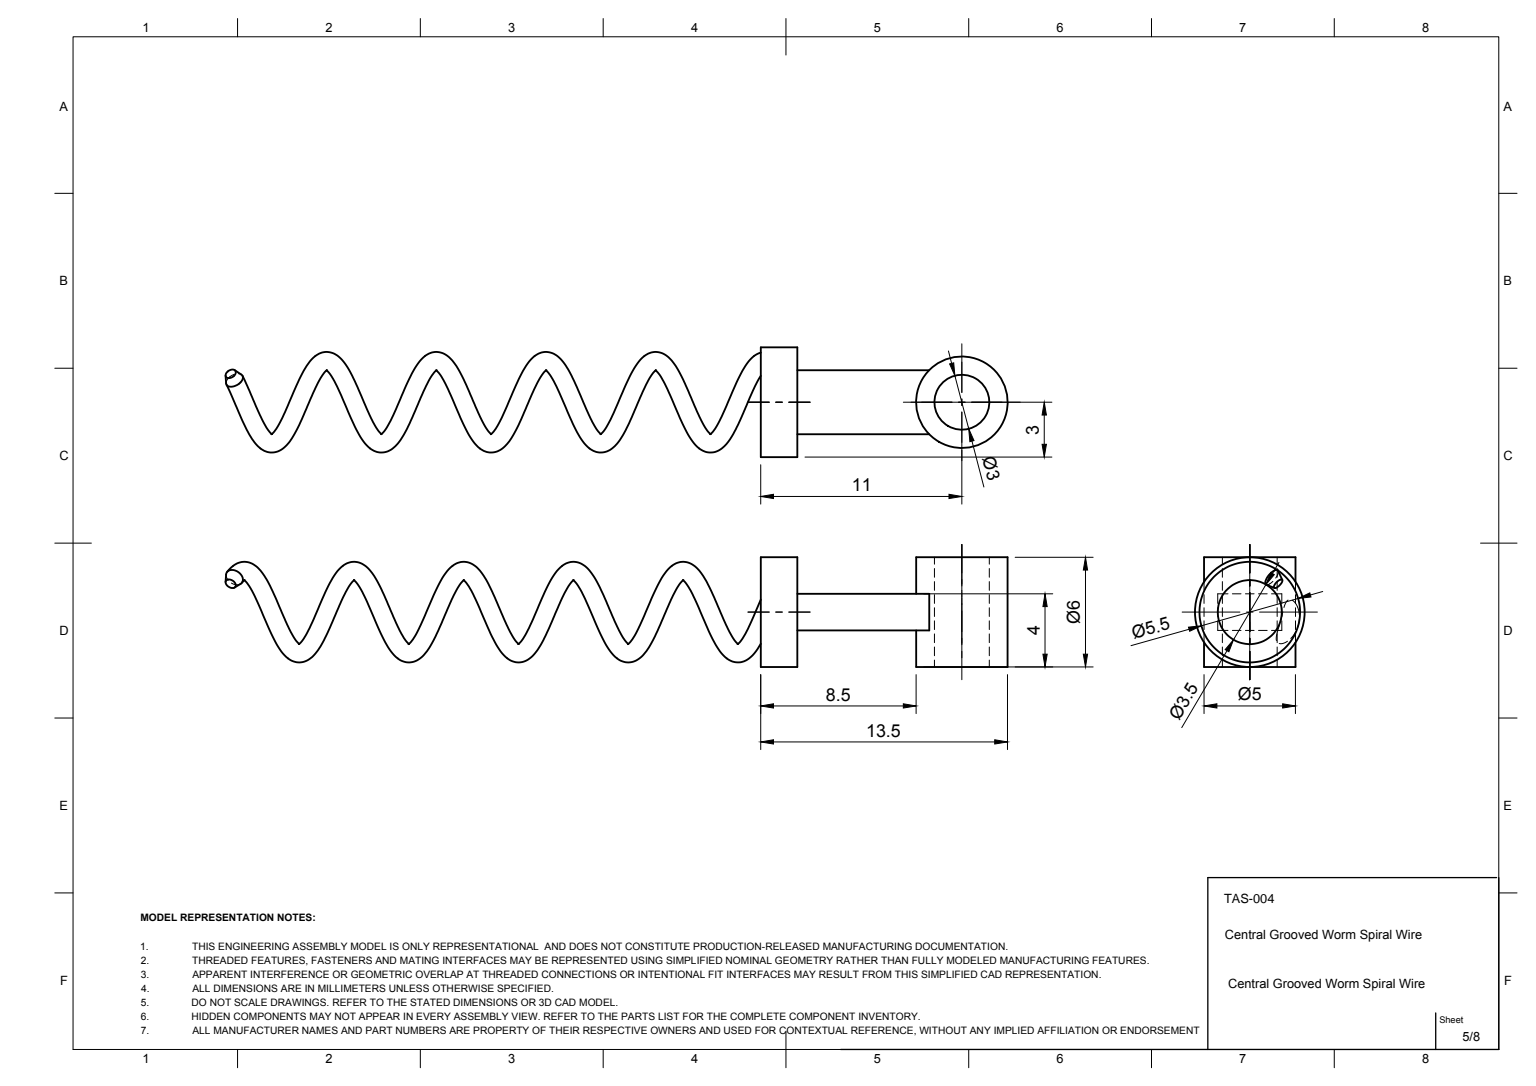
ISO-10303-21;
HEADER;
/* Generated by software containing ST-Developer
 * from STEP Tools, Inc. (www.steptools.com) 
 */

FILE_DESCRIPTION(
/* description */ ('STEP AP214'),
/* implementation_level */ '2;1');

FILE_NAME(
/* name */ 'Central Grooved Worm Spiral Wire.step',
/* time_stamp */ '2026-11-04T19:48:07-08:00',
/* author */ (''),
/* organization */ (''),
/* preprocessor_version */ 'ST-DEVELOPER v20.2',
/* originating_system */ 'Autodesk Translation Framework v15.17.0.0',
/* authorisation */ '');

FILE_SCHEMA (('AUTOMOTIVE_DESIGN { 1 0 10303 214 3 1 1 }'));
ENDSEC;

DATA;
#10=MECHANICAL_DESIGN_GEOMETRIC_PRESENTATION_REPRESENTATION('',(#61),#9561);
#35=(
BOUNDED_SURFACE()
B_SPLINE_SURFACE(3,2,((#4268,#4269,#4270,#4271,#4272,#4273,#4274,#4275,
#4276,#4277,#4278,#4279,#4280,#4281,#4282,#4283,#4284,#4285,#4286,#4287,
#4288,#4289,#4290,#4291,#4292,#4293,#4294,#4295,#4296,#4297,#4298,#4299,
#4300,#4301,#4302,#4303,#4304,#4305,#4306,#4307,#4308,#4309,#4310,#4311,
#4312,#4313,#4314,#4315,#4316,#4317,#4318,#4319,#4320,#4321,#4322,#4323,
#4324,#4325,#4326,#4327,#4328,#4329,#4330,#4331,#4332,#4333,#4334,#4335,
#4336,#4337,#4338,#4339,#4340,#4341,#4342,#4343,#4344,#4345,#4346,#4347,
#4348,#4349,#4350,#4351,#4352,#4353,#4354,#4355,#4356,#4357,#4358,#4359,
#4360,#4361,#4362,#4363,#4364,#4365,#4366,#4367,#4368,#4369,#4370,#4371,
#4372,#4373,#4374,#4375,#4376,#4377,#4378,#4379,#4380,#4381,#4382,#4383,
#4384,#4385,#4386,#4387,#4388,#4389,#4390,#4391,#4392,#4393,#4394,#4395,
#4396,#4397,#4398,#4399,#4400,#4401,#4402,#4403,#4404,#4405,#4406,#4407,
#4408),(#4409,#4410,#4411,#4412,#4413,#4414,#4415,#4416,#4417,#4418,#4419,
#4420,#4421,#4422,#4423,#4424,#4425,#4426,#4427,#4428,#4429,#4430,#4431,
#4432,#4433,#4434,#4435,#4436,#4437,#4438,#4439,#4440,#4441,#4442,#4443,
#4444,#4445,#4446,#4447,#4448,#4449,#4450,#4451,#4452,#4453,#4454,#4455,
#4456,#4457,#4458,#4459,#4460,#4461,#4462,#4463,#4464,#4465,#4466,#4467,
#4468,#4469,#4470,#4471,#4472,#4473,#4474,#4475,#4476,#4477,#4478,#4479,
#4480,#4481,#4482,#4483,#4484,#4485,#4486,#4487,#4488,#4489,#4490,#4491,
#4492,#4493,#4494,#4495,#4496,#4497,#4498,#4499,#4500,#4501,#4502,#4503,
#4504,#4505,#4506,#4507,#4508,#4509,#4510,#4511,#4512,#4513,#4514,#4515,
#4516,#4517,#4518,#4519,#4520,#4521,#4522,#4523,#4524,#4525,#4526,#4527,
#4528,#4529,#4530,#4531,#4532,#4533,#4534,#4535,#4536,#4537,#4538,#4539,
#4540,#4541,#4542,#4543,#4544,#4545,#4546,#4547,#4548,#4549),(#4550,#4551,
#4552,#4553,#4554,#4555,#4556,#4557,#4558,#4559,#4560,#4561,#4562,#4563,
#4564,#4565,#4566,#4567,#4568,#4569,#4570,#4571,#4572,#4573,#4574,#4575,
#4576,#4577,#4578,#4579,#4580,#4581,#4582,#4583,#4584,#4585,#4586,#4587,
#4588,#4589,#4590,#4591,#4592,#4593,#4594,#4595,#4596,#4597,#4598,#4599,
#4600,#4601,#4602,#4603,#4604,#4605,#4606,#4607,#4608,#4609,#4610,#4611,
#4612,#4613,#4614,#4615,#4616,#4617,#4618,#4619,#4620,#4621,#4622,#4623,
#4624,#4625,#4626,#4627,#4628,#4629,#4630,#4631,#4632,#4633,#4634,#4635,
#4636,#4637,#4638,#4639,#4640,#4641,#4642,#4643,#4644,#4645,#4646,#4647,
#4648,#4649,#4650,#4651,#4652,#4653,#4654,#4655,#4656,#4657,#4658,#4659,
#4660,#4661,#4662,#4663,#4664,#4665,#4666,#4667,#4668,#4669,#4670,#4671,
#4672,#4673,#4674,#4675,#4676,#4677,#4678,#4679,#4680,#4681,#4682,#4683,
#4684,#4685,#4686,#4687,#4688,#4689,#4690),(#4691,#4692,#4693,#4694,#4695,
#4696,#4697,#4698,#4699,#4700,#4701,#4702,#4703,#4704,#4705,#4706,#4707,
#4708,#4709,#4710,#4711,#4712,#4713,#4714,#4715,#4716,#4717,#4718,#4719,
#4720,#4721,#4722,#4723,#4724,#4725,#4726,#4727,#4728,#4729,#4730,#4731,
#4732,#4733,#4734,#4735,#4736,#4737,#4738,#4739,#4740,#4741,#4742,#4743,
#4744,#4745,#4746,#4747,#4748,#4749,#4750,#4751,#4752,#4753,#4754,#4755,
#4756,#4757,#4758,#4759,#4760,#4761,#4762,#4763,#4764,#4765,#4766,#4767,
#4768,#4769,#4770,#4771,#4772,#4773,#4774,#4775,#4776,#4777,#4778,#4779,
#4780,#4781,#4782,#4783,#4784,#4785,#4786,#4787,#4788,#4789,#4790,#4791,
#4792,#4793,#4794,#4795,#4796,#4797,#4798,#4799,#4800,#4801,#4802,#4803,
#4804,#4805,#4806,#4807,#4808,#4809,#4810,#4811,#4812,#4813,#4814,#4815,
#4816,#4817,#4818,#4819,#4820,#4821,#4822,#4823,#4824,#4825,#4826,#4827,
#4828,#4829,#4830,#4831),(#4832,#4833,#4834,#4835,#4836,#4837,#4838,#4839,
#4840,#4841,#4842,#4843,#4844,#4845,#4846,#4847,#4848,#4849,#4850,#4851,
#4852,#4853,#4854,#4855,#4856,#4857,#4858,#4859,#4860,#4861,#4862,#4863,
#4864,#4865,#4866,#4867,#4868,#4869,#4870,#4871,#4872,#4873,#4874,#4875,
#4876,#4877,#4878,#4879,#4880,#4881,#4882,#4883,#4884,#4885,#4886,#4887,
#4888,#4889,#4890,#4891,#4892,#4893,#4894,#4895,#4896,#4897,#4898,#4899,
#4900,#4901,#4902,#4903,#4904,#4905,#4906,#4907,#4908,#4909,#4910,#4911,
#4912,#4913,#4914,#4915,#4916,#4917,#4918,#4919,#4920,#4921,#4922,#4923,
#4924,#4925,#4926,#4927,#4928,#4929,#4930,#4931,#4932,#4933,#4934,#4935,
#4936,#4937,#4938,#4939,#4940,#4941,#4942,#4943,#4944,#4945,#4946,#4947,
#4948,#4949,#4950,#4951,#4952,#4953,#4954,#4955,#4956,#4957,#4958,#4959,
#4960,#4961,#4962,#4963,#4964,#4965,#4966,#4967,#4968,#4969,#4970,#4971,
#4972),(#4973,#4974,#4975,#4976,#4977,#4978,#4979,#4980,#4981,#4982,#4983,
#4984,#4985,#4986,#4987,#4988,#4989,#4990,#4991,#4992,#4993,#4994,#4995,
#4996,#4997,#4998,#4999,#5000,#5001,#5002,#5003,#5004,#5005,#5006,#5007,
#5008,#5009,#5010,#5011,#5012,#5013,#5014,#5015,#5016,#5017,#5018,#5019,
#5020,#5021,#5022,#5023,#5024,#5025,#5026,#5027,#5028,#5029,#5030,#5031,
#5032,#5033,#5034,#5035,#5036,#5037,#5038,#5039,#5040,#5041,#5042,#5043,
#5044,#5045,#5046,#5047,#5048,#5049,#5050,#5051,#5052,#5053,#5054,#5055,
#5056,#5057,#5058,#5059,#5060,#5061,#5062,#5063,#5064,#5065,#5066,#5067,
#5068,#5069,#5070,#5071,#5072,#5073,#5074,#5075,#5076,#5077,#5078,#5079,
#5080,#5081,#5082,#5083,#5084,#5085,#5086,#5087,#5088,#5089,#5090,#5091,
#5092,#5093,#5094,#5095,#5096,#5097,#5098,#5099,#5100,#5101,#5102,#5103,
#5104,#5105,#5106,#5107,#5108,#5109,#5110,#5111,#5112,#5113),(#5114,#5115,
#5116,#5117,#5118,#5119,#5120,#5121,#5122,#5123,#5124,#5125,#5126,#5127,
#5128,#5129,#5130,#5131,#5132,#5133,#5134,#5135,#5136,#5137,#5138,#5139,
#5140,#5141,#5142,#5143,#5144,#5145,#5146,#5147,#5148,#5149,#5150,#5151,
#5152,#5153,#5154,#5155,#5156,#5157,#5158,#5159,#5160,#5161,#5162,#5163,
#5164,#5165,#5166,#5167,#5168,#5169,#5170,#5171,#5172,#5173,#5174,#5175,
#5176,#5177,#5178,#5179,#5180,#5181,#5182,#5183,#5184,#5185,#5186,#5187,
#5188,#5189,#5190,#5191,#5192,#5193,#5194,#5195,#5196,#5197,#5198,#5199,
#5200,#5201,#5202,#5203,#5204,#5205,#5206,#5207,#5208,#5209,#5210,#5211,
#5212,#5213,#5214,#5215,#5216,#5217,#5218,#5219,#5220,#5221,#5222,#5223,
#5224,#5225,#5226,#5227,#5228,#5229,#5230,#5231,#5232,#5233,#5234,#5235,
#5236,#5237,#5238,#5239,#5240,#5241,#5242,#5243,#5244,#5245,#5246,#5247,
#5248,#5249,#5250,#5251,#5252,#5253,#5254)),.UNSPECIFIED.,.T.,.F.,.F.)
B_SPLINE_SURFACE_WITH_KNOTS((4,3,4),(3,2,2,2,2,2,2,2,2,2,2,2,2,2,2,2,2,
2,2,2,2,2,2,2,2,2,2,2,2,2,2,2,2,2,2,2,2,2,2,2,2,2,2,2,2,2,2,2,2,2,2,2,2,
2,2,2,2,2,2,2,2,2,2,2,2,2,2,2,2,2,3),(0.,0.5,1.),(0.,0.0142857142857143,
0.0285714285714286,0.0428571428571429,0.0571428571428571,0.0714285714285714,
0.0857142857142857,0.1,0.114285714285714,0.128571428571429,0.142857142857143,
0.157142857142857,0.171428571428571,0.185714285714286,0.2,0.214285714285714,
0.228571428571429,0.242857142857143,0.257142857142857,0.271428571428571,
0.285714285714286,0.3,0.314285714285714,0.328571428571429,0.342857142857143,
0.357142857142857,0.371428571428571,0.385714285714286,0.4,0.414285714285714,
0.428571428571429,0.442857142857143,0.457142857142857,0.471428571428571,
0.485714285714286,0.5,0.514285714285714,0.528571428571429,0.542857142857143,
0.557142857142857,0.571428571428571,0.585714285714286,0.6,0.614285714285714,
0.628571428571429,0.642857142857143,0.657142857142857,0.671428571428571,
0.685714285714286,0.7,0.714285714285714,0.728571428571429,0.742857142857143,
0.757142857142857,0.771428571428571,0.785714285714286,0.8,0.814285714285714,
0.828571428571429,0.842857142857143,0.857142857142857,0.871428571428571,
0.885714285714286,0.9,0.914285714285714,0.928571428571429,0.942857142857143,
0.957142857142857,0.971428571428571,0.985714285714286,1.),.UNSPECIFIED.)
GEOMETRIC_REPRESENTATION_ITEM()
RATIONAL_B_SPLINE_SURFACE(((1.,0.974927912181824,1.,0.974927912181824,1.,
0.974927912181824,1.,0.974927912181824,1.,0.974927912181824,1.,0.974927912181824,
1.,0.974927912181824,1.,0.974927912181824,1.,0.974927912181824,1.,0.974927912181824,
1.,0.974927912181824,1.,0.974927912181824,1.,0.974927912181824,1.,0.974927912181824,
1.,0.974927912181824,1.,0.974927912181824,1.,0.974927912181824,1.,0.974927912181824,
1.,0.974927912181824,1.,0.974927912181824,1.,0.974927912181824,1.,0.974927912181824,
1.,0.974927912181824,1.,0.974927912181824,1.,0.974927912181824,1.,0.974927912181824,
1.,0.974927912181824,1.,0.974927912181824,1.,0.974927912181824,1.,0.974927912181824,
1.,0.974927912181824,1.,0.974927912181824,1.,0.974927912181824,1.,0.974927912181824,
1.,0.974927912181824,1.,0.974927912181824,1.,0.974927912181824,1.,0.974927912181824,
1.,0.974927912181824,1.,0.974927912181824,1.,0.974927912181824,1.,0.974927912181824,
1.,0.974927912181824,1.,0.974927912181824,1.,0.974927912181824,1.,0.974927912181824,
1.,0.974927912181824,1.,0.974927912181824,1.,0.974927912181824,1.,0.974927912181824,
1.,0.974927912181824,1.,0.974927912181824,1.,0.974927912181824,1.,0.974927912181824,
1.,0.974927912181824,1.,0.974927912181824,1.,0.974927912181824,1.,0.974927912181824,
1.,0.974927912181824,1.,0.974927912181824,1.,0.974927912181824,1.,0.974927912181824,
1.,0.974927912181824,1.,0.974927912181824,1.,0.974927912181824,1.,0.974927912181824,
1.,0.974927912181824,1.,0.974927912181824,1.,0.974927912181824,1.,0.974927912181824,
1.),(0.333333333333333,0.324975970727275,0.333333333333333,0.324975970727275,
0.333333333333333,0.324975970727275,0.333333333333333,0.324975970727275,
0.333333333333333,0.324975970727275,0.333333333333333,0.324975970727275,
0.333333333333333,0.324975970727275,0.333333333333333,0.324975970727275,
0.333333333333333,0.324975970727275,0.333333333333333,0.324975970727275,
0.333333333333333,0.324975970727275,0.333333333333333,0.324975970727275,
0.333333333333333,0.324975970727275,0.333333333333333,0.324975970727275,
0.333333333333333,0.324975970727275,0.333333333333333,0.324975970727275,
0.333333333333333,0.324975970727275,0.333333333333333,0.324975970727275,
0.333333333333333,0.324975970727275,0.333333333333333,0.324975970727275,
0.333333333333333,0.324975970727275,0.333333333333333,0.324975970727275,
0.333333333333333,0.324975970727275,0.333333333333333,0.324975970727275,
0.333333333333333,0.324975970727275,0.333333333333333,0.324975970727275,
0.333333333333333,0.324975970727275,0.333333333333333,0.324975970727275,
0.333333333333333,0.324975970727275,0.333333333333333,0.324975970727275,
0.333333333333333,0.324975970727275,0.333333333333333,0.324975970727275,
0.333333333333333,0.324975970727275,0.333333333333333,0.324975970727275,
0.333333333333333,0.324975970727275,0.333333333333333,0.324975970727275,
0.333333333333333,0.324975970727275,0.333333333333333,0.324975970727275,
0.333333333333333,0.324975970727275,0.333333333333333,0.324975970727275,
0.333333333333333,0.324975970727275,0.333333333333333,0.324975970727275,
0.333333333333333,0.324975970727275,0.333333333333333,0.324975970727275,
0.333333333333333,0.324975970727275,0.333333333333333,0.324975970727275,
0.333333333333333,0.324975970727275,0.333333333333333,0.324975970727275,
0.333333333333333,0.324975970727275,0.333333333333333,0.324975970727275,
0.333333333333333,0.324975970727275,0.333333333333333,0.324975970727275,
0.333333333333333,0.324975970727275,0.333333333333333,0.324975970727275,
0.333333333333333,0.324975970727275,0.333333333333333,0.324975970727275,
0.333333333333333,0.324975970727275,0.333333333333333,0.324975970727275,
0.333333333333333,0.324975970727275,0.333333333333333,0.324975970727275,
0.333333333333333,0.324975970727275,0.333333333333333,0.324975970727275,
0.333333333333333,0.324975970727275,0.333333333333333,0.324975970727275,
0.333333333333333,0.324975970727275,0.333333333333333,0.324975970727275,
0.333333333333333,0.324975970727275,0.333333333333333,0.324975970727275,
0.333333333333333,0.324975970727275,0.333333333333333,0.324975970727275,
0.333333333333333),(0.333333333333333,0.324975970727275,0.333333333333333,
0.324975970727275,0.333333333333333,0.324975970727275,0.333333333333333,
0.324975970727275,0.333333333333333,0.324975970727275,0.333333333333333,
0.324975970727275,0.333333333333333,0.324975970727275,0.333333333333333,
0.324975970727275,0.333333333333333,0.324975970727275,0.333333333333333,
0.324975970727275,0.333333333333333,0.324975970727275,0.333333333333333,
0.324975970727275,0.333333333333333,0.324975970727275,0.333333333333333,
0.324975970727275,0.333333333333333,0.324975970727275,0.333333333333333,
0.324975970727275,0.333333333333333,0.324975970727275,0.333333333333333,
0.324975970727275,0.333333333333333,0.324975970727275,0.333333333333333,
0.324975970727275,0.333333333333333,0.324975970727275,0.333333333333333,
0.324975970727275,0.333333333333333,0.324975970727275,0.333333333333333,
0.324975970727275,0.333333333333333,0.324975970727275,0.333333333333333,
0.324975970727275,0.333333333333333,0.324975970727275,0.333333333333333,
0.324975970727275,0.333333333333333,0.324975970727275,0.333333333333333,
0.324975970727275,0.333333333333333,0.324975970727275,0.333333333333333,
0.324975970727275,0.333333333333333,0.324975970727275,0.333333333333333,
0.324975970727275,0.333333333333333,0.324975970727275,0.333333333333333,
0.324975970727275,0.333333333333333,0.324975970727275,0.333333333333333,
0.324975970727275,0.333333333333333,0.324975970727275,0.333333333333333,
0.324975970727275,0.333333333333333,0.324975970727275,0.333333333333333,
0.324975970727275,0.333333333333333,0.324975970727275,0.333333333333333,
0.324975970727275,0.333333333333333,0.324975970727275,0.333333333333333,
0.324975970727275,0.333333333333333,0.324975970727275,0.333333333333333,
0.324975970727275,0.333333333333333,0.324975970727275,0.333333333333333,
0.324975970727275,0.333333333333333,0.324975970727275,0.333333333333333,
0.324975970727275,0.333333333333333,0.324975970727275,0.333333333333333,
0.324975970727275,0.333333333333333,0.324975970727275,0.333333333333333,
0.324975970727275,0.333333333333333,0.324975970727275,0.333333333333333,
0.324975970727275,0.333333333333333,0.324975970727275,0.333333333333333,
0.324975970727275,0.333333333333333,0.324975970727275,0.333333333333333,
0.324975970727275,0.333333333333333,0.324975970727275,0.333333333333333,
0.324975970727275,0.333333333333333,0.324975970727275,0.333333333333333,
0.324975970727275,0.333333333333333,0.324975970727275,0.333333333333333,
0.324975970727275,0.333333333333333,0.324975970727275,0.333333333333333,
0.324975970727275,0.333333333333333),(1.,0.974927912181824,1.,0.974927912181824,
1.,0.974927912181824,1.,0.974927912181824,1.,0.974927912181824,1.,0.974927912181824,
1.,0.974927912181824,1.,0.974927912181824,1.,0.974927912181824,1.,0.974927912181824,
1.,0.974927912181824,1.,0.974927912181824,1.,0.974927912181824,1.,0.974927912181824,
1.,0.974927912181824,1.,0.974927912181824,1.,0.974927912181824,1.,0.974927912181824,
1.,0.974927912181824,1.,0.974927912181824,1.,0.974927912181824,1.,0.974927912181824,
1.,0.974927912181824,1.,0.974927912181824,1.,0.974927912181824,1.,0.974927912181824,
1.,0.974927912181824,1.,0.974927912181824,1.,0.974927912181824,1.,0.974927912181824,
1.,0.974927912181824,1.,0.974927912181824,1.,0.974927912181824,1.,0.974927912181824,
1.,0.974927912181824,1.,0.974927912181824,1.,0.974927912181824,1.,0.974927912181824,
1.,0.974927912181824,1.,0.974927912181824,1.,0.974927912181824,1.,0.974927912181824,
1.,0.974927912181824,1.,0.974927912181824,1.,0.974927912181824,1.,0.974927912181824,
1.,0.974927912181824,1.,0.974927912181824,1.,0.974927912181824,1.,0.974927912181824,
1.,0.974927912181824,1.,0.974927912181824,1.,0.974927912181824,1.,0.974927912181824,
1.,0.974927912181824,1.,0.974927912181824,1.,0.974927912181824,1.,0.974927912181824,
1.,0.974927912181824,1.,0.974927912181824,1.,0.974927912181824,1.,0.974927912181824,
1.,0.974927912181824,1.,0.974927912181824,1.,0.974927912181824,1.,0.974927912181824,
1.,0.974927912181824,1.,0.974927912181824,1.,0.974927912181824,1.,0.974927912181824,
1.),(0.333333333333333,0.324975970727275,0.333333333333333,0.324975970727275,
0.333333333333333,0.324975970727275,0.333333333333333,0.324975970727275,
0.333333333333333,0.324975970727275,0.333333333333333,0.324975970727275,
0.333333333333333,0.324975970727275,0.333333333333333,0.324975970727275,
0.333333333333333,0.324975970727275,0.333333333333333,0.324975970727275,
0.333333333333333,0.324975970727275,0.333333333333333,0.324975970727275,
0.333333333333333,0.324975970727275,0.333333333333333,0.324975970727275,
0.333333333333333,0.324975970727275,0.333333333333333,0.324975970727275,
0.333333333333333,0.324975970727275,0.333333333333333,0.324975970727275,
0.333333333333333,0.324975970727275,0.333333333333333,0.324975970727275,
0.333333333333333,0.324975970727275,0.333333333333333,0.324975970727275,
0.333333333333333,0.324975970727275,0.333333333333333,0.324975970727275,
0.333333333333333,0.324975970727275,0.333333333333333,0.324975970727275,
0.333333333333333,0.324975970727275,0.333333333333333,0.324975970727275,
0.333333333333333,0.324975970727275,0.333333333333333,0.324975970727275,
0.333333333333333,0.324975970727275,0.333333333333333,0.324975970727275,
0.333333333333333,0.324975970727275,0.333333333333333,0.324975970727275,
0.333333333333333,0.324975970727275,0.333333333333333,0.324975970727275,
0.333333333333333,0.324975970727275,0.333333333333333,0.324975970727275,
0.333333333333333,0.324975970727275,0.333333333333333,0.324975970727275,
0.333333333333333,0.324975970727275,0.333333333333333,0.324975970727275,
0.333333333333333,0.324975970727275,0.333333333333333,0.324975970727275,
0.333333333333333,0.324975970727275,0.333333333333333,0.324975970727275,
0.333333333333333,0.324975970727275,0.333333333333333,0.324975970727275,
0.333333333333333,0.324975970727275,0.333333333333333,0.324975970727275,
0.333333333333333,0.324975970727275,0.333333333333333,0.324975970727275,
0.333333333333333,0.324975970727275,0.333333333333333,0.324975970727275,
0.333333333333333,0.324975970727275,0.333333333333333,0.324975970727275,
0.333333333333333,0.324975970727275,0.333333333333333,0.324975970727275,
0.333333333333333,0.324975970727275,0.333333333333333,0.324975970727275,
0.333333333333333,0.324975970727275,0.333333333333333,0.324975970727275,
0.333333333333333,0.324975970727275,0.333333333333333,0.324975970727275,
0.333333333333333,0.324975970727275,0.333333333333333,0.324975970727275,
0.333333333333333,0.324975970727275,0.333333333333333,0.324975970727275,
0.333333333333333,0.324975970727275,0.333333333333333,0.324975970727275,
0.333333333333333),(0.333333333333333,0.324975970727275,0.333333333333333,
0.324975970727275,0.333333333333333,0.324975970727275,0.333333333333333,
0.324975970727275,0.333333333333333,0.324975970727275,0.333333333333333,
0.324975970727275,0.333333333333333,0.324975970727275,0.333333333333333,
0.324975970727275,0.333333333333333,0.324975970727275,0.333333333333333,
0.324975970727275,0.333333333333333,0.324975970727275,0.333333333333333,
0.324975970727275,0.333333333333333,0.324975970727275,0.333333333333333,
0.324975970727275,0.333333333333333,0.324975970727275,0.333333333333333,
0.324975970727275,0.333333333333333,0.324975970727275,0.333333333333333,
0.324975970727275,0.333333333333333,0.324975970727275,0.333333333333333,
0.324975970727275,0.333333333333333,0.324975970727275,0.333333333333333,
0.324975970727275,0.333333333333333,0.324975970727275,0.333333333333333,
0.324975970727275,0.333333333333333,0.324975970727275,0.333333333333333,
0.324975970727275,0.333333333333333,0.324975970727275,0.333333333333333,
0.324975970727275,0.333333333333333,0.324975970727275,0.333333333333333,
0.324975970727275,0.333333333333333,0.324975970727275,0.333333333333333,
0.324975970727275,0.333333333333333,0.324975970727275,0.333333333333333,
0.324975970727275,0.333333333333333,0.324975970727275,0.333333333333333,
0.324975970727275,0.333333333333333,0.324975970727275,0.333333333333333,
0.324975970727275,0.333333333333333,0.324975970727275,0.333333333333333,
0.324975970727275,0.333333333333333,0.324975970727275,0.333333333333333,
0.324975970727275,0.333333333333333,0.324975970727275,0.333333333333333,
0.324975970727275,0.333333333333333,0.324975970727275,0.333333333333333,
0.324975970727275,0.333333333333333,0.324975970727275,0.333333333333333,
0.324975970727275,0.333333333333333,0.324975970727275,0.333333333333333,
0.324975970727275,0.333333333333333,0.324975970727275,0.333333333333333,
0.324975970727275,0.333333333333333,0.324975970727275,0.333333333333333,
0.324975970727275,0.333333333333333,0.324975970727275,0.333333333333333,
0.324975970727275,0.333333333333333,0.324975970727275,0.333333333333333,
0.324975970727275,0.333333333333333,0.324975970727275,0.333333333333333,
0.324975970727275,0.333333333333333,0.324975970727275,0.333333333333333,
0.324975970727275,0.333333333333333,0.324975970727275,0.333333333333333,
0.324975970727275,0.333333333333333,0.324975970727275,0.333333333333333,
0.324975970727275,0.333333333333333,0.324975970727275,0.333333333333333,
0.324975970727275,0.333333333333333,0.324975970727275,0.333333333333333,
0.324975970727275,0.333333333333333),(1.,0.974927912181824,1.,0.974927912181824,
1.,0.974927912181824,1.,0.974927912181824,1.,0.974927912181824,1.,0.974927912181824,
1.,0.974927912181824,1.,0.974927912181824,1.,0.974927912181824,1.,0.974927912181824,
1.,0.974927912181824,1.,0.974927912181824,1.,0.974927912181824,1.,0.974927912181824,
1.,0.974927912181824,1.,0.974927912181824,1.,0.974927912181824,1.,0.974927912181824,
1.,0.974927912181824,1.,0.974927912181824,1.,0.974927912181824,1.,0.974927912181824,
1.,0.974927912181824,1.,0.974927912181824,1.,0.974927912181824,1.,0.974927912181824,
1.,0.974927912181824,1.,0.974927912181824,1.,0.974927912181824,1.,0.974927912181824,
1.,0.974927912181824,1.,0.974927912181824,1.,0.974927912181824,1.,0.974927912181824,
1.,0.974927912181824,1.,0.974927912181824,1.,0.974927912181824,1.,0.974927912181824,
1.,0.974927912181824,1.,0.974927912181824,1.,0.974927912181824,1.,0.974927912181824,
1.,0.974927912181824,1.,0.974927912181824,1.,0.974927912181824,1.,0.974927912181824,
1.,0.974927912181824,1.,0.974927912181824,1.,0.974927912181824,1.,0.974927912181824,
1.,0.974927912181824,1.,0.974927912181824,1.,0.974927912181824,1.,0.974927912181824,
1.,0.974927912181824,1.,0.974927912181824,1.,0.974927912181824,1.,0.974927912181824,
1.,0.974927912181824,1.,0.974927912181824,1.,0.974927912181824,1.,0.974927912181824,
1.,0.974927912181824,1.,0.974927912181824,1.,0.974927912181824,1.,0.974927912181824,
1.,0.974927912181824,1.,0.974927912181824,1.,0.974927912181824,1.,0.974927912181824,
1.)))
REPRESENTATION_ITEM('')
SURFACE()
);
#36=(
BOUNDED_SURFACE()
B_SPLINE_SURFACE(3,2,((#8296,#8297,#8298,#8299,#8300,#8301,#8302,#8303,
#8304,#8305,#8306,#8307,#8308,#8309,#8310,#8311,#8312,#8313,#8314,#8315,
#8316,#8317,#8318,#8319,#8320,#8321,#8322,#8323,#8324,#8325,#8326,#8327,
#8328,#8329,#8330,#8331,#8332,#8333,#8334,#8335,#8336,#8337,#8338,#8339,
#8340,#8341,#8342,#8343,#8344,#8345,#8346,#8347,#8348,#8349,#8350,#8351,
#8352,#8353,#8354,#8355,#8356,#8357,#8358,#8359,#8360,#8361,#8362,#8363,
#8364,#8365,#8366,#8367,#8368,#8369,#8370,#8371,#8372,#8373,#8374,#8375,
#8376,#8377,#8378,#8379,#8380,#8381,#8382,#8383,#8384,#8385,#8386,#8387,
#8388,#8389,#8390,#8391,#8392,#8393,#8394,#8395,#8396,#8397,#8398,#8399,
#8400,#8401,#8402,#8403,#8404,#8405,#8406,#8407,#8408,#8409,#8410,#8411,
#8412,#8413,#8414,#8415,#8416,#8417,#8418,#8419,#8420,#8421,#8422,#8423,
#8424,#8425,#8426,#8427,#8428,#8429,#8430,#8431,#8432,#8433,#8434,#8435,
#8436),(#8437,#8438,#8439,#8440,#8441,#8442,#8443,#8444,#8445,#8446,#8447,
#8448,#8449,#8450,#8451,#8452,#8453,#8454,#8455,#8456,#8457,#8458,#8459,
#8460,#8461,#8462,#8463,#8464,#8465,#8466,#8467,#8468,#8469,#8470,#8471,
#8472,#8473,#8474,#8475,#8476,#8477,#8478,#8479,#8480,#8481,#8482,#8483,
#8484,#8485,#8486,#8487,#8488,#8489,#8490,#8491,#8492,#8493,#8494,#8495,
#8496,#8497,#8498,#8499,#8500,#8501,#8502,#8503,#8504,#8505,#8506,#8507,
#8508,#8509,#8510,#8511,#8512,#8513,#8514,#8515,#8516,#8517,#8518,#8519,
#8520,#8521,#8522,#8523,#8524,#8525,#8526,#8527,#8528,#8529,#8530,#8531,
#8532,#8533,#8534,#8535,#8536,#8537,#8538,#8539,#8540,#8541,#8542,#8543,
#8544,#8545,#8546,#8547,#8548,#8549,#8550,#8551,#8552,#8553,#8554,#8555,
#8556,#8557,#8558,#8559,#8560,#8561,#8562,#8563,#8564,#8565,#8566,#8567,
#8568,#8569,#8570,#8571,#8572,#8573,#8574,#8575,#8576,#8577),(#8578,#8579,
#8580,#8581,#8582,#8583,#8584,#8585,#8586,#8587,#8588,#8589,#8590,#8591,
#8592,#8593,#8594,#8595,#8596,#8597,#8598,#8599,#8600,#8601,#8602,#8603,
#8604,#8605,#8606,#8607,#8608,#8609,#8610,#8611,#8612,#8613,#8614,#8615,
#8616,#8617,#8618,#8619,#8620,#8621,#8622,#8623,#8624,#8625,#8626,#8627,
#8628,#8629,#8630,#8631,#8632,#8633,#8634,#8635,#8636,#8637,#8638,#8639,
#8640,#8641,#8642,#8643,#8644,#8645,#8646,#8647,#8648,#8649,#8650,#8651,
#8652,#8653,#8654,#8655,#8656,#8657,#8658,#8659,#8660,#8661,#8662,#8663,
#8664,#8665,#8666,#8667,#8668,#8669,#8670,#8671,#8672,#8673,#8674,#8675,
#8676,#8677,#8678,#8679,#8680,#8681,#8682,#8683,#8684,#8685,#8686,#8687,
#8688,#8689,#8690,#8691,#8692,#8693,#8694,#8695,#8696,#8697,#8698,#8699,
#8700,#8701,#8702,#8703,#8704,#8705,#8706,#8707,#8708,#8709,#8710,#8711,
#8712,#8713,#8714,#8715,#8716,#8717,#8718),(#8719,#8720,#8721,#8722,#8723,
#8724,#8725,#8726,#8727,#8728,#8729,#8730,#8731,#8732,#8733,#8734,#8735,
#8736,#8737,#8738,#8739,#8740,#8741,#8742,#8743,#8744,#8745,#8746,#8747,
#8748,#8749,#8750,#8751,#8752,#8753,#8754,#8755,#8756,#8757,#8758,#8759,
#8760,#8761,#8762,#8763,#8764,#8765,#8766,#8767,#8768,#8769,#8770,#8771,
#8772,#8773,#8774,#8775,#8776,#8777,#8778,#8779,#8780,#8781,#8782,#8783,
#8784,#8785,#8786,#8787,#8788,#8789,#8790,#8791,#8792,#8793,#8794,#8795,
#8796,#8797,#8798,#8799,#8800,#8801,#8802,#8803,#8804,#8805,#8806,#8807,
#8808,#8809,#8810,#8811,#8812,#8813,#8814,#8815,#8816,#8817,#8818,#8819,
#8820,#8821,#8822,#8823,#8824,#8825,#8826,#8827,#8828,#8829,#8830,#8831,
#8832,#8833,#8834,#8835,#8836,#8837,#8838,#8839,#8840,#8841,#8842,#8843,
#8844,#8845,#8846,#8847,#8848,#8849,#8850,#8851,#8852,#8853,#8854,#8855,
#8856,#8857,#8858,#8859),(#8860,#8861,#8862,#8863,#8864,#8865,#8866,#8867,
#8868,#8869,#8870,#8871,#8872,#8873,#8874,#8875,#8876,#8877,#8878,#8879,
#8880,#8881,#8882,#8883,#8884,#8885,#8886,#8887,#8888,#8889,#8890,#8891,
#8892,#8893,#8894,#8895,#8896,#8897,#8898,#8899,#8900,#8901,#8902,#8903,
#8904,#8905,#8906,#8907,#8908,#8909,#8910,#8911,#8912,#8913,#8914,#8915,
#8916,#8917,#8918,#8919,#8920,#8921,#8922,#8923,#8924,#8925,#8926,#8927,
#8928,#8929,#8930,#8931,#8932,#8933,#8934,#8935,#8936,#8937,#8938,#8939,
#8940,#8941,#8942,#8943,#8944,#8945,#8946,#8947,#8948,#8949,#8950,#8951,
#8952,#8953,#8954,#8955,#8956,#8957,#8958,#8959,#8960,#8961,#8962,#8963,
#8964,#8965,#8966,#8967,#8968,#8969,#8970,#8971,#8972,#8973,#8974,#8975,
#8976,#8977,#8978,#8979,#8980,#8981,#8982,#8983,#8984,#8985,#8986,#8987,
#8988,#8989,#8990,#8991,#8992,#8993,#8994,#8995,#8996,#8997,#8998,#8999,
#9000),(#9001,#9002,#9003,#9004,#9005,#9006,#9007,#9008,#9009,#9010,#9011,
#9012,#9013,#9014,#9015,#9016,#9017,#9018,#9019,#9020,#9021,#9022,#9023,
#9024,#9025,#9026,#9027,#9028,#9029,#9030,#9031,#9032,#9033,#9034,#9035,
#9036,#9037,#9038,#9039,#9040,#9041,#9042,#9043,#9044,#9045,#9046,#9047,
#9048,#9049,#9050,#9051,#9052,#9053,#9054,#9055,#9056,#9057,#9058,#9059,
#9060,#9061,#9062,#9063,#9064,#9065,#9066,#9067,#9068,#9069,#9070,#9071,
#9072,#9073,#9074,#9075,#9076,#9077,#9078,#9079,#9080,#9081,#9082,#9083,
#9084,#9085,#9086,#9087,#9088,#9089,#9090,#9091,#9092,#9093,#9094,#9095,
#9096,#9097,#9098,#9099,#9100,#9101,#9102,#9103,#9104,#9105,#9106,#9107,
#9108,#9109,#9110,#9111,#9112,#9113,#9114,#9115,#9116,#9117,#9118,#9119,
#9120,#9121,#9122,#9123,#9124,#9125,#9126,#9127,#9128,#9129,#9130,#9131,
#9132,#9133,#9134,#9135,#9136,#9137,#9138,#9139,#9140,#9141),(#9142,#9143,
#9144,#9145,#9146,#9147,#9148,#9149,#9150,#9151,#9152,#9153,#9154,#9155,
#9156,#9157,#9158,#9159,#9160,#9161,#9162,#9163,#9164,#9165,#9166,#9167,
#9168,#9169,#9170,#9171,#9172,#9173,#9174,#9175,#9176,#9177,#9178,#9179,
#9180,#9181,#9182,#9183,#9184,#9185,#9186,#9187,#9188,#9189,#9190,#9191,
#9192,#9193,#9194,#9195,#9196,#9197,#9198,#9199,#9200,#9201,#9202,#9203,
#9204,#9205,#9206,#9207,#9208,#9209,#9210,#9211,#9212,#9213,#9214,#9215,
#9216,#9217,#9218,#9219,#9220,#9221,#9222,#9223,#9224,#9225,#9226,#9227,
#9228,#9229,#9230,#9231,#9232,#9233,#9234,#9235,#9236,#9237,#9238,#9239,
#9240,#9241,#9242,#9243,#9244,#9245,#9246,#9247,#9248,#9249,#9250,#9251,
#9252,#9253,#9254,#9255,#9256,#9257,#9258,#9259,#9260,#9261,#9262,#9263,
#9264,#9265,#9266,#9267,#9268,#9269,#9270,#9271,#9272,#9273,#9274,#9275,
#9276,#9277,#9278,#9279,#9280,#9281,#9282)),.UNSPECIFIED.,.T.,.F.,.F.)
B_SPLINE_SURFACE_WITH_KNOTS((4,3,4),(3,2,2,2,2,2,2,2,2,2,2,2,2,2,2,2,2,
2,2,2,2,2,2,2,2,2,2,2,2,2,2,2,2,2,2,2,2,2,2,2,2,2,2,2,2,2,2,2,2,2,2,2,2,
2,2,2,2,2,2,2,2,2,2,2,2,2,2,2,2,2,3),(0.,0.5,1.),(0.,0.0142857142857143,
0.0285714285714286,0.0428571428571429,0.0571428571428571,0.0714285714285714,
0.0857142857142857,0.1,0.114285714285714,0.128571428571429,0.142857142857143,
0.157142857142857,0.171428571428571,0.185714285714286,0.2,0.214285714285714,
0.228571428571429,0.242857142857143,0.257142857142857,0.271428571428571,
0.285714285714286,0.3,0.314285714285714,0.328571428571429,0.342857142857143,
0.357142857142857,0.371428571428571,0.385714285714286,0.4,0.414285714285714,
0.428571428571429,0.442857142857143,0.457142857142857,0.471428571428571,
0.485714285714286,0.5,0.514285714285714,0.528571428571429,0.542857142857143,
0.557142857142857,0.571428571428571,0.585714285714286,0.6,0.614285714285714,
0.628571428571429,0.642857142857143,0.657142857142857,0.671428571428571,
0.685714285714286,0.7,0.714285714285714,0.728571428571429,0.742857142857143,
0.757142857142857,0.771428571428571,0.785714285714286,0.8,0.814285714285714,
0.828571428571429,0.842857142857143,0.857142857142857,0.871428571428571,
0.885714285714286,0.9,0.914285714285714,0.928571428571429,0.942857142857143,
0.957142857142857,0.971428571428571,0.985714285714286,1.),.UNSPECIFIED.)
GEOMETRIC_REPRESENTATION_ITEM()
RATIONAL_B_SPLINE_SURFACE(((1.,0.974927912181824,1.,0.974927912181824,1.,
0.974927912181824,1.,0.974927912181824,1.,0.974927912181824,1.,0.974927912181824,
1.,0.974927912181824,1.,0.974927912181824,1.,0.974927912181824,1.,0.974927912181824,
1.,0.974927912181824,1.,0.974927912181824,1.,0.974927912181824,1.,0.974927912181824,
1.,0.974927912181824,1.,0.974927912181824,1.,0.974927912181824,1.,0.974927912181824,
1.,0.974927912181824,1.,0.974927912181824,1.,0.974927912181824,1.,0.974927912181824,
1.,0.974927912181824,1.,0.974927912181824,1.,0.974927912181824,1.,0.974927912181824,
1.,0.974927912181824,1.,0.974927912181824,1.,0.974927912181824,1.,0.974927912181824,
1.,0.974927912181824,1.,0.974927912181824,1.,0.974927912181824,1.,0.974927912181824,
1.,0.974927912181824,1.,0.974927912181824,1.,0.974927912181824,1.,0.974927912181824,
1.,0.974927912181824,1.,0.974927912181824,1.,0.974927912181824,1.,0.974927912181824,
1.,0.974927912181824,1.,0.974927912181824,1.,0.974927912181824,1.,0.974927912181824,
1.,0.974927912181824,1.,0.974927912181824,1.,0.974927912181824,1.,0.974927912181824,
1.,0.974927912181824,1.,0.974927912181824,1.,0.974927912181824,1.,0.974927912181824,
1.,0.974927912181824,1.,0.974927912181824,1.,0.974927912181824,1.,0.974927912181824,
1.,0.974927912181824,1.,0.974927912181824,1.,0.974927912181824,1.,0.974927912181824,
1.,0.974927912181824,1.,0.974927912181824,1.,0.974927912181824,1.,0.974927912181824,
1.,0.974927912181824,1.,0.974927912181824,1.,0.974927912181824,1.,0.974927912181824,
1.),(0.333333333333333,0.324975970727275,0.333333333333333,0.324975970727275,
0.333333333333333,0.324975970727275,0.333333333333333,0.324975970727275,
0.333333333333333,0.324975970727275,0.333333333333333,0.324975970727275,
0.333333333333333,0.324975970727275,0.333333333333333,0.324975970727275,
0.333333333333333,0.324975970727275,0.333333333333333,0.324975970727275,
0.333333333333333,0.324975970727275,0.333333333333333,0.324975970727275,
0.333333333333333,0.324975970727275,0.333333333333333,0.324975970727275,
0.333333333333333,0.324975970727275,0.333333333333333,0.324975970727275,
0.333333333333333,0.324975970727275,0.333333333333333,0.324975970727275,
0.333333333333333,0.324975970727275,0.333333333333333,0.324975970727275,
0.333333333333333,0.324975970727275,0.333333333333333,0.324975970727275,
0.333333333333333,0.324975970727275,0.333333333333333,0.324975970727275,
0.333333333333333,0.324975970727275,0.333333333333333,0.324975970727275,
0.333333333333333,0.324975970727275,0.333333333333333,0.324975970727275,
0.333333333333333,0.324975970727275,0.333333333333333,0.324975970727275,
0.333333333333333,0.324975970727275,0.333333333333333,0.324975970727275,
0.333333333333333,0.324975970727275,0.333333333333333,0.324975970727275,
0.333333333333333,0.324975970727275,0.333333333333333,0.324975970727275,
0.333333333333333,0.324975970727275,0.333333333333333,0.324975970727275,
0.333333333333333,0.324975970727275,0.333333333333333,0.324975970727275,
0.333333333333333,0.324975970727275,0.333333333333333,0.324975970727275,
0.333333333333333,0.324975970727275,0.333333333333333,0.324975970727275,
0.333333333333333,0.324975970727275,0.333333333333333,0.324975970727275,
0.333333333333333,0.324975970727275,0.333333333333333,0.324975970727275,
0.333333333333333,0.324975970727275,0.333333333333333,0.324975970727275,
0.333333333333333,0.324975970727275,0.333333333333333,0.324975970727275,
0.333333333333333,0.324975970727275,0.333333333333333,0.324975970727275,
0.333333333333333,0.324975970727275,0.333333333333333,0.324975970727275,
0.333333333333333,0.324975970727275,0.333333333333333,0.324975970727275,
0.333333333333333,0.324975970727275,0.333333333333333,0.324975970727275,
0.333333333333333,0.324975970727275,0.333333333333333,0.324975970727275,
0.333333333333333,0.324975970727275,0.333333333333333,0.324975970727275,
0.333333333333333,0.324975970727275,0.333333333333333,0.324975970727275,
0.333333333333333,0.324975970727275,0.333333333333333,0.324975970727275,
0.333333333333333,0.324975970727275,0.333333333333333,0.324975970727275,
0.333333333333333),(0.333333333333333,0.324975970727275,0.333333333333333,
0.324975970727275,0.333333333333333,0.324975970727275,0.333333333333333,
0.324975970727275,0.333333333333333,0.324975970727275,0.333333333333333,
0.324975970727275,0.333333333333333,0.324975970727275,0.333333333333333,
0.324975970727275,0.333333333333333,0.324975970727275,0.333333333333333,
0.324975970727275,0.333333333333333,0.324975970727275,0.333333333333333,
0.324975970727275,0.333333333333333,0.324975970727275,0.333333333333333,
0.324975970727275,0.333333333333333,0.324975970727275,0.333333333333333,
0.324975970727275,0.333333333333333,0.324975970727275,0.333333333333333,
0.324975970727275,0.333333333333333,0.324975970727275,0.333333333333333,
0.324975970727275,0.333333333333333,0.324975970727275,0.333333333333333,
0.324975970727275,0.333333333333333,0.324975970727275,0.333333333333333,
0.324975970727275,0.333333333333333,0.324975970727275,0.333333333333333,
0.324975970727275,0.333333333333333,0.324975970727275,0.333333333333333,
0.324975970727275,0.333333333333333,0.324975970727275,0.333333333333333,
0.324975970727275,0.333333333333333,0.324975970727275,0.333333333333333,
0.324975970727275,0.333333333333333,0.324975970727275,0.333333333333333,
0.324975970727275,0.333333333333333,0.324975970727275,0.333333333333333,
0.324975970727275,0.333333333333333,0.324975970727275,0.333333333333333,
0.324975970727275,0.333333333333333,0.324975970727275,0.333333333333333,
0.324975970727275,0.333333333333333,0.324975970727275,0.333333333333333,
0.324975970727275,0.333333333333333,0.324975970727275,0.333333333333333,
0.324975970727275,0.333333333333333,0.324975970727275,0.333333333333333,
0.324975970727275,0.333333333333333,0.324975970727275,0.333333333333333,
0.324975970727275,0.333333333333333,0.324975970727275,0.333333333333333,
0.324975970727275,0.333333333333333,0.324975970727275,0.333333333333333,
0.324975970727275,0.333333333333333,0.324975970727275,0.333333333333333,
0.324975970727275,0.333333333333333,0.324975970727275,0.333333333333333,
0.324975970727275,0.333333333333333,0.324975970727275,0.333333333333333,
0.324975970727275,0.333333333333333,0.324975970727275,0.333333333333333,
0.324975970727275,0.333333333333333,0.324975970727275,0.333333333333333,
0.324975970727275,0.333333333333333,0.324975970727275,0.333333333333333,
0.324975970727275,0.333333333333333,0.324975970727275,0.333333333333333,
0.324975970727275,0.333333333333333,0.324975970727275,0.333333333333333,
0.324975970727275,0.333333333333333,0.324975970727275,0.333333333333333,
0.324975970727275,0.333333333333333),(1.,0.974927912181824,1.,0.974927912181824,
1.,0.974927912181824,1.,0.974927912181824,1.,0.974927912181824,1.,0.974927912181824,
1.,0.974927912181824,1.,0.974927912181824,1.,0.974927912181824,1.,0.974927912181824,
1.,0.974927912181824,1.,0.974927912181824,1.,0.974927912181824,1.,0.974927912181824,
1.,0.974927912181824,1.,0.974927912181824,1.,0.974927912181824,1.,0.974927912181824,
1.,0.974927912181824,1.,0.974927912181824,1.,0.974927912181824,1.,0.974927912181824,
1.,0.974927912181824,1.,0.974927912181824,1.,0.974927912181824,1.,0.974927912181824,
1.,0.974927912181824,1.,0.974927912181824,1.,0.974927912181824,1.,0.974927912181824,
1.,0.974927912181824,1.,0.974927912181824,1.,0.974927912181824,1.,0.974927912181824,
1.,0.974927912181824,1.,0.974927912181824,1.,0.974927912181824,1.,0.974927912181824,
1.,0.974927912181824,1.,0.974927912181824,1.,0.974927912181824,1.,0.974927912181824,
1.,0.974927912181824,1.,0.974927912181824,1.,0.974927912181824,1.,0.974927912181824,
1.,0.974927912181824,1.,0.974927912181824,1.,0.974927912181824,1.,0.974927912181824,
1.,0.974927912181824,1.,0.974927912181824,1.,0.974927912181824,1.,0.974927912181824,
1.,0.974927912181824,1.,0.974927912181824,1.,0.974927912181824,1.,0.974927912181824,
1.,0.974927912181824,1.,0.974927912181824,1.,0.974927912181824,1.,0.974927912181824,
1.,0.974927912181824,1.,0.974927912181824,1.,0.974927912181824,1.,0.974927912181824,
1.,0.974927912181824,1.,0.974927912181824,1.,0.974927912181824,1.,0.974927912181824,
1.),(0.333333333333333,0.324975970727275,0.333333333333333,0.324975970727275,
0.333333333333333,0.324975970727275,0.333333333333333,0.324975970727275,
0.333333333333333,0.324975970727275,0.333333333333333,0.324975970727275,
0.333333333333333,0.324975970727275,0.333333333333333,0.324975970727275,
0.333333333333333,0.324975970727275,0.333333333333333,0.324975970727275,
0.333333333333333,0.324975970727275,0.333333333333333,0.324975970727275,
0.333333333333333,0.324975970727275,0.333333333333333,0.324975970727275,
0.333333333333333,0.324975970727275,0.333333333333333,0.324975970727275,
0.333333333333333,0.324975970727275,0.333333333333333,0.324975970727275,
0.333333333333333,0.324975970727275,0.333333333333333,0.324975970727275,
0.333333333333333,0.324975970727275,0.333333333333333,0.324975970727275,
0.333333333333333,0.324975970727275,0.333333333333333,0.324975970727275,
0.333333333333333,0.324975970727275,0.333333333333333,0.324975970727275,
0.333333333333333,0.324975970727275,0.333333333333333,0.324975970727275,
0.333333333333333,0.324975970727275,0.333333333333333,0.324975970727275,
0.333333333333333,0.324975970727275,0.333333333333333,0.324975970727275,
0.333333333333333,0.324975970727275,0.333333333333333,0.324975970727275,
0.333333333333333,0.324975970727275,0.333333333333333,0.324975970727275,
0.333333333333333,0.324975970727275,0.333333333333333,0.324975970727275,
0.333333333333333,0.324975970727275,0.333333333333333,0.324975970727275,
0.333333333333333,0.324975970727275,0.333333333333333,0.324975970727275,
0.333333333333333,0.324975970727275,0.333333333333333,0.324975970727275,
0.333333333333333,0.324975970727275,0.333333333333333,0.324975970727275,
0.333333333333333,0.324975970727275,0.333333333333333,0.324975970727275,
0.333333333333333,0.324975970727275,0.333333333333333,0.324975970727275,
0.333333333333333,0.324975970727275,0.333333333333333,0.324975970727275,
0.333333333333333,0.324975970727275,0.333333333333333,0.324975970727275,
0.333333333333333,0.324975970727275,0.333333333333333,0.324975970727275,
0.333333333333333,0.324975970727275,0.333333333333333,0.324975970727275,
0.333333333333333,0.324975970727275,0.333333333333333,0.324975970727275,
0.333333333333333,0.324975970727275,0.333333333333333,0.324975970727275,
0.333333333333333,0.324975970727275,0.333333333333333,0.324975970727275,
0.333333333333333,0.324975970727275,0.333333333333333,0.324975970727275,
0.333333333333333,0.324975970727275,0.333333333333333,0.324975970727275,
0.333333333333333,0.324975970727275,0.333333333333333,0.324975970727275,
0.333333333333333),(0.333333333333333,0.324975970727275,0.333333333333333,
0.324975970727275,0.333333333333333,0.324975970727275,0.333333333333333,
0.324975970727275,0.333333333333333,0.324975970727275,0.333333333333333,
0.324975970727275,0.333333333333333,0.324975970727275,0.333333333333333,
0.324975970727275,0.333333333333333,0.324975970727275,0.333333333333333,
0.324975970727275,0.333333333333333,0.324975970727275,0.333333333333333,
0.324975970727275,0.333333333333333,0.324975970727275,0.333333333333333,
0.324975970727275,0.333333333333333,0.324975970727275,0.333333333333333,
0.324975970727275,0.333333333333333,0.324975970727275,0.333333333333333,
0.324975970727275,0.333333333333333,0.324975970727275,0.333333333333333,
0.324975970727275,0.333333333333333,0.324975970727275,0.333333333333333,
0.324975970727275,0.333333333333333,0.324975970727275,0.333333333333333,
0.324975970727275,0.333333333333333,0.324975970727275,0.333333333333333,
0.324975970727275,0.333333333333333,0.324975970727275,0.333333333333333,
0.324975970727275,0.333333333333333,0.324975970727275,0.333333333333333,
0.324975970727275,0.333333333333333,0.324975970727275,0.333333333333333,
0.324975970727275,0.333333333333333,0.324975970727275,0.333333333333333,
0.324975970727275,0.333333333333333,0.324975970727275,0.333333333333333,
0.324975970727275,0.333333333333333,0.324975970727275,0.333333333333333,
0.324975970727275,0.333333333333333,0.324975970727275,0.333333333333333,
0.324975970727275,0.333333333333333,0.324975970727275,0.333333333333333,
0.324975970727275,0.333333333333333,0.324975970727275,0.333333333333333,
0.324975970727275,0.333333333333333,0.324975970727275,0.333333333333333,
0.324975970727275,0.333333333333333,0.324975970727275,0.333333333333333,
0.324975970727275,0.333333333333333,0.324975970727275,0.333333333333333,
0.324975970727275,0.333333333333333,0.324975970727275,0.333333333333333,
0.324975970727275,0.333333333333333,0.324975970727275,0.333333333333333,
0.324975970727275,0.333333333333333,0.324975970727275,0.333333333333333,
0.324975970727275,0.333333333333333,0.324975970727275,0.333333333333333,
0.324975970727275,0.333333333333333,0.324975970727275,0.333333333333333,
0.324975970727275,0.333333333333333,0.324975970727275,0.333333333333333,
0.324975970727275,0.333333333333333,0.324975970727275,0.333333333333333,
0.324975970727275,0.333333333333333,0.324975970727275,0.333333333333333,
0.324975970727275,0.333333333333333,0.324975970727275,0.333333333333333,
0.324975970727275,0.333333333333333,0.324975970727275,0.333333333333333,
0.324975970727275,0.333333333333333),(1.,0.974927912181824,1.,0.974927912181824,
1.,0.974927912181824,1.,0.974927912181824,1.,0.974927912181824,1.,0.974927912181824,
1.,0.974927912181824,1.,0.974927912181824,1.,0.974927912181824,1.,0.974927912181824,
1.,0.974927912181824,1.,0.974927912181824,1.,0.974927912181824,1.,0.974927912181824,
1.,0.974927912181824,1.,0.974927912181824,1.,0.974927912181824,1.,0.974927912181824,
1.,0.974927912181824,1.,0.974927912181824,1.,0.974927912181824,1.,0.974927912181824,
1.,0.974927912181824,1.,0.974927912181824,1.,0.974927912181824,1.,0.974927912181824,
1.,0.974927912181824,1.,0.974927912181824,1.,0.974927912181824,1.,0.974927912181824,
1.,0.974927912181824,1.,0.974927912181824,1.,0.974927912181824,1.,0.974927912181824,
1.,0.974927912181824,1.,0.974927912181824,1.,0.974927912181824,1.,0.974927912181824,
1.,0.974927912181824,1.,0.974927912181824,1.,0.974927912181824,1.,0.974927912181824,
1.,0.974927912181824,1.,0.974927912181824,1.,0.974927912181824,1.,0.974927912181824,
1.,0.974927912181824,1.,0.974927912181824,1.,0.974927912181824,1.,0.974927912181824,
1.,0.974927912181824,1.,0.974927912181824,1.,0.974927912181824,1.,0.974927912181824,
1.,0.974927912181824,1.,0.974927912181824,1.,0.974927912181824,1.,0.974927912181824,
1.,0.974927912181824,1.,0.974927912181824,1.,0.974927912181824,1.,0.974927912181824,
1.,0.974927912181824,1.,0.974927912181824,1.,0.974927912181824,1.,0.974927912181824,
1.,0.974927912181824,1.,0.974927912181824,1.,0.974927912181824,1.,0.974927912181824,
1.)))
REPRESENTATION_ITEM('')
SURFACE()
);
#37=B_SPLINE_CURVE_WITH_KNOTS('',3,(#4016,#4017,#4018,#4019,#4020,#4021,
#4022,#4023,#4024,#4025,#4026,#4027,#4028,#4029,#4030,#4031,#4032,#4033,
#4034,#4035,#4036,#4037,#4038,#4039,#4040,#4041,#4042,#4043,#4044,#4045,
#4046,#4047,#4048,#4049,#4050,#4051,#4052,#4053,#4054,#4055,#4056,#4057,
#4058,#4059,#4060,#4061,#4062,#4063,#4064,#4065,#4066,#4067,#4068,#4069,
#4070,#4071,#4072,#4073,#4074,#4075,#4076,#4077,#4078,#4079,#4080,#4081,
#4082,#4083,#4084,#4085,#4086,#4087,#4088,#4089,#4090,#4091,#4092,#4093,
#4094,#4095,#4096,#4097,#4098,#4099,#4100,#4101,#4102,#4103,#4104,#4105,
#4106,#4107,#4108,#4109,#4110,#4111,#4112,#4113,#4114,#4115,#4116,#4117,
#4118,#4119,#4120,#4121,#4122,#4123,#4124,#4125,#4126,#4127,#4128,#4129,
#4130,#4131,#4132,#4133,#4134,#4135,#4136,#4137,#4138,#4139,#4140,#4141,
#4142,#4143,#4144,#4145,#4146,#4147,#4148,#4149,#4150,#4151,#4152,#4153,
#4154,#4155,#4156,#4157,#4158,#4159,#4160,#4161,#4162,#4163,#4164,#4165,
#4166,#4167,#4168,#4169,#4170,#4171,#4172,#4173,#4174,#4175,#4176,#4177,
#4178,#4179,#4180,#4181,#4182,#4183,#4184,#4185,#4186,#4187,#4188,#4189,
#4190,#4191,#4192,#4193,#4194,#4195,#4196,#4197,#4198,#4199,#4200,#4201,
#4202,#4203,#4204,#4205,#4206,#4207,#4208,#4209,#4210,#4211,#4212,#4213,
#4214,#4215,#4216,#4217,#4218,#4219,#4220,#4221,#4222,#4223,#4224,#4225,
#4226,#4227,#4228,#4229,#4230,#4231,#4232,#4233,#4234,#4235,#4236,#4237,
#4238,#4239,#4240,#4241),.UNSPECIFIED.,.F.,.F.,(4,3,3,3,3,3,3,3,3,3,3,3,
3,3,3,3,3,3,3,3,3,3,3,3,3,3,3,3,3,3,3,3,3,3,3,3,3,3,3,3,3,3,3,3,3,3,3,3,
3,3,3,3,3,3,3,3,3,3,3,3,3,3,3,3,3,3,3,3,3,3,3,3,3,3,3,4),(0.505622875727277,
0.517988160946919,0.520338789948538,0.520905429501515,0.52717265317845,
0.533305555196153,0.535054704170684,0.537132103408132,0.54490516587315,
0.552830838419486,0.563272810879374,0.564486532614977,0.568546357321302,
0.584201801943347,0.599912293797433,0.607745612443856,0.615542041404178,
0.623350189503564,0.631056029515969,0.6456920985192,0.646842539795389,0.661283412185915,
0.66268246093576,0.677297370184217,0.67824270230549,0.682213846392151,0.691716213252626,
0.693762976426177,0.703275083336273,0.709570647326886,0.711645674836442,
0.720271652950763,0.725345909407201,0.734085257246458,0.741077503280732,
0.741106647260554,0.748435460391805,0.751860029569614,0.755793417502878,
0.757713958294146,0.76570174867477,0.770509331725024,0.773347178256837,
0.779737634087422,0.785225245947169,0.785728872145709,0.794897633981219,
0.799848096300002,0.799941160169314,0.807299117280385,0.81097809583592,
0.814316370179752,0.814657074391455,0.818043484932961,0.829372988613599,
0.833425179548027,0.83673094572467,0.840594242287955,0.844088902835742,
0.849462701918626,0.858804817057886,0.864830932205664,0.880572108534982,
0.896355862867048,0.912005776159084,0.917668473946477,0.927580474989763,
0.938300332984732,0.943299451007609,0.947100302390772,0.958694413066092,
0.961816216612921,0.969174173723996,0.972967833922422,0.974936906461323,
0.97653213083507),.UNSPECIFIED.);
#38=B_SPLINE_CURVE_WITH_KNOTS('',3,(#4245,#4246,#4247,#4248,#4249,#4250,
#4251,#4252,#4253,#4254,#4255,#4256,#4257,#4258,#4259,#4260,#4261,#4262,
#4263,#4264),.UNSPECIFIED.,.F.,.F.,(4,2,2,2,2,2,2,2,2,4),(0.,0.0116792314509369,
0.023969165868339,0.036250854130431,0.050588906263982,0.0651100872670082,
0.0773226289799043,0.089228359128315,0.0957523155277064,0.102264320227649),
 .UNSPECIFIED.);
#39=B_SPLINE_CURVE_WITH_KNOTS('',3,(#5257,#5258,#5259,#5260,#5261,#5262,
#5263,#5264,#5265,#5266,#5267,#5268,#5269,#5270,#5271,#5272,#5273,#5274,
#5275,#5276,#5277,#5278,#5279,#5280),.UNSPECIFIED.,.F.,.F.,(4,2,2,2,2,2,
2,2,2,2,2,4),(9.99991793790667E-7,0.0409954758355881,0.116426326291497,
0.178802457956817,0.201487661798833,0.216832635254426,0.230582029229575,
0.246869198666259,0.271413998785539,0.302825983747229,0.319030712132421,
0.33517722448993),.UNSPECIFIED.);
#40=B_SPLINE_CURVE_WITH_KNOTS('',3,(#5282,#5283,#5284,#5285,#5286,#5287,
#5288,#5289,#5290,#5291,#5292,#5293,#5294,#5295,#5296,#5297,#5298,#5299,
#5300,#5301,#5302,#5303,#5304,#5305,#5306,#5307,#5308,#5309,#5310,#5311,
#5312,#5313,#5314,#5315,#5316,#5317,#5318,#5319,#5320,#5321,#5322,#5323,
#5324,#5325,#5326,#5327,#5328,#5329,#5330,#5331,#5332,#5333,#5334,#5335,
#5336,#5337,#5338,#5339,#5340,#5341,#5342,#5343,#5344,#5345,#5346,#5347,
#5348,#5349,#5350,#5351,#5352,#5353,#5354,#5355,#5356,#5357,#5358,#5359,
#5360,#5361,#5362,#5363,#5364,#5365,#5366,#5367,#5368,#5369,#5370,#5371,
#5372,#5373,#5374,#5375,#5376,#5377,#5378,#5379,#5380,#5381,#5382,#5383,
#5384,#5385,#5386,#5387,#5388,#5389,#5390,#5391,#5392,#5393,#5394,#5395,
#5396,#5397,#5398,#5399,#5400,#5401,#5402,#5403,#5404,#5405,#5406,#5407,
#5408,#5409,#5410,#5411,#5412,#5413,#5414,#5415,#5416,#5417,#5418,#5419,
#5420,#5421,#5422,#5423,#5424,#5425,#5426,#5427,#5428,#5429,#5430,#5431,
#5432,#5433,#5434,#5435,#5436,#5437,#5438,#5439,#5440,#5441,#5442,#5443,
#5444,#5445,#5446,#5447,#5448,#5449,#5450,#5451,#5452,#5453,#5454,#5455,
#5456,#5457,#5458,#5459,#5460,#5461,#5462,#5463,#5464,#5465,#5466,#5467,
#5468,#5469,#5470,#5471,#5472,#5473,#5474,#5475,#5476,#5477,#5478,#5479,
#5480,#5481,#5482,#5483,#5484,#5485,#5486,#5487,#5488,#5489,#5490,#5491,
#5492,#5493,#5494,#5495,#5496,#5497,#5498,#5499,#5500,#5501,#5502,#5503,
#5504,#5505,#5506,#5507,#5508,#5509,#5510,#5511,#5512,#5513,#5514,#5515,
#5516,#5517,#5518,#5519,#5520,#5521,#5522,#5523,#5524,#5525,#5526,#5527,
#5528,#5529,#5530,#5531,#5532,#5533,#5534,#5535,#5536,#5537,#5538,#5539,
#5540,#5541,#5542,#5543,#5544,#5545,#5546,#5547,#5548,#5549,#5550,#5551,
#5552,#5553,#5554,#5555,#5556,#5557,#5558,#5559,#5560,#5561,#5562,#5563,
#5564,#5565,#5566,#5567,#5568,#5569,#5570,#5571,#5572,#5573,#5574,#5575,
#5576,#5577,#5578,#5579,#5580,#5581,#5582,#5583,#5584,#5585,#5586,#5587,
#5588,#5589,#5590,#5591,#5592,#5593,#5594,#5595,#5596,#5597,#5598,#5599,
#5600,#5601,#5602,#5603,#5604,#5605,#5606,#5607,#5608,#5609,#5610,#5611,
#5612,#5613,#5614,#5615,#5616,#5617,#5618,#5619,#5620,#5621,#5622,#5623,
#5624,#5625,#5626,#5627,#5628,#5629,#5630,#5631,#5632,#5633,#5634,#5635,
#5636,#5637,#5638,#5639,#5640,#5641,#5642,#5643,#5644,#5645,#5646,#5647,
#5648,#5649,#5650,#5651,#5652,#5653,#5654,#5655,#5656,#5657,#5658,#5659,
#5660,#5661,#5662,#5663,#5664,#5665,#5666,#5667,#5668,#5669,#5670,#5671,
#5672,#5673,#5674,#5675,#5676,#5677,#5678,#5679,#5680,#5681,#5682,#5683,
#5684,#5685,#5686,#5687,#5688,#5689,#5690,#5691,#5692,#5693,#5694,#5695,
#5696,#5697,#5698,#5699,#5700,#5701,#5702,#5703,#5704,#5705,#5706,#5707,
#5708,#5709,#5710,#5711,#5712,#5713,#5714,#5715,#5716,#5717,#5718,#5719,
#5720,#5721,#5722,#5723,#5724,#5725,#5726,#5727,#5728,#5729,#5730,#5731,
#5732,#5733,#5734,#5735,#5736,#5737,#5738,#5739,#5740,#5741,#5742,#5743,
#5744,#5745,#5746,#5747,#5748,#5749,#5750,#5751,#5752,#5753,#5754,#5755,
#5756,#5757,#5758,#5759,#5760,#5761,#5762,#5763,#5764,#5765,#5766,#5767,
#5768,#5769,#5770,#5771,#5772,#5773,#5774,#5775,#5776,#5777,#5778,#5779,
#5780,#5781,#5782,#5783,#5784,#5785,#5786,#5787,#5788,#5789,#5790,#5791,
#5792,#5793,#5794,#5795,#5796,#5797,#5798,#5799,#5800,#5801,#5802,#5803,
#5804,#5805,#5806,#5807,#5808,#5809,#5810,#5811,#5812,#5813,#5814,#5815,
#5816,#5817,#5818,#5819,#5820,#5821,#5822,#5823,#5824,#5825,#5826,#5827,
#5828,#5829,#5830,#5831,#5832,#5833,#5834,#5835,#5836,#5837,#5838,#5839,
#5840,#5841,#5842,#5843,#5844,#5845,#5846,#5847,#5848,#5849,#5850,#5851,
#5852,#5853,#5854,#5855,#5856,#5857,#5858,#5859,#5860,#5861,#5862,#5863,
#5864,#5865,#5866,#5867,#5868,#5869,#5870,#5871,#5872,#5873,#5874,#5875,
#5876,#5877,#5878,#5879,#5880,#5881,#5882,#5883,#5884,#5885,#5886,#5887,
#5888,#5889,#5890,#5891,#5892,#5893,#5894,#5895,#5896,#5897,#5898,#5899,
#5900,#5901,#5902,#5903,#5904,#5905,#5906,#5907,#5908,#5909,#5910,#5911,
#5912,#5913,#5914,#5915,#5916,#5917,#5918,#5919,#5920,#5921,#5922,#5923,
#5924,#5925,#5926,#5927,#5928,#5929,#5930,#5931,#5932,#5933,#5934,#5935,
#5936,#5937,#5938,#5939,#5940,#5941,#5942,#5943,#5944,#5945,#5946,#5947,
#5948,#5949,#5950,#5951,#5952,#5953,#5954,#5955,#5956,#5957,#5958,#5959,
#5960,#5961,#5962,#5963,#5964,#5965,#5966,#5967,#5968,#5969,#5970,#5971,
#5972,#5973,#5974,#5975,#5976,#5977,#5978,#5979,#5980,#5981,#5982,#5983,
#5984,#5985,#5986,#5987,#5988,#5989,#5990,#5991,#5992,#5993,#5994,#5995,
#5996,#5997,#5998,#5999,#6000,#6001,#6002,#6003,#6004,#6005,#6006,#6007,
#6008,#6009,#6010,#6011,#6012,#6013,#6014,#6015,#6016,#6017,#6018,#6019,
#6020,#6021,#6022,#6023,#6024,#6025,#6026,#6027,#6028,#6029,#6030,#6031,
#6032,#6033,#6034,#6035,#6036,#6037,#6038,#6039,#6040,#6041,#6042,#6043,
#6044,#6045,#6046,#6047,#6048,#6049,#6050,#6051,#6052,#6053,#6054,#6055,
#6056,#6057,#6058,#6059,#6060,#6061,#6062,#6063,#6064,#6065,#6066,#6067,
#6068,#6069,#6070,#6071,#6072,#6073,#6074,#6075,#6076,#6077,#6078,#6079,
#6080,#6081,#6082,#6083,#6084,#6085,#6086,#6087,#6088,#6089,#6090,#6091,
#6092,#6093,#6094,#6095,#6096,#6097,#6098,#6099,#6100,#6101,#6102,#6103,
#6104,#6105,#6106,#6107,#6108,#6109,#6110,#6111,#6112,#6113,#6114,#6115,
#6116,#6117,#6118,#6119,#6120,#6121,#6122,#6123,#6124,#6125,#6126,#6127,
#6128,#6129,#6130,#6131,#6132,#6133,#6134,#6135,#6136,#6137,#6138,#6139,
#6140,#6141,#6142,#6143,#6144,#6145,#6146,#6147,#6148,#6149,#6150,#6151,
#6152,#6153,#6154,#6155,#6156,#6157,#6158,#6159,#6160,#6161,#6162,#6163,
#6164,#6165,#6166,#6167,#6168,#6169,#6170,#6171,#6172,#6173,#6174,#6175,
#6176,#6177,#6178,#6179,#6180,#6181,#6182,#6183,#6184,#6185,#6186,#6187,
#6188,#6189,#6190,#6191,#6192,#6193,#6194,#6195,#6196,#6197,#6198,#6199,
#6200,#6201,#6202,#6203,#6204,#6205,#6206,#6207,#6208,#6209,#6210,#6211,
#6212,#6213,#6214,#6215,#6216,#6217,#6218,#6219,#6220,#6221,#6222,#6223,
#6224,#6225,#6226,#6227,#6228,#6229,#6230,#6231,#6232,#6233,#6234,#6235,
#6236,#6237,#6238,#6239,#6240,#6241,#6242,#6243,#6244,#6245,#6246,#6247,
#6248,#6249,#6250,#6251,#6252,#6253,#6254,#6255,#6256,#6257,#6258,#6259,
#6260,#6261,#6262,#6263,#6264,#6265,#6266,#6267,#6268,#6269,#6270,#6271,
#6272,#6273,#6274,#6275,#6276,#6277,#6278,#6279,#6280,#6281,#6282,#6283,
#6284,#6285,#6286,#6287,#6288,#6289,#6290,#6291,#6292,#6293,#6294,#6295,
#6296,#6297,#6298,#6299,#6300,#6301,#6302,#6303,#6304,#6305,#6306,#6307,
#6308,#6309,#6310,#6311,#6312,#6313,#6314,#6315,#6316,#6317,#6318,#6319,
#6320,#6321,#6322,#6323,#6324,#6325,#6326,#6327,#6328,#6329,#6330,#6331,
#6332,#6333,#6334,#6335,#6336,#6337,#6338,#6339,#6340,#6341,#6342,#6343,
#6344,#6345,#6346,#6347,#6348,#6349,#6350,#6351,#6352,#6353,#6354,#6355,
#6356,#6357,#6358,#6359,#6360,#6361,#6362,#6363,#6364,#6365,#6366,#6367,
#6368,#6369,#6370,#6371,#6372,#6373,#6374,#6375,#6376,#6377,#6378,#6379,
#6380,#6381,#6382,#6383,#6384,#6385,#6386,#6387,#6388,#6389,#6390,#6391,
#6392,#6393,#6394,#6395,#6396,#6397,#6398,#6399,#6400,#6401,#6402,#6403,
#6404,#6405,#6406,#6407,#6408,#6409,#6410,#6411,#6412,#6413,#6414,#6415,
#6416,#6417,#6418,#6419,#6420,#6421,#6422,#6423,#6424,#6425,#6426,#6427,
#6428,#6429,#6430,#6431,#6432,#6433,#6434,#6435,#6436,#6437,#6438,#6439,
#6440,#6441,#6442,#6443,#6444,#6445,#6446,#6447,#6448,#6449,#6450,#6451,
#6452,#6453,#6454,#6455,#6456,#6457,#6458,#6459,#6460,#6461,#6462,#6463,
#6464,#6465,#6466,#6467,#6468,#6469,#6470,#6471,#6472,#6473,#6474,#6475,
#6476),.UNSPECIFIED.,.F.,.F.,(4,3,3,3,3,3,3,3,3,3,3,3,3,3,3,3,3,3,3,3,3,
3,3,3,3,3,3,3,3,3,3,3,3,3,3,3,3,3,3,3,3,3,3,3,3,3,3,3,3,3,3,3,3,3,3,3,3,
3,3,3,3,3,3,3,3,3,3,3,3,3,3,3,3,3,3,3,3,3,3,3,3,3,3,3,3,3,3,3,3,3,3,3,3,
3,3,3,3,3,3,3,3,3,3,3,3,3,3,3,3,3,3,3,3,3,3,3,3,3,3,3,3,3,3,3,3,3,3,3,3,
3,3,3,3,3,3,3,3,3,3,3,3,3,3,3,3,3,3,3,3,3,3,3,3,3,3,3,3,3,3,3,3,3,3,3,3,
3,3,3,3,3,3,3,3,3,3,3,3,3,3,3,3,3,3,3,3,3,3,3,3,3,3,3,3,3,3,3,3,3,3,3,3,
3,3,3,3,3,3,3,3,3,3,3,3,3,3,3,3,3,3,3,3,3,3,3,3,3,3,3,3,3,3,3,3,3,3,3,3,
3,3,3,3,3,3,3,3,3,3,3,3,3,3,3,3,3,3,3,3,3,3,3,3,3,3,3,3,3,3,3,3,3,3,3,3,
3,3,3,3,3,3,3,3,3,3,3,3,3,3,3,3,3,3,3,3,3,3,3,3,3,3,3,3,3,3,3,3,3,3,3,3,
3,3,3,3,3,3,3,3,3,3,3,3,3,3,3,3,3,3,3,3,3,3,3,3,3,3,3,3,3,3,3,3,3,3,3,3,
3,3,3,3,3,3,3,3,3,3,3,3,3,3,3,3,3,3,3,3,3,3,3,3,3,3,3,3,3,3,3,3,3,3,3,3,
3,3,3,3,3,3,3,3,3,3,3,3,3,3,3,3,3,4),(0.0434521468850362,0.0461873441657508,
0.0489269991702234,0.0516650038763463,0.0544039305096017,0.0571428571428571,
0.059877893422679,0.0626138848522894,0.065352304603236,0.0680886385499103,
0.0708234140605492,0.0714285714285714,0.0741636077083921,0.0768995991380027,
0.0796380188889482,0.0823743528356205,0.0851091283462598,0.0857142857142857,
0.0884493219941073,0.0911853134237064,0.093923733174652,0.0966600671213259,
0.0993948426319571,0.1,0.102735036279824,0.105471027709443,0.108209447460392,
0.110945781407079,0.113680556917732,0.114285714285714,0.117020750565535,
0.119756741995136,0.122495161746079,0.125231495692751,0.127966271203388,
0.128571428571429,0.131306464851251,0.134042456280861,0.136780876031805,
0.139517209978476,0.142251985489111,0.142857142857143,0.145592179136964,
0.148328170566579,0.151066590317524,0.153802924264195,0.156537699774842,
0.157142857142857,0.159877893422678,0.162613884852275,0.165352304603217,
0.168088638549894,0.170823414060526,0.171428571428571,0.174163607708387,
0.176899599137999,0.179638018888945,0.182374352835622,0.185109128346255,
0.185714285714286,0.188449321994121,0.191185313423734,0.193923733174678,
0.196660067121338,0.199394842631953,0.2,0.202735036279828,0.205471027709437,
0.208209447460376,0.210945781407047,0.21368055691771,0.214285714285714,
0.217020750565534,0.21975674199515,0.222495161746102,0.225231495692787,
0.227966271203424,0.228571428571429,0.231306464851263,0.23404245628089,
0.236780876031837,0.239517209978489,0.242251985489098,0.242857142857143,
0.245592179136972,0.248328170566582,0.251066590317521,0.253802924264199,
0.256537699774829,0.257142857142857,0.259877893422686,0.26261388485229,
0.265352304603237,0.268088638549896,0.270823414060528,0.271428571428571,
0.2741636077084,0.276899599138014,0.27963801888896,0.282374352835653,0.285109128346286,
0.285714285714286,0.28844932199411,0.291185313423707,0.293923733174651,
0.296660067121322,0.299394842631966,0.3,0.302735036279835,0.305471027709446,
0.308209447460395,0.310945781407089,0.313680556917723,0.314285714285714,
0.31702075056553,0.319756741995162,0.322495161746109,0.325231495692777,
0.32796627120343,0.328571428571429,0.331306464851255,0.334042456280855,
0.336780876031804,0.339517209978488,0.342251985489124,0.342857142857143,
0.345592179136954,0.348328170566521,0.351066590317465,0.353802924264142,
0.3565376997748,0.357142857142857,0.359877893422679,0.362613884852294,0.365352304603241,
0.368088638549919,0.370823414060555,0.371428571428571,0.374163607708382,
0.376899599137964,0.37963801888891,0.382374352835591,0.385109128346204,
0.385714285714286,0.388449321994103,0.391185313423703,0.393923733174653,
0.396660067121351,0.399394842632005,0.4,0.402735036279825,0.405471027709447,
0.408209447460393,0.410945781407081,0.413680556917718,0.414285714285714,
0.417020750565532,0.419756741995165,0.422495161746111,0.425231495692786,
0.427966271203415,0.428571428571429,0.431306464851253,0.434042456280863,
0.436780876031811,0.439517209978483,0.442251985489122,0.442857142857143,
0.445592179136974,0.448328170566577,0.451066590317522,0.453802924264206,
0.45653769977484,0.457142857142857,0.459877893422679,0.462613884852274,
0.46535230460322,0.468088638549892,0.470823414060526,0.471428571428571,
0.474163607708389,0.476899599137977,0.479638018888923,0.482374352835603,
0.485109128346238,0.485714285714286,0.488449321994099,0.491185313423694,
0.493923733174635,0.496660067121315,0.499394842631956,0.5,0.502735036279827,
0.505471027709436,0.508209447460376,0.510945781407021,0.513680556917665,
0.514285714285714,0.517020750565532,0.519756741995121,0.522495161746054,
0.525231495692741,0.527966271203371,0.528571428571429,0.531306464851231,
0.534042456280826,0.53678087603177,0.539517209978444,0.542251985489095,
0.542857142857143,0.545592179136964,0.54832817056658,0.551066590317522,
0.553802924264182,0.556537699774845,0.557142857142857,0.559877893422674,
0.562613884852282,0.565352304603234,0.568088638549889,0.570823414060542,
0.571428571428571,0.574163607708401,0.576899599138019,0.579638018888965,
0.582374352835606,0.585109128346239,0.585714285714286,0.588449321994126,
0.591185313423754,0.5939237331747,0.596660067121342,0.599394842631994,0.6,
0.60273503627982,0.605471027709411,0.608209447460348,0.610945781407044,
0.613680556917701,0.614285714285714,0.617020750565514,0.619756741995111,
0.622495161746057,0.625231495692732,0.627966271203357,0.628571428571429,
0.631306464851258,0.634042456280886,0.636780876031825,0.639517209978507,
0.642251985489135,0.642857142857143,0.645592179136954,0.648328170566526,
0.651066590317477,0.653802924264148,0.656537699774774,0.657142857142857,
0.65987789342268,0.662613884852296,0.66535230460324,0.668088638549891,0.670823414060543,
0.671428571428571,0.674163607708392,0.676899599138033,0.679638018888974,
0.682374352835659,0.685109128346312,0.685714285714286,0.688449321994104,
0.6911853134237,0.693923733174643,0.696660067121325,0.699394842631902,0.7,
0.702735036279801,0.705471027709409,0.708209447460343,0.710945781407061,
0.713680556917779,0.714285714285714,0.717020750565534,0.719756741995116,
0.722495161746074,0.72523149569276,0.727966271203408,0.728571428571429,
0.731306464851277,0.734042456280897,0.736780876031841,0.739517209978497,
0.742251985489142,0.742857142857143,0.745592179136962,0.748328170566599,
0.751066590317548,0.753802924264176,0.756537699774778,0.757142857142857,
0.759877893422655,0.762613884852237,0.765352304603176,0.768088638549865,
0.770823414060485,0.771428571428571,0.774163607708391,0.776899599137959,
0.77963801888891,0.782374352835568,0.785109128346213,0.785714285714286,
0.788449321994106,0.791185313423719,0.793923733174654,0.796660067121301,
0.799394842631947,0.8,0.802735036279805,0.805471027709432,0.808209447460388,
0.810945781407092,0.813680556917737,0.814285714285714,0.817020750565548,
0.819756741995165,0.822495161746102,0.825231495692781,0.827966271203429,
0.828571428571429,0.831306464851221,0.83404245628079,0.836780876031735,
0.8395172099784,0.842251985489027,0.842857142857143,0.845592179136976,0.84832817056658,
0.851066590317534,0.853802924264192,0.856537699774856,0.857142857142857,
0.85987789342267,0.86261388485227,0.865352304603208,0.868088638549884,0.870823414060506,
0.871428571428571,0.874163607708391,0.876899599137982,0.87963801888893,
0.882374352835648,0.88510912834627,0.885714285714286,0.888449321994109,
0.891185313423738,0.893923733174676,0.896660067121346,0.899394842631965,
0.9,0.902735036279826,0.9054710277094,0.908209447460347,0.910945781407016,
0.913680556917645,0.914285714285714,0.917020750565528,0.919756741995146,
0.922495161746083,0.925231495692764,0.927966271203396,0.928571428571429,
0.931306464851252,0.934042456280889,0.936780876031843,0.939517209978495,
0.942251985489148,0.942857142857143,0.945592179136907,0.948328170566525,
0.951066590317466,0.953802924264139,0.956537699774797,0.957142857142857,
0.95987789342267,0.962613884852283,0.965352304603234,0.968088638549892,
0.970823414060527,0.971428571428571,0.974163607708378,0.976899599137948,
0.979638018888884,0.982374352835551,0.985109128346214,0.985714285714286,
0.988448991390083,0.991186079127076,0.992296011182497),.UNSPECIFIED.);
#41=B_SPLINE_CURVE_WITH_KNOTS('',3,(#6478,#6479,#6480,#6481,#6482,#6483,
#6484,#6485,#6486,#6487,#6488,#6489,#6490,#6491,#6492,#6493,#6494,#6495,
#6496,#6497,#6498,#6499,#6500,#6501,#6502,#6503,#6504,#6505,#6506,#6507,
#6508,#6509,#6510,#6511,#6512,#6513,#6514,#6515,#6516,#6517,#6518,#6519,
#6520,#6521,#6522,#6523,#6524,#6525,#6526,#6527,#6528,#6529,#6530,#6531,
#6532,#6533,#6534,#6535,#6536,#6537,#6538,#6539,#6540,#6541,#6542,#6543,
#6544,#6545,#6546,#6547,#6548,#6549,#6550,#6551,#6552,#6553,#6554,#6555,
#6556,#6557,#6558,#6559,#6560,#6561,#6562,#6563,#6564,#6565,#6566,#6567,
#6568,#6569,#6570,#6571,#6572,#6573,#6574,#6575,#6576,#6577,#6578,#6579,
#6580,#6581,#6582,#6583,#6584,#6585,#6586,#6587,#6588,#6589,#6590,#6591,
#6592,#6593,#6594,#6595,#6596,#6597,#6598,#6599,#6600,#6601,#6602,#6603,
#6604,#6605,#6606,#6607,#6608,#6609,#6610,#6611,#6612,#6613,#6614,#6615,
#6616,#6617,#6618,#6619,#6620,#6621,#6622,#6623,#6624,#6625,#6626,#6627,
#6628,#6629,#6630,#6631,#6632,#6633,#6634,#6635,#6636,#6637,#6638,#6639,
#6640,#6641,#6642,#6643,#6644,#6645,#6646,#6647,#6648,#6649,#6650,#6651,
#6652,#6653,#6654,#6655,#6656,#6657,#6658,#6659,#6660,#6661,#6662,#6663,
#6664,#6665,#6666,#6667,#6668,#6669,#6670,#6671,#6672,#6673,#6674,#6675,
#6676,#6677,#6678,#6679,#6680,#6681,#6682,#6683,#6684,#6685,#6686,#6687,
#6688,#6689,#6690,#6691,#6692,#6693,#6694,#6695,#6696,#6697,#6698,#6699,
#6700,#6701,#6702,#6703,#6704,#6705,#6706,#6707,#6708,#6709,#6710,#6711,
#6712,#6713,#6714,#6715,#6716,#6717,#6718,#6719,#6720,#6721,#6722,#6723,
#6724,#6725,#6726,#6727,#6728,#6729,#6730,#6731,#6732,#6733,#6734,#6735,
#6736,#6737,#6738,#6739,#6740,#6741,#6742,#6743,#6744,#6745,#6746,#6747,
#6748,#6749,#6750,#6751,#6752,#6753,#6754,#6755,#6756,#6757,#6758,#6759,
#6760,#6761,#6762,#6763,#6764,#6765,#6766,#6767,#6768,#6769,#6770,#6771,
#6772,#6773,#6774,#6775,#6776,#6777,#6778,#6779,#6780,#6781,#6782,#6783,
#6784,#6785,#6786,#6787,#6788,#6789,#6790,#6791,#6792,#6793,#6794,#6795,
#6796,#6797,#6798,#6799,#6800,#6801,#6802,#6803,#6804,#6805,#6806,#6807,
#6808,#6809,#6810,#6811,#6812,#6813,#6814,#6815,#6816,#6817,#6818,#6819,
#6820,#6821,#6822,#6823,#6824,#6825,#6826,#6827,#6828,#6829,#6830,#6831,
#6832,#6833,#6834,#6835,#6836,#6837,#6838,#6839,#6840,#6841,#6842,#6843,
#6844,#6845,#6846,#6847,#6848,#6849,#6850,#6851,#6852,#6853,#6854,#6855,
#6856,#6857,#6858,#6859,#6860,#6861,#6862,#6863,#6864,#6865,#6866,#6867,
#6868,#6869,#6870,#6871,#6872,#6873,#6874,#6875,#6876,#6877,#6878,#6879,
#6880,#6881,#6882,#6883,#6884,#6885,#6886,#6887,#6888,#6889,#6890,#6891,
#6892,#6893,#6894,#6895,#6896,#6897,#6898,#6899,#6900,#6901,#6902,#6903,
#6904,#6905,#6906,#6907,#6908,#6909,#6910,#6911,#6912,#6913,#6914,#6915,
#6916,#6917,#6918,#6919,#6920,#6921,#6922,#6923,#6924,#6925,#6926,#6927,
#6928,#6929,#6930,#6931,#6932,#6933,#6934,#6935,#6936,#6937,#6938,#6939,
#6940,#6941,#6942,#6943,#6944,#6945,#6946,#6947,#6948,#6949,#6950,#6951,
#6952,#6953,#6954,#6955,#6956,#6957,#6958,#6959,#6960,#6961,#6962,#6963,
#6964,#6965,#6966,#6967,#6968,#6969,#6970,#6971,#6972,#6973,#6974,#6975,
#6976,#6977,#6978,#6979,#6980,#6981,#6982,#6983,#6984,#6985,#6986,#6987,
#6988,#6989,#6990,#6991,#6992,#6993,#6994,#6995,#6996,#6997,#6998,#6999,
#7000,#7001,#7002,#7003,#7004,#7005,#7006,#7007,#7008,#7009,#7010,#7011,
#7012,#7013,#7014,#7015,#7016,#7017,#7018,#7019,#7020,#7021,#7022,#7023,
#7024,#7025,#7026,#7027,#7028,#7029,#7030,#7031,#7032,#7033,#7034,#7035,
#7036,#7037,#7038,#7039,#7040,#7041,#7042,#7043,#7044,#7045,#7046,#7047,
#7048,#7049,#7050,#7051,#7052,#7053,#7054,#7055,#7056,#7057,#7058,#7059,
#7060,#7061,#7062,#7063,#7064,#7065,#7066,#7067,#7068,#7069,#7070,#7071,
#7072,#7073,#7074,#7075,#7076,#7077,#7078,#7079,#7080,#7081,#7082,#7083,
#7084,#7085,#7086,#7087,#7088,#7089,#7090,#7091,#7092,#7093,#7094,#7095,
#7096,#7097,#7098,#7099,#7100,#7101,#7102,#7103,#7104,#7105,#7106,#7107,
#7108,#7109,#7110,#7111,#7112,#7113,#7114,#7115,#7116,#7117,#7118,#7119,
#7120,#7121,#7122,#7123,#7124,#7125,#7126,#7127,#7128,#7129,#7130,#7131,
#7132,#7133,#7134,#7135,#7136,#7137,#7138,#7139,#7140,#7141,#7142,#7143,
#7144,#7145,#7146,#7147,#7148,#7149,#7150,#7151,#7152,#7153,#7154,#7155,
#7156,#7157,#7158,#7159,#7160,#7161,#7162,#7163,#7164,#7165,#7166,#7167,
#7168,#7169,#7170,#7171,#7172,#7173,#7174,#7175,#7176,#7177,#7178,#7179,
#7180,#7181,#7182,#7183,#7184,#7185,#7186,#7187,#7188,#7189,#7190,#7191,
#7192,#7193,#7194,#7195,#7196,#7197,#7198,#7199,#7200,#7201,#7202,#7203,
#7204,#7205,#7206,#7207,#7208,#7209,#7210,#7211,#7212,#7213,#7214,#7215,
#7216,#7217,#7218,#7219,#7220,#7221,#7222,#7223,#7224,#7225,#7226,#7227,
#7228,#7229,#7230,#7231,#7232,#7233,#7234,#7235,#7236,#7237,#7238,#7239,
#7240,#7241,#7242,#7243,#7244,#7245,#7246,#7247,#7248,#7249,#7250,#7251,
#7252,#7253,#7254,#7255,#7256,#7257,#7258,#7259,#7260,#7261,#7262,#7263,
#7264,#7265,#7266,#7267,#7268,#7269,#7270,#7271,#7272,#7273,#7274,#7275,
#7276,#7277,#7278,#7279,#7280,#7281,#7282,#7283,#7284,#7285,#7286,#7287,
#7288,#7289,#7290,#7291,#7292,#7293,#7294,#7295,#7296,#7297,#7298,#7299,
#7300,#7301,#7302,#7303,#7304,#7305,#7306,#7307,#7308,#7309,#7310,#7311,
#7312,#7313,#7314,#7315,#7316,#7317,#7318,#7319,#7320,#7321,#7322,#7323,
#7324,#7325,#7326,#7327,#7328,#7329,#7330,#7331,#7332,#7333,#7334,#7335,
#7336,#7337,#7338,#7339,#7340,#7341,#7342,#7343,#7344,#7345,#7346,#7347,
#7348,#7349,#7350,#7351,#7352,#7353,#7354,#7355,#7356,#7357,#7358,#7359,
#7360,#7361,#7362,#7363,#7364,#7365,#7366,#7367,#7368,#7369,#7370,#7371,
#7372,#7373,#7374,#7375,#7376,#7377,#7378,#7379,#7380,#7381,#7382,#7383,
#7384,#7385,#7386,#7387,#7388,#7389,#7390,#7391,#7392,#7393,#7394,#7395,
#7396,#7397,#7398,#7399,#7400,#7401,#7402,#7403,#7404,#7405,#7406,#7407,
#7408,#7409,#7410,#7411,#7412,#7413,#7414,#7415,#7416,#7417,#7418,#7419,
#7420,#7421,#7422,#7423,#7424,#7425,#7426,#7427,#7428,#7429,#7430,#7431,
#7432,#7433,#7434,#7435,#7436,#7437,#7438,#7439,#7440,#7441,#7442,#7443,
#7444,#7445,#7446,#7447,#7448,#7449,#7450,#7451,#7452,#7453,#7454,#7455,
#7456,#7457,#7458,#7459,#7460,#7461,#7462,#7463,#7464,#7465,#7466,#7467,
#7468,#7469,#7470,#7471,#7472,#7473,#7474,#7475,#7476,#7477,#7478,#7479,
#7480,#7481,#7482,#7483,#7484,#7485,#7486,#7487,#7488,#7489,#7490,#7491,
#7492,#7493,#7494,#7495,#7496,#7497,#7498,#7499,#7500,#7501,#7502,#7503,
#7504,#7505,#7506,#7507,#7508,#7509,#7510,#7511,#7512,#7513,#7514,#7515,
#7516,#7517,#7518,#7519,#7520,#7521,#7522,#7523,#7524,#7525,#7526,#7527,
#7528,#7529,#7530,#7531,#7532,#7533,#7534,#7535,#7536,#7537,#7538,#7539,
#7540,#7541,#7542,#7543,#7544,#7545,#7546,#7547,#7548,#7549,#7550,#7551,
#7552,#7553,#7554,#7555,#7556,#7557,#7558,#7559,#7560,#7561,#7562,#7563,
#7564,#7565,#7566,#7567,#7568,#7569,#7570,#7571,#7572,#7573,#7574,#7575,
#7576,#7577,#7578,#7579,#7580,#7581,#7582,#7583,#7584,#7585,#7586,#7587,
#7588,#7589,#7590,#7591,#7592,#7593,#7594,#7595,#7596,#7597,#7598,#7599,
#7600,#7601,#7602,#7603,#7604,#7605,#7606,#7607,#7608,#7609,#7610,#7611,
#7612,#7613,#7614,#7615,#7616,#7617,#7618,#7619,#7620,#7621,#7622,#7623,
#7624,#7625,#7626,#7627,#7628,#7629,#7630,#7631,#7632,#7633,#7634,#7635,
#7636,#7637,#7638,#7639,#7640,#7641,#7642,#7643,#7644,#7645,#7646,#7647,
#7648,#7649,#7650,#7651,#7652,#7653,#7654,#7655,#7656,#7657,#7658,#7659,
#7660,#7661,#7662,#7663,#7664,#7665,#7666,#7667,#7668,#7669,#7670,#7671,
#7672,#7673,#7674,#7675,#7676,#7677,#7678,#7679,#7680,#7681,#7682,#7683,
#7684,#7685,#7686,#7687,#7688,#7689,#7690,#7691,#7692,#7693,#7694,#7695,
#7696,#7697,#7698,#7699,#7700,#7701,#7702),.UNSPECIFIED.,.F.,.F.,(4,3,3,
3,3,3,3,3,3,3,3,3,3,3,3,3,3,3,3,3,3,3,3,3,3,3,3,3,3,3,3,3,3,3,3,3,3,3,3,
3,3,3,3,3,3,3,3,3,3,3,3,3,3,3,3,3,3,3,3,3,3,3,3,3,3,3,3,3,3,3,3,3,3,3,3,
3,3,3,3,3,3,3,3,3,3,3,3,3,3,3,3,3,3,3,3,3,3,3,3,3,3,3,3,3,3,3,3,3,3,3,3,
3,3,3,3,3,3,3,3,3,3,3,3,3,3,3,3,3,3,3,3,3,3,3,3,3,3,3,3,3,3,3,3,3,3,3,3,
3,3,3,3,3,3,3,3,3,3,3,3,3,3,3,3,3,3,3,3,3,3,3,3,3,3,3,3,3,3,3,3,3,3,3,3,
3,3,3,3,3,3,3,3,3,3,3,3,3,3,3,3,3,3,3,3,3,3,3,3,3,3,3,3,3,3,3,3,3,3,3,3,
3,3,3,3,3,3,3,3,3,3,3,3,3,3,3,3,3,3,3,3,3,3,3,3,3,3,3,3,3,3,3,3,3,3,3,3,
3,3,3,3,3,3,3,3,3,3,3,3,3,3,3,3,3,3,3,3,3,3,3,3,3,3,3,3,3,3,3,3,3,3,3,3,
3,3,3,3,3,3,3,3,3,3,3,3,3,3,3,3,3,3,3,3,3,3,3,3,3,3,3,3,3,3,3,3,3,3,3,3,
3,3,3,3,3,3,3,3,3,3,3,3,3,3,3,3,3,3,3,3,3,3,3,3,3,3,3,3,3,3,3,3,3,3,3,3,
3,3,3,3,3,3,3,3,3,3,3,3,3,3,3,3,3,3,3,3,3,3,3,3,3,3,3,3,3,3,3,3,3,3,3,3,
3,3,3,3,3,3,3,3,3,4),(0.023206495763431,0.0257239292490225,0.0282450189887502,
0.0285714285714286,0.0310923942810177,0.0336100262627011,0.0361278182416742,
0.0386450010909029,0.0411660098458559,0.0428571428571429,0.0453781085667337,
0.0478957405484203,0.0504135325273945,0.0529307153766255,0.0554517241315774,
0.0571428571428571,0.059663822852449,0.0621814548341318,0.0646992468131065,
0.0672164296623363,0.0697374384172902,0.0714285714285714,0.0739495371381627,
0.076467169119844,0.0789849610988178,0.0815021439480481,0.084023152703002,
0.0857142857142857,0.088235251423873,0.0907528834055563,0.0932706753845298,
0.0957878582337589,0.098308866988713,0.1,0.10252096570959,0.105038597691268,
0.107556389670243,0.110073572519475,0.112594581274429,0.114285714285714,
0.116806679995307,0.119324311976988,0.121842103955963,0.124359286805196,
0.126880295560147,0.128571428571429,0.131092394281013,0.133610026262683,
0.136127818241655,0.138645001090891,0.141166009845844,0.142857142857143,
0.145378108566732,0.147895740548422,0.150413532527396,0.152930715376634,
0.155451724131588,0.157142857142857,0.159663822852444,0.162181454834132,
0.164699246813105,0.167216429662338,0.169737438417291,0.171428571428571,
0.173949537138155,0.176467169119835,0.178984961098808,0.181502143948042,
0.184023152702995,0.185714285714286,0.188235251423882,0.190752883405569,
0.193270675384542,0.195787858233769,0.19830886698872,0.2,0.202520965709589,
0.205038597691277,0.207556389670251,0.210073572519482,0.212594581274431,
0.214285714285714,0.216806679995304,0.219324311976987,0.221842103955961,
0.224359286805185,0.226880295560131,0.228571428571429,0.231092394281016,
0.23361002626269,0.236127818241664,0.238645001090892,0.241166009845845,
0.242857142857143,0.245378108566735,0.247895740548416,0.25041353252739,
0.252930715376624,0.255451724131578,0.257142857142857,0.259663822852451,
0.262181454834138,0.264699246813112,0.267216429662339,0.269737438417293,
0.271428571428571,0.273949537138167,0.276467169119861,0.278984961098836,
0.281502143948073,0.284023152703024,0.285714285714286,0.288235251423881,
0.290752883405567,0.293270675384543,0.295787858233765,0.298308866988717,
0.3,0.302520965709596,0.30503859769128,0.307556389670252,0.31007357251948,
0.312594581274429,0.314285714285714,0.316806679995287,0.319324311976971,
0.321842103955943,0.324359286805174,0.326880295560125,0.328571428571429,
0.33109239428101,0.333610026262706,0.336127818241682,0.338645001090916,
0.34116600984586,0.342857142857143,0.345378108566721,0.347895740548409,
0.350413532527381,0.352930715376615,0.355451724131572,0.357142857142857,
0.359663822852443,0.362181454834099,0.364699246813074,0.367216429662306,
0.369737438417254,0.371428571428571,0.373949537138159,0.376467169119829,
0.378984961098804,0.381502143948016,0.384023152702971,0.385714285714286,
0.38823525142388,0.390752883405583,0.393270675384557,0.395787858233787,
0.398308866988739,0.4,0.402520965709584,0.405038597691256,0.407556389670229,
0.41007357251945,0.412594581274402,0.414285714285714,0.416806679995293,
0.419324311976974,0.421842103955951,0.424359286805177,0.426880295560129,
0.428571428571429,0.43109239428102,0.433610026262699,0.436127818241675,
0.438645001090902,0.441166009845859,0.442857142857143,0.445378108566734,
0.447895740548424,0.450413532527398,0.452930715376623,0.455451724131568,
0.457142857142857,0.459663822852451,0.462181454834118,0.464699246813092,
0.467216429662323,0.469737438417271,0.471428571428571,0.473949537138167,
0.476467169119847,0.478984961098823,0.481502143948057,0.484023152703002,
0.485714285714286,0.488235251423869,0.490752883405553,0.493270675384525,
0.495787858233748,0.498308866988705,0.5,0.502520965709591,0.505038597691261,
0.507556389670239,0.510073572519473,0.512594581274426,0.514285714285714,
0.516806679995304,0.519324311976992,0.521842103955964,0.524359286805211,
0.526880295560167,0.528571428571429,0.531092394281006,0.533610026262715,
0.53612781824169,0.538645001090917,0.541166009845867,0.542857142857143,
0.54537810856674,0.547895740548404,0.550413532527373,0.552930715376607,
0.555451724131568,0.557142857142857,0.559663822852453,0.562181454834126,
0.564699246813095,0.567216429662329,0.569737438417277,0.571428571428571,
0.57394953713816,0.576467169119855,0.578984961098832,0.581502143948056,
0.584023152703013,0.585714285714286,0.58823525142385,0.590752883405521,
0.593270675384497,0.595787858233757,0.598308866988711,0.6,0.602520965709609,
0.605038597691303,0.607556389670285,0.610073572519503,0.612594581274451,
0.614285714285714,0.616806679995288,0.619324311976971,0.621842103955946,
0.624359286805171,0.626880295560112,0.628571428571429,0.631092394281018,
0.633610026262711,0.636127818241686,0.638645001090888,0.641166009845846,
0.642857142857143,0.645378108566731,0.647895740548437,0.65041353252741,
0.652930715376643,0.655451724131588,0.657142857142857,0.659663822852448,
0.662181454834114,0.664699246813086,0.667216429662316,0.669737438417258,
0.671428571428571,0.673949537138158,0.67646716911984,0.67898496109881,0.681502143948056,
0.684023152703005,0.685714285714286,0.688235251423882,0.690752883405585,
0.693270675384566,0.695787858233805,0.698308866988762,0.7,0.7025209657096,
0.705038597691304,0.707556389670276,0.710073572519505,0.712594581274454,
0.714285714285714,0.716806679995296,0.719324311976947,0.721842103955917,
0.724359286805131,0.726880295560062,0.728571428571429,0.731092394281035,
0.733610026262732,0.736127818241713,0.738645001090942,0.741166009845897,
0.742857142857143,0.745378108566722,0.747895740548415,0.750413532527391,
0.752930715376615,0.75545172413156,0.757142857142857,0.759663822852465,
0.762181454834149,0.764699246813129,0.767216429662351,0.769737438417299,
0.771428571428571,0.773949537138153,0.776467169119842,0.778984961098804,
0.781502143948032,0.784023152702966,0.785714285714286,0.788235251423874,
0.790752883405565,0.793270675384545,0.795787858233779,0.79830886698873,
0.8,0.802520965709581,0.805038597691266,0.807556389670235,0.810073572519464,
0.812594581274417,0.814285714285714,0.816806679995304,0.819324311977038,
0.82184210395602,0.824359286805267,0.826880295560212,0.828571428571429,
0.831092394280992,0.833610026262696,0.836127818241669,0.838645001090894,
0.841166009845847,0.842857142857143,0.845378108566734,0.847895740548434,
0.850413532527405,0.852930715376647,0.855451724131588,0.857142857142857,
0.859663822852412,0.86218145483413,0.864699246813113,0.867216429662333,
0.869737438417301,0.871428571428571,0.873949537138163,0.876467169119875,
0.878984961098842,0.881502143948064,0.884023152703011,0.885714285714286,
0.888235251423884,0.890752883405557,0.893270675384532,0.895787858233751,
0.89830886698871,0.9,0.902520965709585,0.90503859769128,0.90755638967025,
0.910073572519495,0.912594581274447,0.914285714285714,0.916806679995308,
0.919324311977025,0.921842103956005,0.92435928680524,0.926880295560179,
0.928571428571429,0.931092394281023,0.933610026262707,0.936127818241673,
0.938645001090907,0.941166009845862,0.942857142857143,0.945378108566741,
0.947895740548478,0.950413532527452,0.952930715376688,0.955451724131655,
0.957142857142857,0.959663822852439,0.962181454834151,0.964699246813133,
0.967216429662383,0.969737438417352,0.971428571428572,0.973949537138156,
0.976467169119865,0.978984961098835,0.98150214394807,0.984023152703024,
0.985714285714286,0.988235247165933,0.990852917116709,0.993470587067484),
 .UNSPECIFIED.);
#42=B_SPLINE_CURVE_WITH_KNOTS('',3,(#7749,#7750,#7751,#7752,#7753,#7754,
#7755,#7756,#7757,#7758,#7759,#7760,#7761,#7762,#7763,#7764,#7765,#7766,
#7767,#7768,#7769,#7770,#7771,#7772),.UNSPECIFIED.,.F.,.F.,(4,2,2,2,2,2,
2,2,2,2,2,4),(9.99997522730752E-7,0.0373212594653978,0.0837444328860222,
0.127999538981999,0.168138172256258,0.195435295899977,0.213313281312765,
0.225803333956439,0.236147330446737,0.247437939130784,0.264210428398769,
0.300000948832372),.UNSPECIFIED.);
#43=B_SPLINE_CURVE_WITH_KNOTS('',3,(#7774,#7775,#7776,#7777,#7778,#7779,
#7780,#7781,#7782,#7783,#7784,#7785,#7786,#7787,#7788,#7789,#7790,#7791,
#7792,#7793),.UNSPECIFIED.,.F.,.F.,(4,2,2,2,2,2,2,2,2,4),(1.10999191885525E-10,
0.0114224997171007,0.0238925436228599,0.0362967112517097,0.0484706620322139,
0.0615854552568996,0.0761727562847049,0.0902646072806745,0.0975841853107938,
0.104919277808089),.UNSPECIFIED.);
#44=B_SPLINE_CURVE_WITH_KNOTS('',3,(#8082,#8083,#8084,#8085,#8086,#8087,
#8088,#8089,#8090,#8091,#8092,#8093,#8094,#8095,#8096,#8097,#8098,#8099,
#8100,#8101,#8102,#8103,#8104,#8105,#8106,#8107,#8108,#8109,#8110,#8111,
#8112,#8113,#8114,#8115,#8116,#8117,#8118,#8119,#8120,#8121,#8122,#8123,
#8124,#8125,#8126,#8127,#8128,#8129,#8130,#8131,#8132,#8133,#8134,#8135,
#8136,#8137,#8138,#8139,#8140,#8141,#8142,#8143,#8144,#8145,#8146,#8147,
#8148,#8149,#8150,#8151,#8152,#8153,#8154,#8155,#8156,#8157,#8158,#8159,
#8160,#8161,#8162,#8163,#8164,#8165,#8166,#8167,#8168,#8169,#8170,#8171,
#8172,#8173,#8174,#8175,#8176,#8177,#8178,#8179,#8180,#8181,#8182,#8183,
#8184,#8185,#8186,#8187,#8188,#8189,#8190,#8191,#8192,#8193,#8194,#8195,
#8196,#8197,#8198,#8199,#8200,#8201,#8202,#8203,#8204,#8205,#8206,#8207,
#8208,#8209,#8210,#8211,#8212,#8213,#8214,#8215,#8216,#8217,#8218,#8219,
#8220,#8221,#8222,#8223,#8224,#8225,#8226,#8227,#8228,#8229,#8230,#8231,
#8232,#8233,#8234,#8235,#8236,#8237,#8238,#8239,#8240,#8241,#8242,#8243,
#8244,#8245,#8246,#8247,#8248,#8249,#8250,#8251,#8252,#8253,#8254,#8255,
#8256,#8257,#8258,#8259,#8260,#8261,#8262,#8263,#8264,#8265,#8266,#8267,
#8268,#8269,#8270,#8271,#8272,#8273,#8274,#8275,#8276,#8277,#8278,#8279,
#8280,#8281,#8282,#8283,#8284,#8285,#8286,#8287,#8288,#8289,#8290,#8291,
#8292,#8293,#8294,#8295),.UNSPECIFIED.,.F.,.F.,(4,3,3,3,3,3,3,3,3,3,3,3,
3,3,3,3,3,3,3,3,3,3,3,3,3,3,3,3,3,3,3,3,3,3,3,3,3,3,3,3,3,3,3,3,3,3,3,3,
3,3,3,3,3,3,3,3,3,3,3,3,3,3,3,3,3,3,3,3,3,3,3,4),(0.00581528851415237,0.0198568721625981,
0.0211877409662844,0.0290621003554579,0.0370052281862515,0.0512291292287845,
0.0529041937053002,0.0644502614911372,0.0685278037786423,0.0841159711918372,
0.0919424126878769,0.0997790634725718,0.115448233246931,0.123085234974729,
0.131078038316822,0.146752253766709,0.162464053667518,0.178185986283123,
0.186042112011005,0.193890422727681,0.209550039573698,0.225138286678832,
0.240355181941911,0.240630028387911,0.248484045283646,0.256473909857358,
0.266662688666893,0.269672668683709,0.272111589151239,0.278265459195196,
0.284331412054608,0.288069318728516,0.298990155425507,0.303816384109195,
0.306319527110955,0.309583018903716,0.313229521738243,0.313648898796403,
0.319844455210027,0.325614289631532,0.328307642167298,0.332940771087925,
0.339713242837541,0.342966385538194,0.34605817259295,0.349007561947065,
0.350295757223643,0.357625128909093,0.364110633619828,0.372283872279993,
0.377813672911342,0.380677984752505,0.385953186130796,0.386942615650894,
0.395918491286659,0.401601359021794,0.408640030677264,0.411952448078052,
0.416260102392695,0.425748224011398,0.427444685160084,0.437067118782021,
0.443188392123352,0.445577589134499,0.458668272113456,0.4602363325054,0.467565704190851,
0.469398047112214,0.470772304303236,0.472833690089769,0.473864382983036,
0.474895075721047),.UNSPECIFIED.);
#45=B_SPLINE_SURFACE_WITH_KNOTS('',1,3,((#3726,#3727,#3728,#3729,#3730,
#3731,#3732,#3733,#3734,#3735,#3736,#3737,#3738,#3739,#3740,#3741,#3742,
#3743,#3744,#3745,#3746,#3747,#3748,#3749,#3750,#3751,#3752,#3753,#3754,
#3755,#3756,#3757,#3758,#3759,#3760,#3761,#3762,#3763,#3764,#3765,#3766,
#3767,#3768,#3769,#3770,#3771,#3772,#3773,#3774,#3775,#3776,#3777,#3778,
#3779,#3780,#3781,#3782,#3783,#3784,#3785,#3786,#3787,#3788,#3789,#3790,
#3791,#3792,#3793,#3794,#3795,#3796,#3797,#3798,#3799,#3800,#3801,#3802,
#3803,#3804,#3805,#3806,#3807,#3808,#3809,#3810,#3811,#3812,#3813,#3814,
#3815,#3816,#3817,#3818,#3819,#3820,#3821,#3822,#3823,#3824,#3825,#3826,
#3827,#3828,#3829,#3830,#3831,#3832,#3833,#3834,#3835,#3836,#3837,#3838,
#3839,#3840,#3841,#3842,#3843,#3844,#3845,#3846,#3847,#3848,#3849,#3850,
#3851,#3852,#3853,#3854,#3855,#3856,#3857,#3858,#3859,#3860,#3861,#3862,
#3863,#3864,#3865,#3866,#3867,#3868,#3869),(#3870,#3871,#3872,#3873,#3874,
#3875,#3876,#3877,#3878,#3879,#3880,#3881,#3882,#3883,#3884,#3885,#3886,
#3887,#3888,#3889,#3890,#3891,#3892,#3893,#3894,#3895,#3896,#3897,#3898,
#3899,#3900,#3901,#3902,#3903,#3904,#3905,#3906,#3907,#3908,#3909,#3910,
#3911,#3912,#3913,#3914,#3915,#3916,#3917,#3918,#3919,#3920,#3921,#3922,
#3923,#3924,#3925,#3926,#3927,#3928,#3929,#3930,#3931,#3932,#3933,#3934,
#3935,#3936,#3937,#3938,#3939,#3940,#3941,#3942,#3943,#3944,#3945,#3946,
#3947,#3948,#3949,#3950,#3951,#3952,#3953,#3954,#3955,#3956,#3957,#3958,
#3959,#3960,#3961,#3962,#3963,#3964,#3965,#3966,#3967,#3968,#3969,#3970,
#3971,#3972,#3973,#3974,#3975,#3976,#3977,#3978,#3979,#3980,#3981,#3982,
#3983,#3984,#3985,#3986,#3987,#3988,#3989,#3990,#3991,#3992,#3993,#3994,
#3995,#3996,#3997,#3998,#3999,#4000,#4001,#4002,#4003,#4004,#4005,#4006,
#4007,#4008,#4009,#4010,#4011,#4012,#4013)),.UNSPECIFIED.,.F.,.T.,.F.,(2,
2),(4,2,2,2,2,2,2,2,2,2,2,2,2,2,2,2,2,2,2,2,2,2,2,2,2,2,2,2,2,2,2,2,2,2,
2,2,2,2,2,2,2,2,2,2,2,2,2,2,2,2,2,2,2,2,2,2,2,2,2,2,2,2,2,2,2,2,2,2,2,2,
2,4),(0.,1.),(-4.79963010313954E-5,-1.80312514392642E-5,-3.04872664319862E-6,
1.1933798152867E-5,4.18988477449981E-5,7.18638973371293E-5,0.00010182894692926,
0.000116811471725326,0.000131793996521392,0.000161759046113523,0.000191724095705654,
0.000221689145297785,0.000251654194889916,0.000281619244482047,0.000296601769278113,
0.000311584294074179,0.00034154934366631,0.000371514393258441,0.000401479442850572,
0.000416461967646638,0.000431444492442703,0.000461409542034834,0.000491374591626965,
0.000521339641219097,0.000551304690811228,0.000581269740403359,0.00061123478999549,
0.000641199839587621,0.000671164889179752,0.000701129938771884,0.000731094988364015,
0.000761060037956146,0.000791025087548277,0.000820990137140408,0.000850955186732539,
0.000880920236324671,0.000910885285916802,0.000940850335508933,0.000970815385101064,
0.000985797909897129,0.0010007804346932,0.00103074548428533,0.00106071053387746,
0.00109067558346959,0.00110565810826565,0.00112064063306172,0.00115060568265385,
0.00118057073224598,0.00121053578183811,0.00124050083143024,0.00127046588102238,
0.00130043093061451,0.00133039598020664,0.00136036102979877,0.0013903260793909,
0.00142029112898303,0.00145025617857516,0.00148022122816729,0.00151018627775943,
0.00154015132735156,0.00157011637694369,0.00160008142653582,0.00163004647612795,
0.00166001152572008,0.00168997657531221,0.00171994162490434,0.00174990667449647,
0.00177987172408861,0.00180983677368074,0.0018248192984768,0.00183980182327287,
0.001869766872865),.UNSPECIFIED.);
#46=B_SPLINE_SURFACE_WITH_KNOTS('',1,3,((#7794,#7795,#7796,#7797,#7798,
#7799,#7800,#7801,#7802,#7803,#7804,#7805,#7806,#7807,#7808,#7809,#7810,
#7811,#7812,#7813,#7814,#7815,#7816,#7817,#7818,#7819,#7820,#7821,#7822,
#7823,#7824,#7825,#7826,#7827,#7828,#7829,#7830,#7831,#7832,#7833,#7834,
#7835,#7836,#7837,#7838,#7839,#7840,#7841,#7842,#7843,#7844,#7845,#7846,
#7847,#7848,#7849,#7850,#7851,#7852,#7853,#7854,#7855,#7856,#7857,#7858,
#7859,#7860,#7861,#7862,#7863,#7864,#7865,#7866,#7867,#7868,#7869,#7870,
#7871,#7872,#7873,#7874,#7875,#7876,#7877,#7878,#7879,#7880,#7881,#7882,
#7883,#7884,#7885,#7886,#7887,#7888,#7889,#7890,#7891,#7892,#7893,#7894,
#7895,#7896,#7897,#7898,#7899,#7900,#7901,#7902,#7903,#7904,#7905,#7906,
#7907,#7908,#7909,#7910,#7911,#7912,#7913,#7914,#7915,#7916,#7917,#7918,
#7919,#7920,#7921,#7922,#7923,#7924,#7925,#7926,#7927,#7928,#7929,#7930,
#7931,#7932,#7933,#7934,#7935,#7936,#7937),(#7938,#7939,#7940,#7941,#7942,
#7943,#7944,#7945,#7946,#7947,#7948,#7949,#7950,#7951,#7952,#7953,#7954,
#7955,#7956,#7957,#7958,#7959,#7960,#7961,#7962,#7963,#7964,#7965,#7966,
#7967,#7968,#7969,#7970,#7971,#7972,#7973,#7974,#7975,#7976,#7977,#7978,
#7979,#7980,#7981,#7982,#7983,#7984,#7985,#7986,#7987,#7988,#7989,#7990,
#7991,#7992,#7993,#7994,#7995,#7996,#7997,#7998,#7999,#8000,#8001,#8002,
#8003,#8004,#8005,#8006,#8007,#8008,#8009,#8010,#8011,#8012,#8013,#8014,
#8015,#8016,#8017,#8018,#8019,#8020,#8021,#8022,#8023,#8024,#8025,#8026,
#8027,#8028,#8029,#8030,#8031,#8032,#8033,#8034,#8035,#8036,#8037,#8038,
#8039,#8040,#8041,#8042,#8043,#8044,#8045,#8046,#8047,#8048,#8049,#8050,
#8051,#8052,#8053,#8054,#8055,#8056,#8057,#8058,#8059,#8060,#8061,#8062,
#8063,#8064,#8065,#8066,#8067,#8068,#8069,#8070,#8071,#8072,#8073,#8074,
#8075,#8076,#8077,#8078,#8079,#8080,#8081)),.UNSPECIFIED.,.F.,.T.,.F.,(2,
2),(4,2,2,2,2,2,2,2,2,2,2,2,2,2,2,2,2,2,2,2,2,2,2,2,2,2,2,2,2,2,2,2,2,2,
2,2,2,2,2,2,2,2,2,2,2,2,2,2,2,2,2,2,2,2,2,2,2,2,2,2,2,2,2,2,2,2,2,2,2,2,
2,4),(0.,1.),(-4.79963010313954E-5,-1.80312514392642E-5,-3.04872664319862E-6,
1.1933798152867E-5,4.18988477449981E-5,7.18638973371293E-5,0.00010182894692926,
0.000116811471725326,0.000131793996521392,0.000161759046113523,0.000191724095705654,
0.000221689145297785,0.000251654194889916,0.000281619244482047,0.000296601769278113,
0.000311584294074179,0.00034154934366631,0.000371514393258441,0.000401479442850572,
0.000416461967646638,0.000431444492442703,0.000461409542034834,0.000491374591626965,
0.000521339641219097,0.000551304690811228,0.000581269740403359,0.00061123478999549,
0.000641199839587621,0.000671164889179752,0.000701129938771884,0.000731094988364015,
0.000761060037956146,0.000791025087548277,0.000820990137140408,0.000850955186732539,
0.000880920236324671,0.000910885285916802,0.000940850335508933,0.000970815385101064,
0.000985797909897129,0.0010007804346932,0.00103074548428533,0.00106071053387746,
0.00109067558346959,0.00110565810826565,0.00112064063306172,0.00115060568265385,
0.00118057073224598,0.00121053578183811,0.00124050083143024,0.00127046588102238,
0.00130043093061451,0.00133039598020664,0.00136036102979877,0.0013903260793909,
0.00142029112898303,0.00145025617857516,0.00148022122816729,0.00151018627775943,
0.00154015132735156,0.00157011637694369,0.00160008142653582,0.00163004647612795,
0.00166001152572008,0.00168997657531221,0.00171994162490434,0.00174990667449647,
0.00177987172408861,0.00180983677368074,0.0018248192984768,0.00183980182327287,
0.001869766872865),.UNSPECIFIED.);
#49=SHAPE_REPRESENTATION_RELATIONSHIP('SRR','None',#9589,#55);
#55=ADVANCED_BREP_SHAPE_REPRESENTATION('',(#67),#9557);
#61=STYLED_ITEM('',(#9628),#67);
#67=MANIFOLD_SOLID_BREP('Body1',#2407);
#79=FACE_BOUND('',#413,.T.);
#80=FACE_BOUND('',#419,.T.);
#81=FACE_BOUND('',#421,.T.);
#82=FACE_BOUND('',#423,.T.);
#83=FACE_BOUND('',#425,.T.);
#126=PLANE('',#2604);
#127=PLANE('',#2605);
#128=PLANE('',#2606);
#129=PLANE('',#2607);
#130=PLANE('',#2608);
#131=PLANE('',#2609);
#132=PLANE('',#2610);
#133=PLANE('',#2611);
#134=PLANE('',#2612);
#257=FACE_OUTER_BOUND('',#408,.T.);
#258=FACE_OUTER_BOUND('',#409,.T.);
#259=FACE_OUTER_BOUND('',#410,.T.);
#260=FACE_OUTER_BOUND('',#411,.T.);
#261=FACE_OUTER_BOUND('',#412,.T.);
#262=FACE_OUTER_BOUND('',#414,.T.);
#263=FACE_OUTER_BOUND('',#415,.T.);
#264=FACE_OUTER_BOUND('',#416,.T.);
#265=FACE_OUTER_BOUND('',#417,.T.);
#266=FACE_OUTER_BOUND('',#418,.T.);
#267=FACE_OUTER_BOUND('',#420,.T.);
#268=FACE_OUTER_BOUND('',#422,.T.);
#269=FACE_OUTER_BOUND('',#424,.T.);
#270=FACE_OUTER_BOUND('',#426,.T.);
#271=FACE_OUTER_BOUND('',#427,.T.);
#272=FACE_OUTER_BOUND('',#428,.T.);
#408=EDGE_LOOP('',(#1917,#1918,#1919,#1920,#1921));
#409=EDGE_LOOP('',(#1922,#1923,#1924,#1925,#1926));
#410=EDGE_LOOP('',(#1927,#1928,#1929,#1930));
#411=EDGE_LOOP('',(#1931,#1932,#1933,#1934));
#412=EDGE_LOOP('',(#1935,#1936,#1937,#1938));
#413=EDGE_LOOP('',(#1939,#1940,#1941,#1942));
#414=EDGE_LOOP('',(#1943,#1944,#1945,#1946));
#415=EDGE_LOOP('',(#1947,#1948,#1949,#1950));
#416=EDGE_LOOP('',(#1951,#1952,#1953,#1954));
#417=EDGE_LOOP('',(#1955,#1956,#1957,#1958));
#418=EDGE_LOOP('',(#1959));
#419=EDGE_LOOP('',(#1960));
#420=EDGE_LOOP('',(#1961));
#421=EDGE_LOOP('',(#1962));
#422=EDGE_LOOP('',(#1963));
#423=EDGE_LOOP('',(#1964,#1965,#1966,#1967));
#424=EDGE_LOOP('',(#1968));
#425=EDGE_LOOP('',(#1969,#1970));
#426=EDGE_LOOP('',(#1971,#1972));
#427=EDGE_LOOP('',(#1973,#1974,#1975,#1976,#1977));
#428=EDGE_LOOP('',(#1978,#1979,#1980,#1981,#1982));
#616=LINE('',#4243,#866);
#617=LINE('',#4266,#867);
#618=LINE('',#7707,#868);
#619=LINE('',#7713,#869);
#620=LINE('',#7719,#870);
#621=LINE('',#7725,#871);
#622=LINE('',#7728,#872);
#623=LINE('',#7732,#873);
#624=LINE('',#7733,#874);
#625=LINE('',#7734,#875);
#626=LINE('',#7737,#876);
#627=LINE('',#7739,#877);
#628=LINE('',#7740,#878);
#629=LINE('',#7742,#879);
#630=LINE('',#7744,#880);
#866=VECTOR('',#3043,10.);
#867=VECTOR('',#3044,10.);
#868=VECTOR('',#3053,3.);
#869=VECTOR('',#3060,1.5);
#870=VECTOR('',#3067,2.5);
#871=VECTOR('',#3072,1000.);
#872=VECTOR('',#3075,1000.);
#873=VECTOR('',#3078,1000.);
#874=VECTOR('',#3079,1000.);
#875=VECTOR('',#3080,1000.);
#876=VECTOR('',#3083,1000.);
#877=VECTOR('',#3084,1000.);
#878=VECTOR('',#3085,1000.);
#879=VECTOR('',#3088,1000.);
#880=VECTOR('',#3091,1000.);
#1041=CIRCLE('',#2591,0.500322308738118);
#1042=CIRCLE('',#2592,0.500483076506173);
#1043=CIRCLE('',#2594,3.);
#1044=CIRCLE('',#2595,3.);
#1045=CIRCLE('',#2597,1.5);
#1046=CIRCLE('',#2598,1.5);
#1047=CIRCLE('',#2600,2.5);
#1048=CIRCLE('',#2601,2.5);
#1049=CIRCLE('',#2602,2.5);
#1050=CIRCLE('',#2603,2.5);
#1171=VERTEX_POINT('',#4014);
#1172=VERTEX_POINT('',#4015);
#1173=VERTEX_POINT('',#4242);
#1174=VERTEX_POINT('',#4244);
#1175=VERTEX_POINT('',#4265);
#1176=VERTEX_POINT('',#5255);
#1177=VERTEX_POINT('',#5256);
#1178=VERTEX_POINT('',#5281);
#1179=VERTEX_POINT('',#7704);
#1180=VERTEX_POINT('',#7706);
#1181=VERTEX_POINT('',#7710);
#1182=VERTEX_POINT('',#7712);
#1183=VERTEX_POINT('',#7716);
#1184=VERTEX_POINT('',#7718);
#1185=VERTEX_POINT('',#7721);
#1186=VERTEX_POINT('',#7722);
#1187=VERTEX_POINT('',#7724);
#1188=VERTEX_POINT('',#7726);
#1189=VERTEX_POINT('',#7730);
#1190=VERTEX_POINT('',#7731);
#1191=VERTEX_POINT('',#7736);
#1192=VERTEX_POINT('',#7738);
#1426=EDGE_CURVE('',#1171,#1172,#37,.T.);
#1427=EDGE_CURVE('',#1171,#1173,#616,.T.);
#1428=EDGE_CURVE('',#1174,#1173,#38,.T.);
#1429=EDGE_CURVE('',#1175,#1174,#617,.T.);
#1430=EDGE_CURVE('',#1172,#1175,#1041,.T.);
#1431=EDGE_CURVE('',#1176,#1177,#39,.T.);
#1432=EDGE_CURVE('',#1176,#1178,#40,.T.);
#1433=EDGE_CURVE('',#1178,#1171,#1042,.T.);
#1434=EDGE_CURVE('',#1177,#1172,#41,.T.);
#1435=EDGE_CURVE('',#1179,#1179,#1043,.T.);
#1436=EDGE_CURVE('',#1179,#1180,#618,.T.);
#1437=EDGE_CURVE('',#1180,#1180,#1044,.T.);
#1438=EDGE_CURVE('',#1181,#1181,#1045,.T.);
#1439=EDGE_CURVE('',#1181,#1182,#619,.T.);
#1440=EDGE_CURVE('',#1182,#1182,#1046,.T.);
#1441=EDGE_CURVE('',#1183,#1183,#1047,.T.);
#1442=EDGE_CURVE('',#1183,#1184,#620,.T.);
#1443=EDGE_CURVE('',#1184,#1184,#1048,.T.);
#1444=EDGE_CURVE('',#1185,#1186,#1049,.T.);
#1445=EDGE_CURVE('',#1185,#1187,#621,.T.);
#1446=EDGE_CURVE('',#1187,#1188,#1050,.T.);
#1447=EDGE_CURVE('',#1186,#1188,#622,.T.);
#1448=EDGE_CURVE('',#1189,#1190,#623,.T.);
#1449=EDGE_CURVE('',#1186,#1189,#624,.T.);
#1450=EDGE_CURVE('',#1188,#1190,#625,.T.);
#1451=EDGE_CURVE('',#1185,#1191,#626,.T.);
#1452=EDGE_CURVE('',#1191,#1192,#627,.T.);
#1453=EDGE_CURVE('',#1187,#1192,#628,.T.);
#1454=EDGE_CURVE('',#1191,#1189,#629,.T.);
#1455=EDGE_CURVE('',#1192,#1190,#630,.T.);
#1456=EDGE_CURVE('',#1177,#1176,#42,.T.);
#1457=EDGE_CURVE('',#1173,#1174,#43,.T.);
#1458=EDGE_CURVE('',#1175,#1178,#44,.T.);
#1917=ORIENTED_EDGE('',*,*,#1426,.F.);
#1918=ORIENTED_EDGE('',*,*,#1427,.T.);
#1919=ORIENTED_EDGE('',*,*,#1428,.F.);
#1920=ORIENTED_EDGE('',*,*,#1429,.F.);
#1921=ORIENTED_EDGE('',*,*,#1430,.F.);
#1922=ORIENTED_EDGE('',*,*,#1431,.F.);
#1923=ORIENTED_EDGE('',*,*,#1432,.T.);
#1924=ORIENTED_EDGE('',*,*,#1433,.T.);
#1925=ORIENTED_EDGE('',*,*,#1426,.T.);
#1926=ORIENTED_EDGE('',*,*,#1434,.F.);
#1927=ORIENTED_EDGE('',*,*,#1435,.T.);
#1928=ORIENTED_EDGE('',*,*,#1436,.T.);
#1929=ORIENTED_EDGE('',*,*,#1437,.F.);
#1930=ORIENTED_EDGE('',*,*,#1436,.F.);
#1931=ORIENTED_EDGE('',*,*,#1438,.T.);
#1932=ORIENTED_EDGE('',*,*,#1439,.T.);
#1933=ORIENTED_EDGE('',*,*,#1440,.F.);
#1934=ORIENTED_EDGE('',*,*,#1439,.F.);
#1935=ORIENTED_EDGE('',*,*,#1441,.T.);
#1936=ORIENTED_EDGE('',*,*,#1442,.T.);
#1937=ORIENTED_EDGE('',*,*,#1443,.F.);
#1938=ORIENTED_EDGE('',*,*,#1442,.F.);
#1939=ORIENTED_EDGE('',*,*,#1444,.F.);
#1940=ORIENTED_EDGE('',*,*,#1445,.T.);
#1941=ORIENTED_EDGE('',*,*,#1446,.T.);
#1942=ORIENTED_EDGE('',*,*,#1447,.F.);
#1943=ORIENTED_EDGE('',*,*,#1448,.F.);
#1944=ORIENTED_EDGE('',*,*,#1449,.F.);
#1945=ORIENTED_EDGE('',*,*,#1447,.T.);
#1946=ORIENTED_EDGE('',*,*,#1450,.T.);
#1947=ORIENTED_EDGE('',*,*,#1451,.T.);
#1948=ORIENTED_EDGE('',*,*,#1452,.T.);
#1949=ORIENTED_EDGE('',*,*,#1453,.F.);
#1950=ORIENTED_EDGE('',*,*,#1445,.F.);
#1951=ORIENTED_EDGE('',*,*,#1454,.F.);
#1952=ORIENTED_EDGE('',*,*,#1451,.F.);
#1953=ORIENTED_EDGE('',*,*,#1444,.T.);
#1954=ORIENTED_EDGE('',*,*,#1449,.T.);
#1955=ORIENTED_EDGE('',*,*,#1453,.T.);
#1956=ORIENTED_EDGE('',*,*,#1455,.T.);
#1957=ORIENTED_EDGE('',*,*,#1450,.F.);
#1958=ORIENTED_EDGE('',*,*,#1446,.F.);
#1959=ORIENTED_EDGE('',*,*,#1443,.T.);
#1960=ORIENTED_EDGE('',*,*,#1438,.F.);
#1961=ORIENTED_EDGE('',*,*,#1441,.F.);
#1962=ORIENTED_EDGE('',*,*,#1440,.T.);
#1963=ORIENTED_EDGE('',*,*,#1435,.F.);
#1964=ORIENTED_EDGE('',*,*,#1452,.F.);
#1965=ORIENTED_EDGE('',*,*,#1454,.T.);
#1966=ORIENTED_EDGE('',*,*,#1448,.T.);
#1967=ORIENTED_EDGE('',*,*,#1455,.F.);
#1968=ORIENTED_EDGE('',*,*,#1437,.T.);
#1969=ORIENTED_EDGE('',*,*,#1456,.T.);
#1970=ORIENTED_EDGE('',*,*,#1431,.T.);
#1971=ORIENTED_EDGE('',*,*,#1428,.T.);
#1972=ORIENTED_EDGE('',*,*,#1457,.T.);
#1973=ORIENTED_EDGE('',*,*,#1427,.F.);
#1974=ORIENTED_EDGE('',*,*,#1433,.F.);
#1975=ORIENTED_EDGE('',*,*,#1458,.F.);
#1976=ORIENTED_EDGE('',*,*,#1429,.T.);
#1977=ORIENTED_EDGE('',*,*,#1457,.F.);
#1978=ORIENTED_EDGE('',*,*,#1432,.F.);
#1979=ORIENTED_EDGE('',*,*,#1456,.F.);
#1980=ORIENTED_EDGE('',*,*,#1434,.T.);
#1981=ORIENTED_EDGE('',*,*,#1430,.T.);
#1982=ORIENTED_EDGE('',*,*,#1458,.T.);
#2254=CYLINDRICAL_SURFACE('',#2593,3.);
#2255=CYLINDRICAL_SURFACE('',#2596,1.5);
#2256=CYLINDRICAL_SURFACE('',#2599,2.5);
#2325=ADVANCED_FACE('',(#257),#45,.T.);
#2326=ADVANCED_FACE('',(#258),#35,.T.);
#2327=ADVANCED_FACE('',(#259),#2254,.T.);
#2328=ADVANCED_FACE('',(#260),#2255,.F.);
#2329=ADVANCED_FACE('',(#261,#79),#2256,.T.);
#2330=ADVANCED_FACE('',(#262),#126,.F.);
#2331=ADVANCED_FACE('',(#263),#127,.T.);
#2332=ADVANCED_FACE('',(#264),#128,.F.);
#2333=ADVANCED_FACE('',(#265),#129,.T.);
#2334=ADVANCED_FACE('',(#266,#80),#130,.T.);
#2335=ADVANCED_FACE('',(#267,#81),#131,.F.);
#2336=ADVANCED_FACE('',(#268,#82),#132,.F.);
#2337=ADVANCED_FACE('',(#269,#83),#133,.T.);
#2338=ADVANCED_FACE('',(#270),#134,.F.);
#2339=ADVANCED_FACE('',(#271),#46,.T.);
#2340=ADVANCED_FACE('',(#272),#36,.T.);
#2407=CLOSED_SHELL('',(#2325,#2326,#2327,#2328,#2329,#2330,#2331,#2332,
#2333,#2334,#2335,#2336,#2337,#2338,#2339,#2340));
#2590=AXIS2_PLACEMENT_3D('',#3725,#3041,#3042);
#2591=AXIS2_PLACEMENT_3D('',#4267,#3045,#3046);
#2592=AXIS2_PLACEMENT_3D('',#6477,#3047,#3048);
#2593=AXIS2_PLACEMENT_3D('',#7703,#3049,#3050);
#2594=AXIS2_PLACEMENT_3D('',#7705,#3051,#3052);
#2595=AXIS2_PLACEMENT_3D('',#7708,#3054,#3055);
#2596=AXIS2_PLACEMENT_3D('',#7709,#3056,#3057);
#2597=AXIS2_PLACEMENT_3D('',#7711,#3058,#3059);
#2598=AXIS2_PLACEMENT_3D('',#7714,#3061,#3062);
#2599=AXIS2_PLACEMENT_3D('',#7715,#3063,#3064);
#2600=AXIS2_PLACEMENT_3D('',#7717,#3065,#3066);
#2601=AXIS2_PLACEMENT_3D('',#7720,#3068,#3069);
#2602=AXIS2_PLACEMENT_3D('',#7723,#3070,#3071);
#2603=AXIS2_PLACEMENT_3D('',#7727,#3073,#3074);
#2604=AXIS2_PLACEMENT_3D('',#7729,#3076,#3077);
#2605=AXIS2_PLACEMENT_3D('',#7735,#3081,#3082);
#2606=AXIS2_PLACEMENT_3D('',#7741,#3086,#3087);
#2607=AXIS2_PLACEMENT_3D('',#7743,#3089,#3090);
#2608=AXIS2_PLACEMENT_3D('',#7745,#3092,#3093);
#2609=AXIS2_PLACEMENT_3D('',#7746,#3094,#3095);
#2610=AXIS2_PLACEMENT_3D('',#7747,#3096,#3097);
#2611=AXIS2_PLACEMENT_3D('',#7748,#3098,#3099);
#2612=AXIS2_PLACEMENT_3D('',#7773,#3100,#3101);
#3041=DIRECTION('axis',(0.,0.,1.));
#3042=DIRECTION('refdir',(1.,0.,0.));
#3043=DIRECTION('',(-0.37576669481491,-0.860797132775134,0.34326037824658));
#3044=DIRECTION('',(-0.319221716607877,-0.41191406004893,0.853477769353091));
#3045=DIRECTION('center_axis',(0.405557992046095,0.691428751056098,-0.597870385033866));
#3046=DIRECTION('ref_axis',(-0.0717210395256331,-0.627988322886608,-0.774910807001314));
#3047=DIRECTION('center_axis',(0.421321917352423,0.692775741612449,-0.58527738192399));
#3048=DIRECTION('ref_axis',(0.0676843725596094,0.619533124468324,0.782047014825661));
#3049=DIRECTION('center_axis',(-0.499999999999995,0.866025403784442,0.));
#3050=DIRECTION('ref_axis',(-0.866025403784442,-0.499999999999995,0.));
#3051=DIRECTION('center_axis',(0.499999999999995,-0.866025403784442,0.));
#3052=DIRECTION('ref_axis',(0.866025403784442,0.499999999999995,0.));
#3053=DIRECTION('',(0.499999999999995,-0.866025403784442,0.));
#3054=DIRECTION('center_axis',(0.499999999999995,-0.866025403784442,0.));
#3055=DIRECTION('ref_axis',(0.866025403784442,0.499999999999995,0.));
#3056=DIRECTION('center_axis',(0.,0.,-1.));
#3057=DIRECTION('ref_axis',(-1.,0.,0.));
#3058=DIRECTION('center_axis',(0.,0.,1.));
#3059=DIRECTION('ref_axis',(1.,0.,0.));
#3060=DIRECTION('',(0.,0.,-1.));
#3061=DIRECTION('center_axis',(0.,0.,1.));
#3062=DIRECTION('ref_axis',(1.,0.,0.));
#3063=DIRECTION('center_axis',(0.,0.,-1.));
#3064=DIRECTION('ref_axis',(-1.,0.,0.));
#3065=DIRECTION('center_axis',(0.,0.,1.));
#3066=DIRECTION('ref_axis',(1.,0.,0.));
#3067=DIRECTION('',(0.,0.,1.));
#3068=DIRECTION('center_axis',(0.,0.,1.));
#3069=DIRECTION('ref_axis',(1.,0.,0.));
#3070=DIRECTION('center_axis',(0.,0.,-1.));
#3071=DIRECTION('ref_axis',(-1.,0.,0.));
#3072=DIRECTION('',(0.,0.,-1.));
#3073=DIRECTION('center_axis',(0.,0.,-1.));
#3074=DIRECTION('ref_axis',(-1.,0.,0.));
#3075=DIRECTION('',(0.,0.,-1.));
#3076=DIRECTION('center_axis',(0.866025403784442,0.499999999999995,0.));
#3077=DIRECTION('ref_axis',(-0.499999999999995,0.866025403784442,0.));
#3078=DIRECTION('',(0.,0.,-1.));
#3079=DIRECTION('',(0.499999999999995,-0.866025403784442,0.));
#3080=DIRECTION('',(0.499999999999995,-0.866025403784442,0.));
#3081=DIRECTION('center_axis',(0.866025403784442,0.499999999999995,0.));
#3082=DIRECTION('ref_axis',(-0.499999999999995,0.866025403784442,0.));
#3083=DIRECTION('',(0.499999999999995,-0.866025403784442,0.));
#3084=DIRECTION('',(0.,0.,-1.));
#3085=DIRECTION('',(0.499999999999995,-0.866025403784442,0.));
#3086=DIRECTION('center_axis',(0.,0.,-1.));
#3087=DIRECTION('ref_axis',(-1.,0.,0.));
#3088=DIRECTION('',(-0.866025403784442,-0.499999999999995,0.));
#3089=DIRECTION('center_axis',(0.,0.,-1.));
#3090=DIRECTION('ref_axis',(-1.,0.,0.));
#3091=DIRECTION('',(-0.866025403784442,-0.499999999999995,0.));
#3092=DIRECTION('center_axis',(0.,0.,1.));
#3093=DIRECTION('ref_axis',(1.,0.,0.));
#3094=DIRECTION('center_axis',(0.,0.,1.));
#3095=DIRECTION('ref_axis',(1.,0.,0.));
#3096=DIRECTION('center_axis',(0.499999999999995,-0.866025403784442,0.));
#3097=DIRECTION('ref_axis',(0.866025403784442,0.499999999999995,0.));
#3098=DIRECTION('center_axis',(0.499999999999995,-0.866025403784442,0.));
#3099=DIRECTION('ref_axis',(0.866025403784442,0.499999999999995,0.));
#3100=DIRECTION('center_axis',(0.368362767830729,0.663796275596578,-0.65090965254803));
#3101=DIRECTION('ref_axis',(-7.6388663671058E-18,0.700142154364021,0.714003475959681));
#3725=CARTESIAN_POINT('',(0.,0.,0.));
#3726=CARTESIAN_POINT('Ctrl Pts',(18.8143835621595,-45.3725581651887,-2.29264601963605));
#3727=CARTESIAN_POINT('Ctrl Pts',(18.799421862846,-45.366692611081,-2.29601323464502));
#3728=CARTESIAN_POINT('Ctrl Pts',(18.7845100498018,-45.360314232665,-2.29875605009942));
#3729=CARTESIAN_POINT('Ctrl Pts',(18.7622518217144,-45.3499802606706,-2.30191697923756));
#3730=CARTESIAN_POINT('Ctrl Pts',(18.7548376244511,-45.3464005096126,-2.30281208768347));
#3731=CARTESIAN_POINT('Ctrl Pts',(18.7400559460073,-45.3389851193664,-2.30427767151426));
#3732=CARTESIAN_POINT('Ctrl Pts',(18.7326634287054,-45.3351353187089,-2.3048487962336));
#3733=CARTESIAN_POINT('Ctrl Pts',(18.7107560010767,-45.3232997976908,-2.30605306308975));
#3734=CARTESIAN_POINT('Ctrl Pts',(18.69647386335,-45.3150169340706,-2.30618966865469));
#3735=CARTESIAN_POINT('Ctrl Pts',(18.668502415621,-45.297660633993,-2.30516256178937));
#3736=CARTESIAN_POINT('Ctrl Pts',(18.6548195137261,-45.2885911850942,-2.3039990903213));
#3737=CARTESIAN_POINT('Ctrl Pts',(18.6280626028503,-45.269665384442,-2.3003672370976));
#3738=CARTESIAN_POINT('Ctrl Pts',(18.6150036070141,-45.2598211706463,-2.29790262175487));
#3739=CARTESIAN_POINT('Ctrl Pts',(18.5958424864585,-45.244407875027,-2.29318270097683));
#3740=CARTESIAN_POINT('Ctrl Pts',(18.5895683887268,-45.2391944776938,-2.29144761696805));
#3741=CARTESIAN_POINT('Ctrl Pts',(18.5773056208511,-45.2286717796098,-2.28767708876727));
#3742=CARTESIAN_POINT('Ctrl Pts',(18.571302721882,-45.2233510576313,-2.28563816739681));
#3743=CARTESIAN_POINT('Ctrl Pts',(18.5536922471648,-45.2072288630195,-2.27907242657322));
#3744=CARTESIAN_POINT('Ctrl Pts',(18.5424689819436,-45.1962571521417,-2.27409434987581));
#3745=CARTESIAN_POINT('Ctrl Pts',(18.5210534195265,-45.1738767847226,-2.26294902313096));
#3746=CARTESIAN_POINT('Ctrl Pts',(18.5108563517502,-45.1624608434638,-2.2567766707594));
#3747=CARTESIAN_POINT('Ctrl Pts',(18.4915255994775,-45.1392076266336,-2.24323675136636));
#3748=CARTESIAN_POINT('Ctrl Pts',(18.4823425082748,-45.1272886562345,-2.23580916151862));
#3749=CARTESIAN_POINT('Ctrl Pts',(18.4654779188592,-45.1035758058956,-2.22008460131979));
#3750=CARTESIAN_POINT('Ctrl Pts',(18.4577062314804,-45.0916806335816,-2.21173267647811));
#3751=CARTESIAN_POINT('Ctrl Pts',(18.4435024450096,-45.0678731904181,-2.19410226893954));
#3752=CARTESIAN_POINT('Ctrl Pts',(18.4370613768115,-45.0559500756431,-2.18481745164526));
#3753=CARTESIAN_POINT('Ctrl Pts',(18.4283974556018,-45.0380432871124,-2.17018589369896));
#3754=CARTESIAN_POINT('Ctrl Pts',(18.4256747602959,-45.0320672479267,-2.1651880723044));
#3755=CARTESIAN_POINT('Ctrl Pts',(18.4205692543985,-45.0201143102805,-2.15495946376726));
#3756=CARTESIAN_POINT('Ctrl Pts',(18.4181811783317,-45.0141230761169,-2.14971582230565));
#3757=CARTESIAN_POINT('Ctrl Pts',(18.411557743034,-44.996204520912,-2.13367800718911));
#3758=CARTESIAN_POINT('Ctrl Pts',(18.4079107853335,-44.9844773686462,-2.12271082270486));
#3759=CARTESIAN_POINT('Ctrl Pts',(18.4020639448891,-44.9613631523321,-2.10017046144782));
#3760=CARTESIAN_POINT('Ctrl Pts',(18.3998694271457,-44.9499903424353,-2.08860999048261));
#3761=CARTESIAN_POINT('Ctrl Pts',(18.3969224236575,-44.927612616283,-2.06491243172319));
#3762=CARTESIAN_POINT('Ctrl Pts',(18.3961709968481,-44.9166059372197,-2.05277259205872));
#3763=CARTESIAN_POINT('Ctrl Pts',(18.3961415719036,-44.9003846022915,-2.03412910558187));
#3764=CARTESIAN_POINT('Ctrl Pts',(18.3963173860228,-44.8950134660865,-2.02782648667107));
#3765=CARTESIAN_POINT('Ctrl Pts',(18.3970392739734,-44.8844199010087,-2.01513320991302));
#3766=CARTESIAN_POINT('Ctrl Pts',(18.3975826848578,-44.879219163033,-2.00876936719308));
#3767=CARTESIAN_POINT('Ctrl Pts',(18.3997509614153,-44.8639020731823,-1.98962815132851));
#3768=CARTESIAN_POINT('Ctrl Pts',(18.4019103092124,-44.8540407117655,-1.97676890218923));
#3769=CARTESIAN_POINT('Ctrl Pts',(18.407622325662,-44.835045996909,-1.95090394599962));
#3770=CARTESIAN_POINT('Ctrl Pts',(18.4111751980384,-44.825905164125,-1.93788950367134));
#3771=CARTESIAN_POINT('Ctrl Pts',(18.4196773870788,-44.8083449742005,-1.91169905664016));
#3772=CARTESIAN_POINT('Ctrl Pts',(18.4246337291704,-44.7999153918194,-1.89850633451621));
#3773=CARTESIAN_POINT('Ctrl Pts',(18.4359627695104,-44.7838395187261,-1.87201135519203));
#3774=CARTESIAN_POINT('Ctrl Pts',(18.4422430814637,-44.7763186261024,-1.85891858586588));
#3775=CARTESIAN_POINT('Ctrl Pts',(18.4560163442605,-44.7622376811399,-1.83296819839048));
#3776=CARTESIAN_POINT('Ctrl Pts',(18.4635048906187,-44.7556841943707,-1.82012124842252));
#3777=CARTESIAN_POINT('Ctrl Pts',(18.4796749688842,-44.7435444443489,-1.79468113425342));
#3778=CARTESIAN_POINT('Ctrl Pts',(18.4883628415307,-44.737956512423,-1.78208152867849));
#3779=CARTESIAN_POINT('Ctrl Pts',(18.5069294527721,-44.7277745729134,-1.75716664715693));
#3780=CARTESIAN_POINT('Ctrl Pts',(18.5168839026318,-44.7231591454028,-1.74477273547151));
#3781=CARTESIAN_POINT('Ctrl Pts',(18.5375829891438,-44.7151329976084,-1.72079652319878));
#3782=CARTESIAN_POINT('Ctrl Pts',(18.5483955659724,-44.7116778811927,-1.70911489538877));
#3783=CARTESIAN_POINT('Ctrl Pts',(18.5708927433727,-44.7058864158376,-1.68640778762084));
#3784=CARTESIAN_POINT('Ctrl Pts',(18.5825836040364,-44.703545953535,-1.67537312136182));
#3785=CARTESIAN_POINT('Ctrl Pts',(18.6068588448963,-44.6999847326678,-1.65394839029514));
#3786=CARTESIAN_POINT('Ctrl Pts',(18.619445513792,-44.6987636790236,-1.64355633794861));
#3787=CARTESIAN_POINT('Ctrl Pts',(18.645538711709,-44.6974830389479,-1.6234501769643));
#3788=CARTESIAN_POINT('Ctrl Pts',(18.6588325169338,-44.6974335055609,-1.61389957814289));
#3789=CARTESIAN_POINT('Ctrl Pts',(18.6859142215439,-44.6984777777184,-1.59576518307013));
#3790=CARTESIAN_POINT('Ctrl Pts',(18.6997000237853,-44.6995718128947,-1.58718313777874));
#3791=CARTESIAN_POINT('Ctrl Pts',(18.7277631107646,-44.7028992757828,-1.57098989163726));
#3792=CARTESIAN_POINT('Ctrl Pts',(18.7420482463831,-44.705135147643,-1.56337590956548));
#3793=CARTESIAN_POINT('Ctrl Pts',(18.7710946722565,-44.7107644468085,-1.54915862669876));
#3794=CARTESIAN_POINT('Ctrl Pts',(18.7859459094799,-44.7141859522031,-1.54252376800531));
#3795=CARTESIAN_POINT('Ctrl Pts',(18.8156397942149,-44.7221041428292,-1.53052427124137));
#3796=CARTESIAN_POINT('Ctrl Pts',(18.8305728440077,-44.7266157346991,-1.52511234349085));
#3797=CARTESIAN_POINT('Ctrl Pts',(18.860539209484,-44.7367266946174,-1.5155044665792));
#3798=CARTESIAN_POINT('Ctrl Pts',(18.8756508883745,-44.7423612795317,-1.51129385304441));
#3799=CARTESIAN_POINT('Ctrl Pts',(18.9054576403702,-44.7545267829697,-1.50424311881235));
#3800=CARTESIAN_POINT('Ctrl Pts',(18.9202547119906,-44.7610889823919,-1.50136656793277));
#3801=CARTESIAN_POINT('Ctrl Pts',(18.9495825981467,-44.7751396990536,-1.49691920365679));
#3802=CARTESIAN_POINT('Ctrl Pts',(18.9641293094195,-44.7826350228748,-1.49534501613366));
#3803=CARTESIAN_POINT('Ctrl Pts',(18.9857447788442,-44.7945759268798,-1.49397586706081));
#3804=CARTESIAN_POINT('Ctrl Pts',(18.9929278602255,-44.7986804211822,-1.49368555779672));
#3805=CARTESIAN_POINT('Ctrl Pts',(19.0072126126538,-44.8071190824507,-1.49344249033367));
#3806=CARTESIAN_POINT('Ctrl Pts',(19.0143424710875,-44.8114714840967,-1.49349117220706));
#3807=CARTESIAN_POINT('Ctrl Pts',(19.0354329844958,-44.8247714038735,-1.49415091340346));
#3808=CARTESIAN_POINT('Ctrl Pts',(19.0491062136184,-44.8339600939764,-1.49526534883766));
#3809=CARTESIAN_POINT('Ctrl Pts',(19.0757504934149,-44.8529989681212,-1.49881561860667));
#3810=CARTESIAN_POINT('Ctrl Pts',(19.0887128011736,-44.8628432034342,-1.50125064598544));
#3811=CARTESIAN_POINT('Ctrl Pts',(19.1139155845031,-44.8831828996875,-1.50744605367826));
#3812=CARTESIAN_POINT('Ctrl Pts',(19.1261415989452,-44.8936651252513,-1.51120097784455));
#3813=CARTESIAN_POINT('Ctrl Pts',(19.1439645943469,-44.9099328769387,-1.51787676636393));
#3814=CARTESIAN_POINT('Ctrl Pts',(19.1497815019618,-44.9154129298509,-1.5202634684245));
#3815=CARTESIAN_POINT('Ctrl Pts',(19.1611066834579,-44.9264248357533,-1.52532718281113));
#3816=CARTESIAN_POINT('Ctrl Pts',(19.1666295883308,-44.9319700105026,-1.52800963496645));
#3817=CARTESIAN_POINT('Ctrl Pts',(19.182766450003,-44.9487031839457,-1.53649330236943));
#3818=CARTESIAN_POINT('Ctrl Pts',(19.1929633751574,-44.9600013145975,-1.54273516166076));
#3819=CARTESIAN_POINT('Ctrl Pts',(19.2122406126713,-44.9828745059678,-1.55637255063521));
#3820=CARTESIAN_POINT('Ctrl Pts',(19.2213264422722,-44.9944588868497,-1.56377534127668));
#3821=CARTESIAN_POINT('Ctrl Pts',(19.2383462415657,-45.0178815598089,-1.5797264080401));
#3822=CARTESIAN_POINT('Ctrl Pts',(19.2463304771073,-45.0298136028999,-1.58835146880908));
#3823=CARTESIAN_POINT('Ctrl Pts',(19.2607714831931,-45.0534013484058,-1.60637132681278));
#3824=CARTESIAN_POINT('Ctrl Pts',(19.2673038350586,-45.0651515570016,-1.61582546123857));
#3825=CARTESIAN_POINT('Ctrl Pts',(19.2789889194292,-45.0885216379426,-1.63556445143045));
#3826=CARTESIAN_POINT('Ctrl Pts',(19.2841483413751,-45.1001499111597,-1.64585461771952));
#3827=CARTESIAN_POINT('Ctrl Pts',(19.2930976235061,-45.1232965562804,-1.66727425622956));
#3828=CARTESIAN_POINT('Ctrl Pts',(19.2968886296023,-45.1348186371361,-1.67840737565011));
#3829=CARTESIAN_POINT('Ctrl Pts',(19.3030533575681,-45.1577395162296,-1.70152165051547));
#3830=CARTESIAN_POINT('Ctrl Pts',(19.3053753002664,-45.1689424569227,-1.71330457990983));
#3831=CARTESIAN_POINT('Ctrl Pts',(19.3085649502556,-45.1908773666279,-1.73731958680616));
#3832=CARTESIAN_POINT('Ctrl Pts',(19.3094315307921,-45.2016060723277,-1.74954856369043));
#3833=CARTESIAN_POINT('Ctrl Pts',(19.3097256320476,-45.2225959572621,-1.77444163318775));
#3834=CARTESIAN_POINT('Ctrl Pts',(19.3091504322929,-45.2328640131764,-1.78711583153893));
#3835=CARTESIAN_POINT('Ctrl Pts',(19.3065477416738,-45.2529009468769,-1.81286399012433));
#3836=CARTESIAN_POINT('Ctrl Pts',(19.3044916971078,-45.2627436719468,-1.82604582345194));
#3837=CARTESIAN_POINT('Ctrl Pts',(19.2989881366047,-45.2815256556052,-1.8522784706461));
#3838=CARTESIAN_POINT('Ctrl Pts',(19.2955400517893,-45.290535759037,-1.86541441902233));
#3839=CARTESIAN_POINT('Ctrl Pts',(19.2872838742066,-45.3077809202632,-1.89168343393709));
#3840=CARTESIAN_POINT('Ctrl Pts',(19.2824758531213,-45.3160216986954,-1.90482330786193));
#3841=CARTESIAN_POINT('Ctrl Pts',(19.2714947564013,-45.3317383217991,-1.93111314012225));
#3842=CARTESIAN_POINT('Ctrl Pts',(19.2653276103518,-45.3392082270028,-1.94425196045163));
#3843=CARTESIAN_POINT('Ctrl Pts',(19.2515609423283,-45.3533830770125,-1.97058421507986));
#3844=CARTESIAN_POINT('Ctrl Pts',(19.244064213872,-45.3599773095852,-1.98357519226534));
#3845=CARTESIAN_POINT('Ctrl Pts',(19.2279384887284,-45.3721611568294,-2.00912118369974));
#3846=CARTESIAN_POINT('Ctrl Pts',(19.2192997653202,-45.37776054843,-2.02169452303134));
#3847=CARTESIAN_POINT('Ctrl Pts',(19.2008823814414,-45.3879779405028,-2.04643994358655));
#3848=CARTESIAN_POINT('Ctrl Pts',(19.1910930202263,-45.3925988298126,-2.05862275579914));
#3849=CARTESIAN_POINT('Ctrl Pts',(19.1703915953673,-45.4008287111318,-2.08254175691223));
#3850=CARTESIAN_POINT('Ctrl Pts',(19.1593769020686,-45.4044612308546,-2.09437589174056));
#3851=CARTESIAN_POINT('Ctrl Pts',(19.1365984286433,-45.4105559999369,-2.11715811641161));
#3852=CARTESIAN_POINT('Ctrl Pts',(19.1247946980441,-45.4130446424486,-2.12816493034605));
#3853=CARTESIAN_POINT('Ctrl Pts',(19.1003849579208,-45.4169112106896,-2.14940462118797));
#3854=CARTESIAN_POINT('Ctrl Pts',(19.0877771726989,-45.4182909661987,-2.15964088112869));
#3855=CARTESIAN_POINT('Ctrl Pts',(19.0617491248472,-45.4199293752183,-2.17933956376603));
#3856=CARTESIAN_POINT('Ctrl Pts',(19.0483317526372,-45.4201882850831,-2.1888003047611));
#3857=CARTESIAN_POINT('Ctrl Pts',(19.0206432686844,-45.4195375776723,-2.20692604496228));
#3858=CARTESIAN_POINT('Ctrl Pts',(19.0065974658149,-45.418632682757,-2.21544292771705));
#3859=CARTESIAN_POINT('Ctrl Pts',(18.9781346138199,-45.415695036091,-2.23140600796168));
#3860=CARTESIAN_POINT('Ctrl Pts',(18.9637143613756,-45.4136621054362,-2.23885416694541));
#3861=CARTESIAN_POINT('Ctrl Pts',(18.9344985968864,-45.4084658423515,-2.25268578324637));
#3862=CARTESIAN_POINT('Ctrl Pts',(18.9196997691129,-45.4053010066314,-2.25906973315595));
#3863=CARTESIAN_POINT('Ctrl Pts',(18.8972234079784,-45.399684523811,-2.26782447509019));
#3864=CARTESIAN_POINT('Ctrl Pts',(18.8896670993892,-45.3976611130282,-2.27061057640927));
#3865=CARTESIAN_POINT('Ctrl Pts',(18.8745247920546,-45.3933350465311,-2.27587916719238));
#3866=CARTESIAN_POINT('Ctrl Pts',(18.86697271241,-45.3910428501848,-2.27835075020622));
#3867=CARTESIAN_POINT('Ctrl Pts',(18.8443734352162,-45.3837824914105,-2.28528292905637));
#3868=CARTESIAN_POINT('Ctrl Pts',(18.8293452614729,-45.3784237192965,-2.28927880462709));
#3869=CARTESIAN_POINT('Ctrl Pts',(18.8143835621595,-45.3725581651887,-2.29264601963605));
#3870=CARTESIAN_POINT('Ctrl Pts',(18.6221620196843,-45.62059505756,-1.77871850124803));
#3871=CARTESIAN_POINT('Ctrl Pts',(18.6129193730699,-45.6172932558704,-1.78058192917525));
#3872=CARTESIAN_POINT('Ctrl Pts',(18.6037208544611,-45.6136589591554,-1.78208130646566));
#3873=CARTESIAN_POINT('Ctrl Pts',(18.5900102210826,-45.6077105512134,-1.78377425389336));
#3874=CARTESIAN_POINT('Ctrl Pts',(18.5854465361298,-45.6056405946596,-1.78424599704345));
#3875=CARTESIAN_POINT('Ctrl Pts',(18.576354527559,-45.6013345885701,-1.78500009038837));
#3876=CARTESIAN_POINT('Ctrl Pts',(18.5718108421278,-45.5990902159595,-1.78528264628693));
#3877=CARTESIAN_POINT('Ctrl Pts',(18.5583557915536,-45.592164749705,-1.78583455232009));
#3878=CARTESIAN_POINT('Ctrl Pts',(18.549597268328,-45.5872853986604,-1.78581522368785));
#3879=CARTESIAN_POINT('Ctrl Pts',(18.5324696592232,-45.5770009406535,-1.78502001129054));
#3880=CARTESIAN_POINT('Ctrl Pts',(18.5241044984817,-45.5715981948212,-1.7842443140869));
#3881=CARTESIAN_POINT('Ctrl Pts',(18.5077731763177,-45.560269424572,-1.78193347961354));
#3882=CARTESIAN_POINT('Ctrl Pts',(18.4998161446777,-45.554350730268,-1.78040065085215));
#3883=CARTESIAN_POINT('Ctrl Pts',(18.4881626129628,-45.5450449208074,-1.77750557246982));
#3884=CARTESIAN_POINT('Ctrl Pts',(18.4843505062967,-45.54189107573,-1.77644663525675));
#3885=CARTESIAN_POINT('Ctrl Pts',(18.4769071413954,-45.5355132808845,-1.77415492247898));
#3886=CARTESIAN_POINT('Ctrl Pts',(18.4732672288629,-45.5322824364064,-1.77292001334332));
#3887=CARTESIAN_POINT('Ctrl Pts',(18.4626004022307,-45.5224752605349,-1.7689552464585));
#3888=CARTESIAN_POINT('Ctrl Pts',(18.4558179103171,-45.5157781683263,-1.76596391369291));
#3889=CARTESIAN_POINT('Ctrl Pts',(18.4429084062604,-45.5020723540079,-1.75929249956289));
#3890=CARTESIAN_POINT('Ctrl Pts',(18.4367785698554,-45.4950591040281,-1.75560939899404));
#3891=CARTESIAN_POINT('Ctrl Pts',(18.4251947575442,-45.4807293651287,-1.74755147248085));
#3892=CARTESIAN_POINT('Ctrl Pts',(18.4197116844311,-45.4733619559223,-1.74314118482812));
#3893=CARTESIAN_POINT('Ctrl Pts',(18.4096841967476,-45.4586601759361,-1.73382309642942));
#3894=CARTESIAN_POINT('Ctrl Pts',(18.4050855722086,-45.4512635702888,-1.72888250720206));
#3895=CARTESIAN_POINT('Ctrl Pts',(18.3967294933308,-45.4364159601022,-1.71846981786302));
#3896=CARTESIAN_POINT('Ctrl Pts',(18.3929666633764,-45.4289582747971,-1.71299394688883));
#3897=CARTESIAN_POINT('Ctrl Pts',(18.387949845685,-45.4177241224448,-1.7043764995696));
#3898=CARTESIAN_POINT('Ctrl Pts',(18.3863815973451,-45.4139692966578,-1.70143483928496));
#3899=CARTESIAN_POINT('Ctrl Pts',(18.3834588294126,-45.4064475115089,-1.69541819155667));
#3900=CARTESIAN_POINT('Ctrl Pts',(18.3821013440093,-45.4026715013318,-1.69233565252243));
#3901=CARTESIAN_POINT('Ctrl Pts',(18.3783678140288,-45.3913602280059,-1.68291331926215));
#3902=CARTESIAN_POINT('Ctrl Pts',(18.3763571442371,-45.3839334687444,-1.67647740418325));
#3903=CARTESIAN_POINT('Ctrl Pts',(18.373239274455,-45.3692470015761,-1.66326464104222));
#3904=CARTESIAN_POINT('Ctrl Pts',(18.3721351020341,-45.361996292618,-1.65649525672691));
#3905=CARTESIAN_POINT('Ctrl Pts',(18.3708276406403,-45.3476781657535,-1.64263357999033));
#3906=CARTESIAN_POINT('Ctrl Pts',(18.3706250612,-45.3406095748083,-1.635539689768));
#3907=CARTESIAN_POINT('Ctrl Pts',(18.3710077529534,-45.3301503262564,-1.62465679749559));
#3908=CARTESIAN_POINT('Ctrl Pts',(18.3712517326172,-45.3266799167243,-1.62097960829253));
#3909=CARTESIAN_POINT('Ctrl Pts',(18.3719701704098,-45.3198204005466,-1.61357771003206));
#3910=CARTESIAN_POINT('Ctrl Pts',(18.3724424090973,-45.3164453844991,-1.60986862656259));
#3911=CARTESIAN_POINT('Ctrl Pts',(18.3741925883538,-45.3064826315517,-1.59871817096884));
#3912=CARTESIAN_POINT('Ctrl Pts',(18.3758024868939,-45.300037895571,-1.59123476923353));
#3913=CARTESIAN_POINT('Ctrl Pts',(18.3798873333543,-45.287560207475,-1.57619835335595));
#3914=CARTESIAN_POINT('Ctrl Pts',(18.3823625923558,-45.2815224282728,-1.56864024051346));
#3915=CARTESIAN_POINT('Ctrl Pts',(18.3881814606797,-45.2698526364099,-1.55344639789905));
#3916=CARTESIAN_POINT('Ctrl Pts',(18.3915297734654,-45.2642137421464,-1.54580098849944));
#3917=CARTESIAN_POINT('Ctrl Pts',(18.3991069351451,-45.2533791834234,-1.53046386154549));
#3918=CARTESIAN_POINT('Ctrl Pts',(18.4032741386649,-45.2482681928533,-1.52289338059093));
#3919=CARTESIAN_POINT('Ctrl Pts',(18.4123563475389,-45.2386112685697,-1.50790546647126));
#3920=CARTESIAN_POINT('Ctrl Pts',(18.4172683983267,-45.2340697519755,-1.50049420992322));
#3921=CARTESIAN_POINT('Ctrl Pts',(18.4278282750222,-45.2255558775991,-1.48583573393937));
#3922=CARTESIAN_POINT('Ctrl Pts',(18.4334801703118,-45.2215821677685,-1.47858483274337));
#3923=CARTESIAN_POINT('Ctrl Pts',(18.4455181297567,-45.2142206641317,-1.46426506544444));
#3924=CARTESIAN_POINT('Ctrl Pts',(18.4519528219293,-45.2108157610502,-1.45715123177322));
#3925=CARTESIAN_POINT('Ctrl Pts',(18.4652968721977,-45.2047449038404,-1.44340852007555));
#3926=CARTESIAN_POINT('Ctrl Pts',(18.4722504447086,-45.2020474267363,-1.43672247316454));
#3927=CARTESIAN_POINT('Ctrl Pts',(18.4866860257431,-45.1973329645429,-1.42374529115857));
#3928=CARTESIAN_POINT('Ctrl Pts',(18.4941721105413,-45.1953130577611,-1.41744886968267));
#3929=CARTESIAN_POINT('Ctrl Pts',(18.5096858061187,-45.1919542156582,-1.40524401960937));
#3930=CARTESIAN_POINT('Ctrl Pts',(18.5177148817011,-45.1906149853657,-1.39933446124003));
#3931=CARTESIAN_POINT('Ctrl Pts',(18.5343294229057,-45.1886445172451,-1.38792248147468));
#3932=CARTESIAN_POINT('Ctrl Pts',(18.542779440216,-45.188029106266,-1.38251285316967));
#3933=CARTESIAN_POINT('Ctrl Pts',(18.5599645231716,-45.1875150185148,-1.37226320603098));
#3934=CARTESIAN_POINT('Ctrl Pts',(18.5686982527055,-45.1876165784289,-1.36742418470241));
#3935=CARTESIAN_POINT('Ctrl Pts',(18.5864477638643,-45.1885360827692,-1.35831709053276));
#3936=CARTESIAN_POINT('Ctrl Pts',(18.5954684722606,-45.1893552624518,-1.35404748924571));
#3937=CARTESIAN_POINT('Ctrl Pts',(18.6137800334896,-45.1917248752601,-1.34610113724339));
#3938=CARTESIAN_POINT('Ctrl Pts',(18.6231272825575,-45.1932895780203,-1.34240702291553));
#3939=CARTESIAN_POINT('Ctrl Pts',(18.6417841046389,-45.1971209486494,-1.33575597841215));
#3940=CARTESIAN_POINT('Ctrl Pts',(18.6511507406784,-45.1993932961657,-1.33277254722322));
#3941=CARTESIAN_POINT('Ctrl Pts',(18.6699132468501,-45.204646120538,-1.32751128947911));
#3942=CARTESIAN_POINT('Ctrl Pts',(18.6793578875184,-45.207646105241,-1.32522575676464));
#3943=CARTESIAN_POINT('Ctrl Pts',(18.6979513544394,-45.214255255135,-1.32144333958208));
#3944=CARTESIAN_POINT('Ctrl Pts',(18.7071641468385,-45.2178802413143,-1.31992638960479));
#3945=CARTESIAN_POINT('Ctrl Pts',(18.7253869486455,-45.225754682879,-1.31764408095801));
#3946=CARTESIAN_POINT('Ctrl Pts',(18.7344068621661,-45.2300078746987,-1.316876927761));
#3947=CARTESIAN_POINT('Ctrl Pts',(18.7477801983432,-45.2368600692891,-1.31629654325037));
#3948=CARTESIAN_POINT('Ctrl Pts',(18.752219283311,-45.2392274939513,-1.31619867106209));
#3949=CARTESIAN_POINT('Ctrl Pts',(18.7610367701067,-45.2441187387261,-1.31619676023362));
#3950=CARTESIAN_POINT('Ctrl Pts',(18.7654325107433,-45.2466532619187,-1.3162938241929));
#3951=CARTESIAN_POINT('Ctrl Pts',(18.7784191500246,-45.2544329831877,-1.31687816890436));
#3952=CARTESIAN_POINT('Ctrl Pts',(18.7868169502624,-45.2598527540315,-1.31765275683562));
#3953=CARTESIAN_POINT('Ctrl Pts',(18.8031371766128,-45.2711680622823,-1.31995614213438));
#3954=CARTESIAN_POINT('Ctrl Pts',(18.8110542369534,-45.2770600838242,-1.3214843906258));
#3955=CARTESIAN_POINT('Ctrl Pts',(18.8264003541456,-45.2893146918086,-1.32529693961078));
#3956=CARTESIAN_POINT('Ctrl Pts',(18.8338206659933,-45.2956692062439,-1.32757795725868));
#3957=CARTESIAN_POINT('Ctrl Pts',(18.8445991939612,-45.3055898547247,-1.33159522925254));
#3958=CARTESIAN_POINT('Ctrl Pts',(18.8481102922723,-45.308941341363,-1.3330260675456));
#3959=CARTESIAN_POINT('Ctrl Pts',(18.8549328043703,-45.3156945009062,-1.33605192943852));
#3960=CARTESIAN_POINT('Ctrl Pts',(18.8582530677542,-45.3191042958294,-1.33765022769154));
#3961=CARTESIAN_POINT('Ctrl Pts',(18.867933585062,-45.3294204870494,-1.34269225948157));
#3962=CARTESIAN_POINT('Ctrl Pts',(18.8740225584048,-45.336421260905,-1.34638576214841));
#3963=CARTESIAN_POINT('Ctrl Pts',(18.8854757967299,-45.3506622005078,-1.35442702575445));
#3964=CARTESIAN_POINT('Ctrl Pts',(18.8908432353629,-45.3579082824918,-1.35877902402508));
#3965=CARTESIAN_POINT('Ctrl Pts',(18.9008330792294,-45.3726243827529,-1.36813301959756));
#3966=CARTESIAN_POINT('Ctrl Pts',(18.9054840795676,-45.380154146016,-1.37317976216689));
#3967=CARTESIAN_POINT('Ctrl Pts',(18.9138227526446,-45.3951016039498,-1.38370412631569));
#3968=CARTESIAN_POINT('Ctrl Pts',(18.9175551433971,-45.4025783442055,-1.38921665563984));
#3969=CARTESIAN_POINT('Ctrl Pts',(18.9241472981129,-45.4175069410417,-1.40071017489184));
#3970=CARTESIAN_POINT('Ctrl Pts',(18.9270110154327,-45.4249640522584,-1.40669428620247));
#3971=CARTESIAN_POINT('Ctrl Pts',(18.9318734081378,-45.4398636906155,-1.41913718051563));
#3972=CARTESIAN_POINT('Ctrl Pts',(18.9338726776514,-45.4473086206934,-1.42559807779935));
#3973=CARTESIAN_POINT('Ctrl Pts',(18.9369783416384,-45.4621742438128,-1.4390004513004));
#3974=CARTESIAN_POINT('Ctrl Pts',(18.9380587854086,-45.4694678481601,-1.44582700875946));
#3975=CARTESIAN_POINT('Ctrl Pts',(18.9393173410065,-45.4838003767252,-1.45973104908589));
#3976=CARTESIAN_POINT('Ctrl Pts',(18.9394948496878,-45.4908371992824,-1.46680673001694));
#3977=CARTESIAN_POINT('Ctrl Pts',(18.9389586363646,-45.504655487356,-1.4812020445518));
#3978=CARTESIAN_POINT('Ctrl Pts',(18.9382429617193,-45.5114415845077,-1.48852750652597));
#3979=CARTESIAN_POINT('Ctrl Pts',(18.935914549752,-45.5247359862846,-1.5034028039268));
#3980=CARTESIAN_POINT('Ctrl Pts',(18.9342813020382,-45.5312939444273,-1.51101488314489));
#3981=CARTESIAN_POINT('Ctrl Pts',(18.9301711295785,-45.543861814362,-1.52615759875804));
#3982=CARTESIAN_POINT('Ctrl Pts',(18.9276914024776,-45.5499184342165,-1.53373745384419));
#3983=CARTESIAN_POINT('Ctrl Pts',(18.9219044584414,-45.5615659591846,-1.5488905221349));
#3984=CARTESIAN_POINT('Ctrl Pts',(18.9185970863043,-45.5671606360396,-1.55646766958521));
#3985=CARTESIAN_POINT('Ctrl Pts',(18.9111518540018,-45.5778903308794,-1.5716231951062));
#3986=CARTESIAN_POINT('Ctrl Pts',(18.9070179238834,-45.5830212371186,-1.57919515593537));
#3987=CARTESIAN_POINT('Ctrl Pts',(18.8978775137544,-45.5928252580521,-1.59436601615716));
#3988=CARTESIAN_POINT('Ctrl Pts',(18.8929394538017,-45.5974219543871,-1.60184826399308));
#3989=CARTESIAN_POINT('Ctrl Pts',(18.8823875119263,-45.6059897116602,-1.61655719916668));
#3990=CARTESIAN_POINT('Ctrl Pts',(18.8767671790069,-45.6099675442075,-1.62379444292518));
#3991=CARTESIAN_POINT('Ctrl Pts',(18.8648446796018,-45.6173136869872,-1.63803320411293));
#3992=CARTESIAN_POINT('Ctrl Pts',(18.8585356910874,-45.620684256901,-1.645040886683));
#3993=CARTESIAN_POINT('Ctrl Pts',(18.8452471260023,-45.6267961002234,-1.65879399575824));
#3994=CARTESIAN_POINT('Ctrl Pts',(18.8382022586574,-45.629556299998,-1.66559567268411));
#3995=CARTESIAN_POINT('Ctrl Pts',(18.8236812226873,-45.6343318803847,-1.67868354354709));
#3996=CARTESIAN_POINT('Ctrl Pts',(18.816179049323,-45.6363659793353,-1.68500354300762));
#3997=CARTESIAN_POINT('Ctrl Pts',(18.8007069179842,-45.6397318406192,-1.69719202919393));
#3998=CARTESIAN_POINT('Ctrl Pts',(18.7927357842832,-45.6410648637206,-1.70306246701553));
#3999=CARTESIAN_POINT('Ctrl Pts',(18.7763184849427,-45.6430238072,-1.7143510708677));
#4000=CARTESIAN_POINT('Ctrl Pts',(18.7678741313109,-45.643649793127,-1.7197682782934));
#4001=CARTESIAN_POINT('Ctrl Pts',(18.750484658679,-45.6441668837513,-1.73013665595371));
#4002=CARTESIAN_POINT('Ctrl Pts',(18.7416810490484,-45.6440534227969,-1.7350030871688));
#4003=CARTESIAN_POINT('Ctrl Pts',(18.7238738472453,-45.6431037361945,-1.74411204981961));
#4004=CARTESIAN_POINT('Ctrl Pts',(18.7148682493225,-45.6422674984819,-1.74835570404536));
#4005=CARTESIAN_POINT('Ctrl Pts',(18.6966533086483,-45.6398726569234,-1.75622164832084));
#4006=CARTESIAN_POINT('Ctrl Pts',(18.6874419268025,-45.6383131841139,-1.75984420616735));
#4007=CARTESIAN_POINT('Ctrl Pts',(18.6734737700129,-45.6354195819173,-1.76479817562067));
#4008=CARTESIAN_POINT('Ctrl Pts',(18.6687815047508,-45.6343591081953,-1.76637215337371));
#4009=CARTESIAN_POINT('Ctrl Pts',(18.6593857582353,-45.6320583062489,-1.76934304099513));
#4010=CARTESIAN_POINT('Ctrl Pts',(18.6547033024031,-45.6308236309591,-1.77073381700843));
#4011=CARTESIAN_POINT('Ctrl Pts',(18.6407016991349,-45.6268695302727,-1.77462522039306));
#4012=CARTESIAN_POINT('Ctrl Pts',(18.6314046662986,-45.6238968592495,-1.77685507332082));
#4013=CARTESIAN_POINT('Ctrl Pts',(18.6221620196843,-45.62059505756,-1.77871850124803));
#4014=CARTESIAN_POINT('',(18.8905539268402,-44.7484447038542,-1.50776822046474));
#4015=CARTESIAN_POINT('',(18.8998729391632,-45.4003277760596,-2.26677057350411));
#4016=CARTESIAN_POINT('Ctrl Pts',(18.8905539268402,-44.7484447038542,-1.50776822046474));
#4017=CARTESIAN_POINT('Ctrl Pts',(18.9031610996921,-44.7535924051018,-1.50478510512969));
#4018=CARTESIAN_POINT('Ctrl Pts',(18.9153195318725,-44.7589335970676,-1.50235806754206));
#4019=CARTESIAN_POINT('Ctrl Pts',(18.9268587021024,-44.7643102161833,-1.50042690153781));
#4020=CARTESIAN_POINT('Ctrl Pts',(18.9290522874274,-44.7653323063818,-1.50005978871058));
#4021=CARTESIAN_POINT('Ctrl Pts',(18.931223536412,-44.7663556008484,-1.49971047085396));
#4022=CARTESIAN_POINT('Ctrl Pts',(18.9333713376819,-44.7673789131467,-1.49937836590513));
#4023=CARTESIAN_POINT('Ctrl Pts',(18.9338890838472,-44.767625591471,-1.49929830912049));
#4024=CARTESIAN_POINT('Ctrl Pts',(18.9344042911217,-44.7678717143732,-1.49921943230172));
#4025=CARTESIAN_POINT('Ctrl Pts',(18.9349171923153,-44.7681173760609,-1.49914167917656));
#4026=CARTESIAN_POINT('Ctrl Pts',(18.940590051698,-44.7708344767955,-1.49828170351057));
#4027=CARTESIAN_POINT('Ctrl Pts',(18.9459838062476,-44.7734936441197,-1.4975551963276));
#4028=CARTESIAN_POINT('Ctrl Pts',(18.9514090992294,-44.7762397711827,-1.49691005297651));
#4029=CARTESIAN_POINT('Ctrl Pts',(18.9567181151493,-44.7789270421458,-1.49627873659727));
#4030=CARTESIAN_POINT('Ctrl Pts',(18.9620573977875,-44.7816976275958,-1.49572532328795));
#4031=CARTESIAN_POINT('Ctrl Pts',(18.9677105039338,-44.7847152231857,-1.49524009137691));
#4032=CARTESIAN_POINT('Ctrl Pts',(18.9693228115803,-44.7855758637465,-1.49510169965027));
#4033=CARTESIAN_POINT('Ctrl Pts',(18.9709605941978,-44.7864567764315,-1.4949691090493));
#4034=CARTESIAN_POINT('Ctrl Pts',(18.9726302937406,-44.7873622109845,-1.49484274021276));
#4035=CARTESIAN_POINT('Ctrl Pts',(18.9746133338402,-44.7884375619567,-1.49469265664155));
#4036=CARTESIAN_POINT('Ctrl Pts',(18.9765824952973,-44.7895155076103,-1.4945558653122));
#4037=CARTESIAN_POINT('Ctrl Pts',(18.9785391615588,-44.7905964953401,-1.49443190148112));
#4038=CARTESIAN_POINT('Ctrl Pts',(18.9858604740922,-44.7946412571732,-1.49396806256899));
#4039=CARTESIAN_POINT('Ctrl Pts',(18.9930191605462,-44.7987358342693,-1.49368354377148));
#4040=CARTESIAN_POINT('Ctrl Pts',(19.0000696572879,-44.8029007956634,-1.49356360210869));
#4041=CARTESIAN_POINT('Ctrl Pts',(19.0072585778343,-44.8071475285728,-1.49344130560738));
#4042=CARTESIAN_POINT('Ctrl Pts',(19.0143634250414,-44.8114857800962,-1.49349151807229));
#4043=CARTESIAN_POINT('Ctrl Pts',(19.0213722794606,-44.8159054154637,-1.49371083042691));
#4044=CARTESIAN_POINT('Ctrl Pts',(19.0306063557352,-44.8217282286723,-1.49399977165603));
#4045=CARTESIAN_POINT('Ctrl Pts',(19.0396805192462,-44.8276914801336,-1.49457633549814));
#4046=CARTESIAN_POINT('Ctrl Pts',(19.0487598877559,-44.8339140289199,-1.49546367796603));
#4047=CARTESIAN_POINT('Ctrl Pts',(19.0498152273431,-44.8346373063219,-1.49556681813848));
#4048=CARTESIAN_POINT('Ctrl Pts',(19.0508706124117,-44.8353641103557,-1.49567420382705));
#4049=CARTESIAN_POINT('Ctrl Pts',(19.0519262829499,-44.8360946464113,-1.49578590842529));
#4050=CARTESIAN_POINT('Ctrl Pts',(19.0554574361024,-44.8385382446765,-1.49615955344986));
#4051=CARTESIAN_POINT('Ctrl Pts',(19.0589574262949,-44.8409997673555,-1.49657789688526));
#4052=CARTESIAN_POINT('Ctrl Pts',(19.0624281525586,-44.8434798481551,-1.49704034979883));
#4053=CARTESIAN_POINT('Ctrl Pts',(19.0758119232263,-44.8530435043288,-1.49882365486802));
#4054=CARTESIAN_POINT('Ctrl Pts',(19.0887526635036,-44.8628762409233,-1.50126029358194));
#4055=CARTESIAN_POINT('Ctrl Pts',(19.1013137349989,-44.8730137161139,-1.50434805664924));
#4056=CARTESIAN_POINT('Ctrl Pts',(19.113918973379,-44.8831868364083,-1.5074466768218));
#4057=CARTESIAN_POINT('Ctrl Pts',(19.1261274095114,-44.8936535753615,-1.51119550771856));
#4058=CARTESIAN_POINT('Ctrl Pts',(19.1380229461204,-44.9045111632162,-1.51565109795051));
#4059=CARTESIAN_POINT('Ctrl Pts',(19.143954111713,-44.9099248031066,-1.51787267435748));
#4060=CARTESIAN_POINT('Ctrl Pts',(19.1497694272033,-44.9154027344374,-1.52025795176899));
#4061=CARTESIAN_POINT('Ctrl Pts',(19.1554434156545,-44.9209197547308,-1.5227949062348));
#4062=CARTESIAN_POINT('Ctrl Pts',(19.1610906834191,-44.9264107935526,-1.52531991334367));
#4063=CARTESIAN_POINT('Ctrl Pts',(19.1666124570964,-44.9319537629785,-1.52800056793989));
#4064=CARTESIAN_POINT('Ctrl Pts',(19.1720079090184,-44.9375485200328,-1.53083713359701));
#4065=CARTESIAN_POINT('Ctrl Pts',(19.1774114710702,-44.9431516868009,-1.53367796301484));
#4066=CARTESIAN_POINT('Ctrl Pts',(19.1826920566001,-44.9488099277027,-1.53667625408543));
#4067=CARTESIAN_POINT('Ctrl Pts',(19.1878522647798,-44.9545295630061,-1.53983751083408));
#4068=CARTESIAN_POINT('Ctrl Pts',(19.1929448601249,-44.9601742554499,-1.54295734647669));
#4069=CARTESIAN_POINT('Ctrl Pts',(19.1978550853105,-44.965806463315,-1.54619576434285));
#4070=CARTESIAN_POINT('Ctrl Pts',(19.2026016057627,-44.9714383576466,-1.54955361672181));
#4071=CARTESIAN_POINT('Ctrl Pts',(19.2116168981582,-44.9821352828257,-1.55593134569646));
#4072=CARTESIAN_POINT('Ctrl Pts',(19.2200484428352,-44.9928385763987,-1.56274402992607));
#4073=CARTESIAN_POINT('Ctrl Pts',(19.227975850479,-45.0036254988957,-1.57002490172002));
#4074=CARTESIAN_POINT('Ctrl Pts',(19.2285989697718,-45.0044733850926,-1.57059720125185));
#4075=CARTESIAN_POINT('Ctrl Pts',(19.2292189565125,-45.0053217930469,-1.5711724126414));
#4076=CARTESIAN_POINT('Ctrl Pts',(19.2298358401891,-45.0061707627611,-1.57175056175926));
#4077=CARTESIAN_POINT('Ctrl Pts',(19.2375792501632,-45.0168274243037,-1.57900775759058));
#4078=CARTESIAN_POINT('Ctrl Pts',(19.244878754062,-45.0276503346359,-1.58678907892552));
#4079=CARTESIAN_POINT('Ctrl Pts',(19.2516100858949,-45.0384653157022,-1.59497152212934));
#4080=CARTESIAN_POINT('Ctrl Pts',(19.2522622252624,-45.039513083824,-1.59576424687792));
#4081=CARTESIAN_POINT('Ctrl Pts',(19.2529089949182,-45.0405607690862,-1.59656075297211));
#4082=CARTESIAN_POINT('Ctrl Pts',(19.2535502558879,-45.0416082043859,-1.59736093675765));
#4083=CARTESIAN_POINT('Ctrl Pts',(19.260249072408,-45.0525500474423,-1.60571991167469));
#4084=CARTESIAN_POINT('Ctrl Pts',(19.2664155159093,-45.0635464214966,-1.61452921889829));
#4085=CARTESIAN_POINT('Ctrl Pts',(19.2720575854048,-45.0746758327777,-1.6238743793119));
#4086=CARTESIAN_POINT('Ctrl Pts',(19.272422529821,-45.0753957134007,-1.62447884973092));
#4087=CARTESIAN_POINT('Ctrl Pts',(19.2727852644496,-45.0761161483359,-1.62508557053341));
#4088=CARTESIAN_POINT('Ctrl Pts',(19.2731457848041,-45.0768371578105,-1.62569456832308));
#4089=CARTESIAN_POINT('Ctrl Pts',(19.2746602560061,-45.0798659690052,-1.62825284167146));
#4090=CARTESIAN_POINT('Ctrl Pts',(19.2761361224734,-45.0829054847382,-1.63085164053693));
#4091=CARTESIAN_POINT('Ctrl Pts',(19.277572904716,-45.0859576117991,-1.63349352538219));
#4092=CARTESIAN_POINT('Ctrl Pts',(19.2810109144354,-45.0932609053601,-1.6398151693354));
#4093=CARTESIAN_POINT('Ctrl Pts',(19.2840733991544,-45.1003073233589,-1.64609582363185));
#4094=CARTESIAN_POINT('Ctrl Pts',(19.2868600061465,-45.1072502054313,-1.65244793958539));
#4095=CARTESIAN_POINT('Ctrl Pts',(19.2874602276128,-45.1087456681463,-1.65381615417853));
#4096=CARTESIAN_POINT('Ctrl Pts',(19.2880474864276,-45.1102363136529,-1.65518778497339));
#4097=CARTESIAN_POINT('Ctrl Pts',(19.288622513537,-45.1117236523756,-1.65656411889582));
#4098=CARTESIAN_POINT('Ctrl Pts',(19.2912948888323,-45.118635895631,-1.66296047954142));
#4099=CARTESIAN_POINT('Ctrl Pts',(19.2937068903777,-45.1254783069726,-1.66945763476478));
#4100=CARTESIAN_POINT('Ctrl Pts',(19.2959010250622,-45.1323978340472,-1.6762010109593));
#4101=CARTESIAN_POINT('Ctrl Pts',(19.2973532075745,-45.1369775056062,-1.68066409750223));
#4102=CARTESIAN_POINT('Ctrl Pts',(19.2987091190889,-45.1415908971441,-1.68523556157793));
#4103=CARTESIAN_POINT('Ctrl Pts',(19.2999702919787,-45.1462796703514,-1.68996401717864));
#4104=CARTESIAN_POINT('Ctrl Pts',(19.3003859764899,-45.147825097164,-1.69152252336869));
#4105=CARTESIAN_POINT('Ctrl Pts',(19.3007903536338,-45.1493751466532,-1.69309452547372));
#4106=CARTESIAN_POINT('Ctrl Pts',(19.3011833659943,-45.1509312276157,-1.69468174294826));
#4107=CARTESIAN_POINT('Ctrl Pts',(19.3028171351878,-45.1573999227367,-1.70127987388149));
#4108=CARTESIAN_POINT('Ctrl Pts',(19.3041469608748,-45.1635341686414,-1.70769026657886));
#4109=CARTESIAN_POINT('Ctrl Pts',(19.3052506878946,-45.1695067470371,-1.71406487112993));
#4110=CARTESIAN_POINT('Ctrl Pts',(19.3058999584912,-45.173020133471,-1.717814750607));
#4111=CARTESIAN_POINT('Ctrl Pts',(19.3064700252133,-45.176477240148,-1.72155252468992));
#4112=CARTESIAN_POINT('Ctrl Pts',(19.3069691692539,-45.1799106820285,-1.7253113759015));
#4113=CARTESIAN_POINT('Ctrl Pts',(19.3078288407013,-45.1858240691695,-1.73178521270814));
#4114=CARTESIAN_POINT('Ctrl Pts',(19.3084803198211,-45.1916671269783,-1.73831990863014));
#4115=CARTESIAN_POINT('Ctrl Pts',(19.3089258684228,-45.1975919843597,-1.74509559154831));
#4116=CARTESIAN_POINT('Ctrl Pts',(19.3092823464461,-45.2023323907711,-1.75051673313525));
#4117=CARTESIAN_POINT('Ctrl Pts',(19.3095062324181,-45.2071249057774,-1.75609237576449));
#4118=CARTESIAN_POINT('Ctrl Pts',(19.3095767014592,-45.2120403257133,-1.76192141946182));
#4119=CARTESIAN_POINT('Ctrl Pts',(19.3095769951772,-45.2120608133933,-1.76194571516467));
#4120=CARTESIAN_POINT('Ctrl Pts',(19.3095772861822,-45.2120813019672,-1.7619700138185));
#4121=CARTESIAN_POINT('Ctrl Pts',(19.3095775744728,-45.2121017914341,-1.76199431542308));
#4122=CARTESIAN_POINT('Ctrl Pts',(19.3096500706704,-45.2172542611667,-1.76810542035325));
#4123=CARTESIAN_POINT('Ctrl Pts',(19.3095501662677,-45.2224648859554,-1.77440566660266));
#4124=CARTESIAN_POINT('Ctrl Pts',(19.3092543196308,-45.2277160746578,-1.7808883526774));
#4125=CARTESIAN_POINT('Ctrl Pts',(19.3091160779735,-45.2301698224415,-1.78391754806325));
#4126=CARTESIAN_POINT('Ctrl Pts',(19.3089694464571,-45.2321010041524,-1.78632752666564));
#4127=CARTESIAN_POINT('Ctrl Pts',(19.3088187707449,-45.2338621207923,-1.78853667120843));
#4128=CARTESIAN_POINT('Ctrl Pts',(19.3086457077997,-45.2358849022229,-1.79107404803929));
#4129=CARTESIAN_POINT('Ctrl Pts',(19.3084671105678,-45.2376833156781,-1.79334660829998));
#4130=CARTESIAN_POINT('Ctrl Pts',(19.3082279498134,-45.2397710718633,-1.79600629485637));
#4131=CARTESIAN_POINT('Ctrl Pts',(19.3081111756757,-45.240790452861,-1.79730493018301));
#4132=CARTESIAN_POINT('Ctrl Pts',(19.3079846031041,-45.2418281112385,-1.79863218212924));
#4133=CARTESIAN_POINT('Ctrl Pts',(19.3078472833032,-45.2428838188181,-1.79998843184757));
#4134=CARTESIAN_POINT('Ctrl Pts',(19.3072761515731,-45.2472746502375,-1.80562925890165));
#4135=CARTESIAN_POINT('Ctrl Pts',(19.306514269498,-45.2519944004966,-1.81179500409166));
#4136=CARTESIAN_POINT('Ctrl Pts',(19.3054899970412,-45.2569968413792,-1.81847964198376));
#4137=CARTESIAN_POINT('Ctrl Pts',(19.3048735218124,-45.2600076427211,-1.82250290127023));
#4138=CARTESIAN_POINT('Ctrl Pts',(19.3041618274159,-45.2631203030561,-1.82671358764469));
#4139=CARTESIAN_POINT('Ctrl Pts',(19.3033379472344,-45.2663183805069,-1.83110364640795));
#4140=CARTESIAN_POINT('Ctrl Pts',(19.3028516227151,-45.2682061592321,-1.83369503441009));
#4141=CARTESIAN_POINT('Ctrl Pts',(19.3023186401626,-45.2701521550093,-1.83638798495598));
#4142=CARTESIAN_POINT('Ctrl Pts',(19.3017373109881,-45.272136535723,-1.83915988629776));
#4143=CARTESIAN_POINT('Ctrl Pts',(19.3004282344149,-45.2766050991776,-1.8454018422643));
#4144=CARTESIAN_POINT('Ctrl Pts',(19.2988710018605,-45.2812824487729,-1.85206311467574));
#4145=CARTESIAN_POINT('Ctrl Pts',(19.2970708305084,-45.2859874631502,-1.85892298274384));
#4146=CARTESIAN_POINT('Ctrl Pts',(19.2955249874694,-45.290027752823,-1.86481368825293));
#4147=CARTESIAN_POINT('Ctrl Pts',(19.2938005148776,-45.2940886659696,-1.87085074760323));
#4148=CARTESIAN_POINT('Ctrl Pts',(19.2919279277246,-45.2980702360208,-1.87689341384836));
#4149=CARTESIAN_POINT('Ctrl Pts',(19.291756070827,-45.2984356450622,-1.87744798022584));
#4150=CARTESIAN_POINT('Ctrl Pts',(19.2915838951129,-45.2987984610612,-1.87799965670778));
#4151=CARTESIAN_POINT('Ctrl Pts',(19.2914114387417,-45.2991587065637,-1.87854844423543));
#4152=CARTESIAN_POINT('Ctrl Pts',(19.2882717859622,-45.30571715254,-1.88853939020666));
#4153=CARTESIAN_POINT('Ctrl Pts',(19.2850429685109,-45.3114291131316,-1.89757671877641));
#4154=CARTESIAN_POINT('Ctrl Pts',(19.2819223052065,-45.316417591916,-1.90567353726888));
#4155=CARTESIAN_POINT('Ctrl Pts',(19.2802373747464,-45.3191110064351,-1.91004522840538));
#4156=CARTESIAN_POINT('Ctrl Pts',(19.2785831810204,-45.3215930602608,-1.91414275007192));
#4157=CARTESIAN_POINT('Ctrl Pts',(19.2769853047611,-45.3238800102474,-1.91796822399195));
#4158=CARTESIAN_POINT('Ctrl Pts',(19.276955266244,-45.3239230026794,-1.91804013917522));
#4159=CARTESIAN_POINT('Ctrl Pts',(19.2769252476959,-45.3239659259204,-1.91811195788365));
#4160=CARTESIAN_POINT('Ctrl Pts',(19.2768952492667,-45.3240087800738,-1.91818368013959));
#4161=CARTESIAN_POINT('Ctrl Pts',(19.2745234678546,-45.3273969802972,-1.9238542941712));
#4162=CARTESIAN_POINT('Ctrl Pts',(19.272276852796,-45.3303569483095,-1.92892674082638));
#4163=CARTESIAN_POINT('Ctrl Pts',(19.2702183165253,-45.3329374402795,-1.93341671392623));
#4164=CARTESIAN_POINT('Ctrl Pts',(19.26918904839,-45.3342276862644,-1.93566170047616));
#4165=CARTESIAN_POINT('Ctrl Pts',(19.2682683746316,-45.3353511621537,-1.9376329604304));
#4166=CARTESIAN_POINT('Ctrl Pts',(19.2671920722735,-45.3366292732086,-1.93989520389112));
#4167=CARTESIAN_POINT('Ctrl Pts',(19.2662154445237,-45.3377890204804,-1.94194794466969));
#4168=CARTESIAN_POINT('Ctrl Pts',(19.2651113457867,-45.3390764142967,-1.94424020849365));
#4169=CARTESIAN_POINT('Ctrl Pts',(19.2636480525984,-45.3407128473262,-1.94719472898812));
#4170=CARTESIAN_POINT('Ctrl Pts',(19.2634987089253,-45.3408798616479,-1.94749626728975));
#4171=CARTESIAN_POINT('Ctrl Pts',(19.2633455833603,-45.341050489925,-1.94780470520987));
#4172=CARTESIAN_POINT('Ctrl Pts',(19.2631883989319,-45.3412249511355,-1.94812049329096));
#4173=CARTESIAN_POINT('Ctrl Pts',(19.2616260730571,-45.3429589986225,-1.95125925133951));
#4174=CARTESIAN_POINT('Ctrl Pts',(19.260044246205,-45.3446482119081,-1.95435747676277));
#4175=CARTESIAN_POINT('Ctrl Pts',(19.2584442081375,-45.3462956982991,-1.95741801675829));
#4176=CARTESIAN_POINT('Ctrl Pts',(19.2530911545275,-45.3518074940197,-1.96765729481361));
#4177=CARTESIAN_POINT('Ctrl Pts',(19.2475997168375,-45.356787186144,-1.9773523720224));
#4178=CARTESIAN_POINT('Ctrl Pts',(19.2420166250089,-45.3613450400677,-1.98660396903331));
#4179=CARTESIAN_POINT('Ctrl Pts',(19.2400197366427,-45.3629752345467,-1.98991296107686));
#4180=CARTESIAN_POINT('Ctrl Pts',(19.2380131049024,-45.3645492458353,-1.9931612156242));
#4181=CARTESIAN_POINT('Ctrl Pts',(19.2360013513002,-45.3660692332073,-1.99634818798254));
#4182=CARTESIAN_POINT('Ctrl Pts',(19.2343601682657,-45.3673092347089,-1.99894811123359));
#4183=CARTESIAN_POINT('Ctrl Pts',(19.2327151668666,-45.3685136887886,-2.00150801558279));
#4184=CARTESIAN_POINT('Ctrl Pts',(19.2310684958453,-45.3696838352387,-2.00402793563221));
#4185=CARTESIAN_POINT('Ctrl Pts',(19.2291441073201,-45.3710513314613,-2.00697285004734));
#4186=CARTESIAN_POINT('Ctrl Pts',(19.227397030422,-45.3722491451667,-2.00959402269974));
#4187=CARTESIAN_POINT('Ctrl Pts',(19.2255353703308,-45.3734861835637,-2.01233998107606));
#4188=CARTESIAN_POINT('Ctrl Pts',(19.2238513499697,-45.3746051836745,-2.01482391992113));
#4189=CARTESIAN_POINT('Ctrl Pts',(19.2220734552544,-45.3757561868767,-2.01740993160128));
#4190=CARTESIAN_POINT('Ctrl Pts',(19.2199591852644,-45.3770711300371,-2.02042077054629));
#4191=CARTESIAN_POINT('Ctrl Pts',(19.2167080362679,-45.379093140545,-2.02505058890496));
#4192=CARTESIAN_POINT('Ctrl Pts',(19.213416289607,-45.3810245230521,-2.02959939975511));
#4193=CARTESIAN_POINT('Ctrl Pts',(19.2100910410519,-45.3828692664555,-2.03406719489437));
#4194=CARTESIAN_POINT('Ctrl Pts',(19.2043102415861,-45.3860762723393,-2.04183426172472));
#4195=CARTESIAN_POINT('Ctrl Pts',(19.198424016323,-45.3890224338998,-2.0493605201506));
#4196=CARTESIAN_POINT('Ctrl Pts',(19.192473591163,-45.3917248373075,-2.05663869990211));
#4197=CARTESIAN_POINT('Ctrl Pts',(19.1886352797465,-45.3934680179328,-2.06133347711209));
#4198=CARTESIAN_POINT('Ctrl Pts',(19.1847250305082,-45.3951304340046,-2.06598050218204));
#4199=CARTESIAN_POINT('Ctrl Pts',(19.1807423013201,-45.3967137749435,-2.07058224811008));
#4200=CARTESIAN_POINT('Ctrl Pts',(19.1703387758504,-45.4008497146488,-2.08260274428377));
#4201=CARTESIAN_POINT('Ctrl Pts',(19.159340113541,-45.4044710910164,-2.09441259586237));
#4202=CARTESIAN_POINT('Ctrl Pts',(19.1479876051885,-45.4075086579881,-2.10576692178429));
#4203=CARTESIAN_POINT('Ctrl Pts',(19.1366043896562,-45.4105544412158,-2.11715195980231));
#4204=CARTESIAN_POINT('Ctrl Pts',(19.1248241373798,-45.4130400365554,-2.12813908010357));
#4205=CARTESIAN_POINT('Ctrl Pts',(19.1125897171975,-45.4149780078223,-2.13878461269783));
#4206=CARTESIAN_POINT('Ctrl Pts',(19.1004590408702,-45.4168995457309,-2.14933987468066));
#4207=CARTESIAN_POINT('Ctrl Pts',(19.0878801520033,-45.4182845655764,-2.15956267184218));
#4208=CARTESIAN_POINT('Ctrl Pts',(19.0747630524034,-45.4191102447313,-2.16949006944939));
#4209=CARTESIAN_POINT('Ctrl Pts',(19.0700168171052,-45.4194090049503,-2.1730821566013));
#4210=CARTESIAN_POINT('Ctrl Pts',(19.0652003300979,-45.4196343284435,-2.17663517975666));
#4211=CARTESIAN_POINT('Ctrl Pts',(19.060307729625,-45.4197834514901,-2.18015001824002));
#4212=CARTESIAN_POINT('Ctrl Pts',(19.0517437089387,-45.4200444768615,-2.18630240073015));
#4213=CARTESIAN_POINT('Ctrl Pts',(19.0431772022301,-45.4200671915454,-2.19217450958827));
#4214=CARTESIAN_POINT('Ctrl Pts',(19.0344874410032,-45.419862988065,-2.19786305520717));
#4215=CARTESIAN_POINT('Ctrl Pts',(19.0250894389292,-45.4196421414063,-2.20401523386074));
#4216=CARTESIAN_POINT('Ctrl Pts',(19.0156502563949,-45.4191585088715,-2.20988554243695));
#4217=CARTESIAN_POINT('Ctrl Pts',(19.006007375568,-45.4184031647075,-2.21557544213857));
#4218=CARTESIAN_POINT('Ctrl Pts',(19.0015104970313,-45.4180509161399,-2.21822888028673));
#4219=CARTESIAN_POINT('Ctrl Pts',(18.9969691419846,-45.4176390560957,-2.22084259167287));
#4220=CARTESIAN_POINT('Ctrl Pts',(18.9923659355898,-45.4171639503319,-2.22342427356174));
#4221=CARTESIAN_POINT('Ctrl Pts',(18.9888660975559,-45.4168027253336,-2.22538713763762));
#4222=CARTESIAN_POINT('Ctrl Pts',(18.9853303025957,-45.4164048969542,-2.22733157337029));
#4223=CARTESIAN_POINT('Ctrl Pts',(18.9817504658063,-45.4159679276941,-2.22926016950443));
#4224=CARTESIAN_POINT('Ctrl Pts',(18.9708305376768,-45.414634997397,-2.23514315591277));
#4225=CARTESIAN_POINT('Ctrl Pts',(18.9599302006986,-45.4129890646533,-2.24064569461223));
#4226=CARTESIAN_POINT('Ctrl Pts',(18.9491064785268,-45.411063974465,-2.24576997387064));
#4227=CARTESIAN_POINT('Ctrl Pts',(18.9461921080148,-45.4105456291131,-2.24714972550591));
#4228=CARTESIAN_POINT('Ctrl Pts',(18.9432831789363,-45.4100070429297,-2.24850212658035));
#4229=CARTESIAN_POINT('Ctrl Pts',(18.9403808821526,-45.4094489146347,-2.24982720828383));
#4230=CARTESIAN_POINT('Ctrl Pts',(18.9335402930706,-45.4081334301734,-2.25295036904543));
#4231=CARTESIAN_POINT('Ctrl Pts',(18.9267361216311,-45.4067092269099,-2.25592187358363));
#4232=CARTESIAN_POINT('Ctrl Pts',(18.919980869073,-45.4051857902904,-2.25874456724948));
#4233=CARTESIAN_POINT('Ctrl Pts',(18.9164979549471,-45.4044003275891,-2.26019990878666));
#4234=CARTESIAN_POINT('Ctrl Pts',(18.9133662240863,-45.4036676302014,-2.2614777053349));
#4235=CARTESIAN_POINT('Ctrl Pts',(18.9100657264646,-45.4028709291528,-2.26279585730047));
#4236=CARTESIAN_POINT('Ctrl Pts',(18.908352626479,-45.402457407099,-2.26348003477071));
#4237=CARTESIAN_POINT('Ctrl Pts',(18.9065938749453,-45.4020260756094,-2.26417455035125));
#4238=CARTESIAN_POINT('Ctrl Pts',(18.9047155105794,-45.4015567031749,-2.26490618841246));
#4239=CARTESIAN_POINT('Ctrl Pts',(18.9031937725225,-45.4011764458034,-2.26549891765171));
#4240=CARTESIAN_POINT('Ctrl Pts',(18.901592767696,-45.4007709222593,-2.26611618194192));
#4241=CARTESIAN_POINT('Ctrl Pts',(18.8998729343624,-45.4003278468303,-2.26677060880248));
#4242=CARTESIAN_POINT('',(18.688654621475,-45.2109506804125,-1.32333454805209));
#4243=CARTESIAN_POINT('',(18.8905539268375,-44.7484447038531,-1.50776822046538));
#4244=CARTESIAN_POINT('',(18.6221620191364,-45.6205950568764,-1.77871850220987));
#4245=CARTESIAN_POINT('Ctrl Pts',(18.6221620189044,-45.6205950572814,-1.77871850140526));
#4246=CARTESIAN_POINT('Ctrl Pts',(18.6581806165478,-45.633462179895,-1.77145672208729));
#4247=CARTESIAN_POINT('Ctrl Pts',(18.6945296453429,-45.6411632239077,-1.75873958924297));
#4248=CARTESIAN_POINT('Ctrl Pts',(18.7659446834003,-45.6457061633278,-1.72295727333315));
#4249=CARTESIAN_POINT('Ctrl Pts',(18.8000184558857,-45.6419289228715,-1.69982222343669));
#4250=CARTESIAN_POINT('Ctrl Pts',(18.8596085346286,-45.6226944096372,-1.64648369257765));
#4251=CARTESIAN_POINT('Ctrl Pts',(18.8843459826501,-45.6074811389323,-1.61696981583715));
#4252=CARTESIAN_POINT('Ctrl Pts',(18.9243319236507,-45.5642815965227,-1.55028617227719));
#4253=CARTESIAN_POINT('Ctrl Pts',(18.9334400302693,-45.5387736862257,-1.51911880037033));
#4254=CARTESIAN_POINT('Ctrl Pts',(18.9407266713295,-45.4973521054937,-1.47275350501765));
#4255=CARTESIAN_POINT('Ctrl Pts',(18.9410687526231,-45.4684948170116,-1.44313131313073));
#4256=CARTESIAN_POINT('Ctrl Pts',(18.9201436069681,-45.4035479484512,-1.38874059277084));
#4257=CARTESIAN_POINT('Ctrl Pts',(18.9036875951198,-45.3736809974723,-1.367595125502));
#4258=CARTESIAN_POINT('Ctrl Pts',(18.8591032411742,-45.3175272792895,-1.33556085947497));
#4259=CARTESIAN_POINT('Ctrl Pts',(18.8317143369514,-45.2917456840402,-1.32476877134019));
#4260=CARTESIAN_POINT('Ctrl Pts',(18.7832988662914,-45.2570891704194,-1.31682541411965));
#4261=CARTESIAN_POINT('Ctrl Pts',(18.7651342495118,-45.2459423680159,-1.31573764809258));
#4262=CARTESIAN_POINT('Ctrl Pts',(18.7275364667659,-45.2263255413164,-1.31700978595565));
#4263=CARTESIAN_POINT('Ctrl Pts',(18.7080536577264,-45.2178461743263,-1.31938825619245));
#4264=CARTESIAN_POINT('Ctrl Pts',(18.6886546214932,-45.2109506803708,-1.32333454806873));
#4265=CARTESIAN_POINT('',(18.814383572052,-45.3725581690366,-2.29264601746227));
#4266=CARTESIAN_POINT('',(18.8143835735432,-45.3725581696516,-2.29264601707409));
#4267=CARTESIAN_POINT('Origin',(18.8502672096237,-45.0583616020844,-1.90494085304907));
#4268=CARTESIAN_POINT('Ctrl Pts',(3.62216201968442,-19.8058202438613,-1.94799199564959));
#4269=CARTESIAN_POINT('Ctrl Pts',(3.34425572651223,-20.2137053466864,-1.54490813204841));
#4270=CARTESIAN_POINT('Ctrl Pts',(3.25594179788809,-20.5121292468035,-0.988830267143717));
#4271=CARTESIAN_POINT('Ctrl Pts',(3.16762786926396,-20.8105531469205,-0.432752402239027));
#4272=CARTESIAN_POINT('Ctrl Pts',(3.3076189187292,-20.9771651064803,0.166181422977342));
#4273=CARTESIAN_POINT('Ctrl Pts',(3.44760996819445,-21.1437770660401,0.765115248193711));
#4274=CARTESIAN_POINT('Ctrl Pts',(3.80940000840298,-21.1823333185883,1.28827884419634));
#4275=CARTESIAN_POINT('Ctrl Pts',(4.17119004861151,-21.2208895711365,1.81144244019896));
#4276=CARTESIAN_POINT('Ctrl Pts',(4.70434308191443,-21.1605093534924,2.15521684061908));
#4277=CARTESIAN_POINT('Ctrl Pts',(5.23749611521735,-21.1001291358485,2.49899124103919));
#4278=CARTESIAN_POINT('Ctrl Pts',(5.8576356015542,-20.9895272661294,2.59528770975726));
#4279=CARTESIAN_POINT('Ctrl Pts',(6.47777508789106,-20.8789253964104,2.69158417847533));
#4280=CARTESIAN_POINT('Ctrl Pts',(7.08329575335921,-20.7767637068552,2.52133001886304));
#4281=CARTESIAN_POINT('Ctrl Pts',(7.68881641882736,-20.6746020173,2.35107585925076));
#4282=CARTESIAN_POINT('Ctrl Pts',(8.18100842628526,-20.6378706589539,1.94799199564959));
#4283=CARTESIAN_POINT('Ctrl Pts',(8.67320043374317,-20.6011393006078,1.54490813204841));
#4284=CARTESIAN_POINT('Ctrl Pts',(8.97580007665302,-20.6738691449698,0.988830267143717));
#4285=CARTESIAN_POINT('Ctrl Pts',(9.27839971956287,-20.7465989893318,0.432752402239027));
#4286=CARTESIAN_POINT('Ctrl Pts',(9.35269438438334,-20.9511407742511,-0.166181422977342));
#4287=CARTESIAN_POINT('Ctrl Pts',(9.4269890492038,-21.1556825591703,-0.765115248193711));
#4288=CARTESIAN_POINT('Ctrl Pts',(9.27948472328098,-21.4882800511012,-1.28827884419634));
#4289=CARTESIAN_POINT('Ctrl Pts',(9.13198039735816,-21.8208775430321,-1.81144244019896));
#4290=CARTESIAN_POINT('Ctrl Pts',(8.81311307834095,-22.2524115051551,-2.15521684061908));
#4291=CARTESIAN_POINT('Ctrl Pts',(8.49424575932375,-22.6839454672782,-2.49899124103919));
#4292=CARTESIAN_POINT('Ctrl Pts',(8.0883919872726,-23.1657010814762,-2.59528770975726));
#4293=CARTESIAN_POINT('Ctrl Pts',(7.68253821522146,-23.6474566956743,-2.69158417847533));
#4294=CARTESIAN_POINT('Ctrl Pts',(7.29130326403902,-24.1207721297085,-2.52133001886305));
#4295=CARTESIAN_POINT('Ctrl Pts',(6.90006831285659,-24.5940875637428,-2.35107585925076));
#4296=CARTESIAN_POINT('Ctrl Pts',(6.62216201968439,-25.0019726665679,-1.94799199564959));
#4297=CARTESIAN_POINT('Ctrl Pts',(6.34425572651219,-25.4098577693931,-1.54490813204841));
#4298=CARTESIAN_POINT('Ctrl Pts',(6.25594179788806,-25.7082816695101,-0.988830267143717));
#4299=CARTESIAN_POINT('Ctrl Pts',(6.16762786926392,-26.0067055696272,-0.432752402239027));
#4300=CARTESIAN_POINT('Ctrl Pts',(6.30761891872917,-26.1733175291869,0.166181422977342));
#4301=CARTESIAN_POINT('Ctrl Pts',(6.44760996819441,-26.3399294887468,0.765115248193711));
#4302=CARTESIAN_POINT('Ctrl Pts',(6.80940000840295,-26.3784857412949,1.28827884419634));
#4303=CARTESIAN_POINT('Ctrl Pts',(7.17119004861148,-26.4170419938431,1.81144244019896));
#4304=CARTESIAN_POINT('Ctrl Pts',(7.7043430819144,-26.3566617761991,2.15521684061908));
#4305=CARTESIAN_POINT('Ctrl Pts',(8.23749611521731,-26.2962815585551,2.49899124103919));
#4306=CARTESIAN_POINT('Ctrl Pts',(8.85763560155417,-26.1856796888361,2.59528770975726));
#4307=CARTESIAN_POINT('Ctrl Pts',(9.47777508789103,-26.0750778191171,2.69158417847533));
#4308=CARTESIAN_POINT('Ctrl Pts',(10.0832957533592,-25.9729161295619,2.52133001886304));
#4309=CARTESIAN_POINT('Ctrl Pts',(10.6888164188273,-25.8707544400067,2.35107585925076));
#4310=CARTESIAN_POINT('Ctrl Pts',(11.1810084262852,-25.8340230816606,1.94799199564959));
#4311=CARTESIAN_POINT('Ctrl Pts',(11.6732004337431,-25.7972917233145,1.54490813204841));
#4312=CARTESIAN_POINT('Ctrl Pts',(11.975800076653,-25.8700215676765,0.988830267143717));
#4313=CARTESIAN_POINT('Ctrl Pts',(12.2783997195628,-25.9427514120385,0.432752402239027));
#4314=CARTESIAN_POINT('Ctrl Pts',(12.3526943843833,-26.1472931969577,-0.166181422977342));
#4315=CARTESIAN_POINT('Ctrl Pts',(12.4269890492038,-26.351834981877,-0.765115248193711));
#4316=CARTESIAN_POINT('Ctrl Pts',(12.279484723281,-26.6844324738078,-1.28827884419634));
#4317=CARTESIAN_POINT('Ctrl Pts',(12.1319803973581,-27.0170299657387,-1.81144244019896));
#4318=CARTESIAN_POINT('Ctrl Pts',(11.8131130783409,-27.4485639278618,-2.15521684061908));
#4319=CARTESIAN_POINT('Ctrl Pts',(11.4942457593237,-27.8800978899848,-2.49899124103919));
#4320=CARTESIAN_POINT('Ctrl Pts',(11.0883919872726,-28.3618535041829,-2.59528770975726));
#4321=CARTESIAN_POINT('Ctrl Pts',(10.6825382152214,-28.8436091183809,-2.69158417847533));
#4322=CARTESIAN_POINT('Ctrl Pts',(10.291303264039,-29.3169245524152,-2.52133001886305));
#4323=CARTESIAN_POINT('Ctrl Pts',(9.90006831285655,-29.7902399864494,-2.35107585925076));
#4324=CARTESIAN_POINT('Ctrl Pts',(9.62216201968436,-30.1981250892746,-1.94799199564959));
#4325=CARTESIAN_POINT('Ctrl Pts',(9.34425572651217,-30.6060101920997,-1.54490813204841));
#4326=CARTESIAN_POINT('Ctrl Pts',(9.25594179788803,-30.9044340922168,-0.988830267143717));
#4327=CARTESIAN_POINT('Ctrl Pts',(9.16762786926389,-31.2028579923338,-0.432752402239027));
#4328=CARTESIAN_POINT('Ctrl Pts',(9.30761891872914,-31.3694699518936,0.166181422977342));
#4329=CARTESIAN_POINT('Ctrl Pts',(9.44760996819438,-31.5360819114534,0.765115248193711));
#4330=CARTESIAN_POINT('Ctrl Pts',(9.80940000840292,-31.5746381640016,1.28827884419634));
#4331=CARTESIAN_POINT('Ctrl Pts',(10.1711900486115,-31.6131944165497,1.81144244019896));
#4332=CARTESIAN_POINT('Ctrl Pts',(10.7043430819144,-31.5528141989058,2.15521684061908));
#4333=CARTESIAN_POINT('Ctrl Pts',(11.2374961152173,-31.4924339812617,2.49899124103919));
#4334=CARTESIAN_POINT('Ctrl Pts',(11.8576356015541,-31.3818321115427,2.59528770975726));
#4335=CARTESIAN_POINT('Ctrl Pts',(12.477775087891,-31.2712302418237,2.69158417847533));
#4336=CARTESIAN_POINT('Ctrl Pts',(13.0832957533591,-31.1690685522685,2.52133001886304));
#4337=CARTESIAN_POINT('Ctrl Pts',(13.6888164188273,-31.0669068627133,2.35107585925076));
#4338=CARTESIAN_POINT('Ctrl Pts',(14.1810084262852,-31.0301755043672,1.94799199564959));
#4339=CARTESIAN_POINT('Ctrl Pts',(14.6732004337431,-30.9934441460211,1.54490813204841));
#4340=CARTESIAN_POINT('Ctrl Pts',(14.975800076653,-31.0661739903831,0.988830267143717));
#4341=CARTESIAN_POINT('Ctrl Pts',(15.2783997195628,-31.1389038347451,0.432752402239027));
#4342=CARTESIAN_POINT('Ctrl Pts',(15.3526943843833,-31.3434456196644,-0.166181422977342));
#4343=CARTESIAN_POINT('Ctrl Pts',(15.4269890492037,-31.5479874045836,-0.765115248193711));
#4344=CARTESIAN_POINT('Ctrl Pts',(15.2794847232809,-31.8805848965145,-1.28827884419634));
#4345=CARTESIAN_POINT('Ctrl Pts',(15.1319803973581,-32.2131823884454,-1.81144244019896));
#4346=CARTESIAN_POINT('Ctrl Pts',(14.8131130783409,-32.6447163505684,-2.15521684061908));
#4347=CARTESIAN_POINT('Ctrl Pts',(14.4942457593237,-33.0762503126915,-2.49899124103919));
#4348=CARTESIAN_POINT('Ctrl Pts',(14.0883919872725,-33.5580059268895,-2.59528770975726));
#4349=CARTESIAN_POINT('Ctrl Pts',(13.6825382152214,-34.0397615410876,-2.69158417847533));
#4350=CARTESIAN_POINT('Ctrl Pts',(13.291303264039,-34.5130769751218,-2.52133001886305));
#4351=CARTESIAN_POINT('Ctrl Pts',(12.9000683128565,-34.9863924091561,-2.35107585925076));
#4352=CARTESIAN_POINT('Ctrl Pts',(12.6221620196843,-35.3942775119812,-1.94799199564959));
#4353=CARTESIAN_POINT('Ctrl Pts',(12.3442557265121,-35.8021626148064,-1.54490813204841));
#4354=CARTESIAN_POINT('Ctrl Pts',(12.255941797888,-36.1005865149234,-0.988830267143717));
#4355=CARTESIAN_POINT('Ctrl Pts',(12.1676278692639,-36.3990104150405,-0.432752402239027));
#4356=CARTESIAN_POINT('Ctrl Pts',(12.3076189187291,-36.5656223746002,0.166181422977342));
#4357=CARTESIAN_POINT('Ctrl Pts',(12.4476099681944,-36.73223433416,0.765115248193711));
#4358=CARTESIAN_POINT('Ctrl Pts',(12.8094000084029,-36.7707905867082,1.28827884419634));
#4359=CARTESIAN_POINT('Ctrl Pts',(13.1711900486114,-36.8093468392564,1.81144244019896));
#4360=CARTESIAN_POINT('Ctrl Pts',(13.7043430819143,-36.7489666216124,2.15521684061908));
#4361=CARTESIAN_POINT('Ctrl Pts',(14.2374961152173,-36.6885864039684,2.49899124103919));
#4362=CARTESIAN_POINT('Ctrl Pts',(14.8576356015541,-36.5779845342494,2.59528770975726));
#4363=CARTESIAN_POINT('Ctrl Pts',(15.477775087891,-36.4673826645304,2.69158417847533));
#4364=CARTESIAN_POINT('Ctrl Pts',(16.0832957533591,-36.3652209749752,2.52133001886304));
#4365=CARTESIAN_POINT('Ctrl Pts',(16.6888164188273,-36.26305928542,2.35107585925076));
#4366=CARTESIAN_POINT('Ctrl Pts',(17.1810084262852,-36.2263279270739,1.94799199564959));
#4367=CARTESIAN_POINT('Ctrl Pts',(17.6732004337431,-36.1895965687278,1.54490813204841));
#4368=CARTESIAN_POINT('Ctrl Pts',(17.9758000766529,-36.2623264130898,0.988830267143717));
#4369=CARTESIAN_POINT('Ctrl Pts',(18.2783997195628,-36.3350562574518,0.432752402239027));
#4370=CARTESIAN_POINT('Ctrl Pts',(18.3526943843832,-36.539598042371,-0.166181422977342));
#4371=CARTESIAN_POINT('Ctrl Pts',(18.4269890492037,-36.7441398272903,-0.765115248193711));
#4372=CARTESIAN_POINT('Ctrl Pts',(18.2794847232809,-37.0767373192211,-1.28827884419634));
#4373=CARTESIAN_POINT('Ctrl Pts',(18.1319803973581,-37.409334811152,-1.81144244019896));
#4374=CARTESIAN_POINT('Ctrl Pts',(17.8131130783409,-37.8408687732751,-2.15521684061908));
#4375=CARTESIAN_POINT('Ctrl Pts',(17.4942457593237,-38.2724027353981,-2.49899124103919));
#4376=CARTESIAN_POINT('Ctrl Pts',(17.0883919872725,-38.7541583495962,-2.59528770975726));
#4377=CARTESIAN_POINT('Ctrl Pts',(16.6825382152214,-39.2359139637942,-2.69158417847533));
#4378=CARTESIAN_POINT('Ctrl Pts',(16.2913032640389,-39.7092293978285,-2.52133001886305));
#4379=CARTESIAN_POINT('Ctrl Pts',(15.9000683128565,-40.1825448318627,-2.35107585925076));
#4380=CARTESIAN_POINT('Ctrl Pts',(15.6221620196843,-40.5904299346879,-1.94799199564959));
#4381=CARTESIAN_POINT('Ctrl Pts',(15.3442557265121,-40.998315037513,-1.54490813204841));
#4382=CARTESIAN_POINT('Ctrl Pts',(15.255941797888,-41.2967389376301,-0.988830267143717));
#4383=CARTESIAN_POINT('Ctrl Pts',(15.1676278692638,-41.5951628377471,-0.432752402239027));
#4384=CARTESIAN_POINT('Ctrl Pts',(15.3076189187291,-41.7617747973069,0.166181422977342));
#4385=CARTESIAN_POINT('Ctrl Pts',(15.4476099681943,-41.9283867568667,0.765115248193711));
#4386=CARTESIAN_POINT('Ctrl Pts',(15.8094000084029,-41.9669430094149,1.28827884419634));
#4387=CARTESIAN_POINT('Ctrl Pts',(16.1711900486114,-42.0054992619631,1.81144244019896));
#4388=CARTESIAN_POINT('Ctrl Pts',(16.7043430819143,-41.945119044319,2.15521684061908));
#4389=CARTESIAN_POINT('Ctrl Pts',(17.2374961152172,-41.884738826675,2.49899124103919));
#4390=CARTESIAN_POINT('Ctrl Pts',(17.8576356015541,-41.774136956956,2.59528770975726));
#4391=CARTESIAN_POINT('Ctrl Pts',(18.4777750878909,-41.6635350872371,2.69158417847533));
#4392=CARTESIAN_POINT('Ctrl Pts',(19.0832957533591,-41.5613733976818,2.52133001886304));
#4393=CARTESIAN_POINT('Ctrl Pts',(19.6888164188272,-41.4592117081266,2.35107585925076));
#4394=CARTESIAN_POINT('Ctrl Pts',(20.1810084262851,-41.4224803497805,1.94799199564959));
#4395=CARTESIAN_POINT('Ctrl Pts',(20.673200433743,-41.3857489914344,1.54490813204841));
#4396=CARTESIAN_POINT('Ctrl Pts',(20.9758000766529,-41.4584788357964,0.988830267143717));
#4397=CARTESIAN_POINT('Ctrl Pts',(21.2783997195627,-41.5312086801584,0.432752402239027));
#4398=CARTESIAN_POINT('Ctrl Pts',(21.3526943843832,-41.7357504650777,-0.166181422977342));
#4399=CARTESIAN_POINT('Ctrl Pts',(21.4269890492037,-41.940292249997,-0.765115248193711));
#4400=CARTESIAN_POINT('Ctrl Pts',(21.2794847232809,-42.2728897419278,-1.28827884419634));
#4401=CARTESIAN_POINT('Ctrl Pts',(21.131980397358,-42.6054872338587,-1.81144244019896));
#4402=CARTESIAN_POINT('Ctrl Pts',(20.8131130783408,-43.0370211959817,-2.15521684061908));
#4403=CARTESIAN_POINT('Ctrl Pts',(20.4942457593236,-43.4685551581048,-2.49899124103919));
#4404=CARTESIAN_POINT('Ctrl Pts',(20.0883919872725,-43.9503107723028,-2.59528770975726));
#4405=CARTESIAN_POINT('Ctrl Pts',(19.6825382152213,-44.4320663865008,-2.69158417847533));
#4406=CARTESIAN_POINT('Ctrl Pts',(19.2913032640389,-44.9053818205351,-2.52133001886305));
#4407=CARTESIAN_POINT('Ctrl Pts',(18.9000683128565,-45.3786972545694,-2.35107585925076));
#4408=CARTESIAN_POINT('Ctrl Pts',(18.6221620196843,-45.7865823573945,-1.94799199564959));
#4409=CARTESIAN_POINT('Ctrl Pts',(4.55184415422078,-20.0688325405066,-1.69008569379309));
#4410=CARTESIAN_POINT('Ctrl Pts',(4.32491681918215,-20.4472849281303,-1.4407517010054));
#4411=CARTESIAN_POINT('Ctrl Pts',(4.22476116346577,-20.7525456525717,-1.04873843619563));
#4412=CARTESIAN_POINT('Ctrl Pts',(4.12460550774938,-21.0578063770131,-0.656725171385866));
#4413=CARTESIAN_POINT('Ctrl Pts',(4.19227954417643,-21.2661705835175,-0.199675669376779));
#4414=CARTESIAN_POINT('Ctrl Pts',(4.25995358060348,-21.4745347900219,0.257373832632308));
#4415=CARTESIAN_POINT('Ctrl Pts',(4.50327459317005,-21.5814891675698,0.688935312623524));
#4416=CARTESIAN_POINT('Ctrl Pts',(4.74659560573663,-21.6884435451177,1.12049679261474));
#4417=CARTESIAN_POINT('Ctrl Pts',(5.13859184064558,-21.7095602430244,1.44109420672161));
#4418=CARTESIAN_POINT('Ctrl Pts',(5.53058807555453,-21.7306769409311,1.76169162082848));
#4419=CARTESIAN_POINT('Ctrl Pts',(6.01484082784187,-21.6985293136949,1.90782671931788));
#4420=CARTESIAN_POINT('Ctrl Pts',(6.49909358012921,-21.6663816864587,2.05396181780729));
#4421=CARTESIAN_POINT('Ctrl Pts',(7.00091161011221,-21.6240927414165,1.99669075219403));
#4422=CARTESIAN_POINT('Ctrl Pts',(7.50272964009522,-21.5818037963743,1.93941968658077));
#4423=CARTESIAN_POINT('Ctrl Pts',(7.94394268941957,-21.5745051532296,1.69008569379309));
#4424=CARTESIAN_POINT('Ctrl Pts',(8.38515573874391,-21.5672065100849,1.4407517010054));
#4425=CARTESIAN_POINT('Ctrl Pts',(8.699597108746,-21.6330995301225,1.04873843619563));
#4426=CARTESIAN_POINT('Ctrl Pts',(9.0140384787481,-21.6989925501602,0.656725171385866));
#4427=CARTESIAN_POINT('Ctrl Pts',(9.16065015660677,-21.8617820881348,0.199675669376779));
#4428=CARTESIAN_POINT('Ctrl Pts',(9.30726183446543,-22.0245716261095,-0.257373832632308));
#4429=CARTESIAN_POINT('Ctrl Pts',(9.27822653618457,-22.2887709930406,-0.688935312623524));
#4430=CARTESIAN_POINT('Ctrl Pts',(9.24919123790371,-22.5529703599718,-1.12049679261474));
#4431=CARTESIAN_POINT('Ctrl Pts',(9.07148071728047,-22.9030074065441,-1.44109420672161));
#4432=CARTESIAN_POINT('Ctrl Pts',(8.89377019665723,-23.2530444531165,-1.76169162082848));
#4433=CARTESIAN_POINT('Ctrl Pts',(8.6238031586556,-23.6563458248317,-1.90782671931788));
#4434=CARTESIAN_POINT('Ctrl Pts',(8.35383612065398,-24.059647196547,-2.05396181780729));
#4435=CARTESIAN_POINT('Ctrl Pts',(8.06630380495668,-24.4730898860682,-1.99669075219403));
#4436=CARTESIAN_POINT('Ctrl Pts',(7.77877148925938,-24.8865325755895,-1.93941968658077));
#4437=CARTESIAN_POINT('Ctrl Pts',(7.55184415422075,-25.2649849632132,-1.69008569379309));
#4438=CARTESIAN_POINT('Ctrl Pts',(7.32491681918212,-25.6434373508369,-1.4407517010054));
#4439=CARTESIAN_POINT('Ctrl Pts',(7.22476116346574,-25.9486980752784,-1.04873843619563));
#4440=CARTESIAN_POINT('Ctrl Pts',(7.12460550774935,-26.2539587997198,-0.656725171385866));
#4441=CARTESIAN_POINT('Ctrl Pts',(7.1922795441764,-26.4623230062242,-0.199675669376779));
#4442=CARTESIAN_POINT('Ctrl Pts',(7.25995358060345,-26.6706872127285,0.257373832632308));
#4443=CARTESIAN_POINT('Ctrl Pts',(7.50327459317002,-26.7776415902764,0.688935312623524));
#4444=CARTESIAN_POINT('Ctrl Pts',(7.7465956057366,-26.8845959678243,1.12049679261474));
#4445=CARTESIAN_POINT('Ctrl Pts',(8.13859184064555,-26.905712665731,1.44109420672161));
#4446=CARTESIAN_POINT('Ctrl Pts',(8.5305880755545,-26.9268293636377,1.76169162082848));
#4447=CARTESIAN_POINT('Ctrl Pts',(9.01484082784184,-26.8946817364015,1.90782671931788));
#4448=CARTESIAN_POINT('Ctrl Pts',(9.49909358012917,-26.8625341091653,2.05396181780729));
#4449=CARTESIAN_POINT('Ctrl Pts',(10.0009116101122,-26.8202451641231,1.99669075219403));
#4450=CARTESIAN_POINT('Ctrl Pts',(10.5027296400952,-26.7779562190809,1.93941968658077));
#4451=CARTESIAN_POINT('Ctrl Pts',(10.9439426894195,-26.7706575759362,1.69008569379309));
#4452=CARTESIAN_POINT('Ctrl Pts',(11.3851557387439,-26.7633589327915,1.4407517010054));
#4453=CARTESIAN_POINT('Ctrl Pts',(11.699597108746,-26.8292519528292,1.04873843619563));
#4454=CARTESIAN_POINT('Ctrl Pts',(12.0140384787481,-26.8951449728668,0.656725171385866));
#4455=CARTESIAN_POINT('Ctrl Pts',(12.1606501566067,-27.0579345108415,0.199675669376779));
#4456=CARTESIAN_POINT('Ctrl Pts',(12.3072618344654,-27.2207240488161,-0.257373832632308));
#4457=CARTESIAN_POINT('Ctrl Pts',(12.2782265361845,-27.4849234157473,-0.688935312623524));
#4458=CARTESIAN_POINT('Ctrl Pts',(12.2491912379037,-27.7491227826784,-1.12049679261474));
#4459=CARTESIAN_POINT('Ctrl Pts',(12.0714807172804,-28.0991598292508,-1.44109420672161));
#4460=CARTESIAN_POINT('Ctrl Pts',(11.8937701966572,-28.4491968758231,-1.76169162082848));
#4461=CARTESIAN_POINT('Ctrl Pts',(11.6238031586556,-28.8524982475384,-1.90782671931788));
#4462=CARTESIAN_POINT('Ctrl Pts',(11.3538361206539,-29.2557996192536,-2.05396181780729));
#4463=CARTESIAN_POINT('Ctrl Pts',(11.0663038049567,-29.6692423087749,-1.99669075219403));
#4464=CARTESIAN_POINT('Ctrl Pts',(10.7787714892594,-30.0826849982961,-1.93941968658077));
#4465=CARTESIAN_POINT('Ctrl Pts',(10.5518441542207,-30.4611373859199,-1.69008569379309));
#4466=CARTESIAN_POINT('Ctrl Pts',(10.3249168191821,-30.8395897735436,-1.4407517010054));
#4467=CARTESIAN_POINT('Ctrl Pts',(10.2247611634657,-31.144850497985,-1.04873843619563));
#4468=CARTESIAN_POINT('Ctrl Pts',(10.1246055077493,-31.4501112224264,-0.656725171385866));
#4469=CARTESIAN_POINT('Ctrl Pts',(10.1922795441764,-31.6584754289308,-0.199675669376779));
#4470=CARTESIAN_POINT('Ctrl Pts',(10.2599535806034,-31.8668396354352,0.257373832632308));
#4471=CARTESIAN_POINT('Ctrl Pts',(10.50327459317,-31.9737940129831,0.688935312623524));
#4472=CARTESIAN_POINT('Ctrl Pts',(10.7465956057366,-32.080748390531,1.12049679261474));
#4473=CARTESIAN_POINT('Ctrl Pts',(11.1385918406455,-32.1018650884377,1.44109420672161));
#4474=CARTESIAN_POINT('Ctrl Pts',(11.5305880755545,-32.1229817863444,1.76169162082848));
#4475=CARTESIAN_POINT('Ctrl Pts',(12.0148408278418,-32.0908341591082,1.90782671931788));
#4476=CARTESIAN_POINT('Ctrl Pts',(12.4990935801291,-32.0586865318719,2.05396181780729));
#4477=CARTESIAN_POINT('Ctrl Pts',(13.0009116101121,-32.0163975868298,1.99669075219403));
#4478=CARTESIAN_POINT('Ctrl Pts',(13.5027296400952,-31.9741086417876,1.93941968658077));
#4479=CARTESIAN_POINT('Ctrl Pts',(13.9439426894195,-31.9668099986429,1.69008569379309));
#4480=CARTESIAN_POINT('Ctrl Pts',(14.3851557387438,-31.9595113554982,1.4407517010054));
#4481=CARTESIAN_POINT('Ctrl Pts',(14.6995971087459,-32.0254043755358,1.04873843619563));
#4482=CARTESIAN_POINT('Ctrl Pts',(15.014038478748,-32.0912973955735,0.656725171385866));
#4483=CARTESIAN_POINT('Ctrl Pts',(15.1606501566067,-32.2540869335481,0.199675669376779));
#4484=CARTESIAN_POINT('Ctrl Pts',(15.3072618344654,-32.4168764715228,-0.257373832632308));
#4485=CARTESIAN_POINT('Ctrl Pts',(15.2782265361845,-32.6810758384539,-0.688935312623524));
#4486=CARTESIAN_POINT('Ctrl Pts',(15.2491912379036,-32.9452752053851,-1.12049679261474));
#4487=CARTESIAN_POINT('Ctrl Pts',(15.0714807172804,-33.2953122519574,-1.44109420672161));
#4488=CARTESIAN_POINT('Ctrl Pts',(14.8937701966572,-33.6453492985298,-1.76169162082848));
#4489=CARTESIAN_POINT('Ctrl Pts',(14.6238031586555,-34.048650670245,-1.90782671931788));
#4490=CARTESIAN_POINT('Ctrl Pts',(14.3538361206539,-34.4519520419603,-2.05396181780729));
#4491=CARTESIAN_POINT('Ctrl Pts',(14.0663038049566,-34.8653947314815,-1.99669075219403));
#4492=CARTESIAN_POINT('Ctrl Pts',(13.7787714892593,-35.2788374210028,-1.93941968658077));
#4493=CARTESIAN_POINT('Ctrl Pts',(13.5518441542207,-35.6572898086265,-1.69008569379309));
#4494=CARTESIAN_POINT('Ctrl Pts',(13.3249168191821,-36.0357421962502,-1.4407517010054));
#4495=CARTESIAN_POINT('Ctrl Pts',(13.2247611634657,-36.3410029206916,-1.04873843619563));
#4496=CARTESIAN_POINT('Ctrl Pts',(13.1246055077493,-36.6462636451331,-0.656725171385866));
#4497=CARTESIAN_POINT('Ctrl Pts',(13.1922795441763,-36.8546278516375,-0.199675669376779));
#4498=CARTESIAN_POINT('Ctrl Pts',(13.2599535806034,-37.0629920581418,0.257373832632308));
#4499=CARTESIAN_POINT('Ctrl Pts',(13.50327459317,-37.1699464356897,0.688935312623524));
#4500=CARTESIAN_POINT('Ctrl Pts',(13.7465956057365,-37.2769008132376,1.12049679261474));
#4501=CARTESIAN_POINT('Ctrl Pts',(14.1385918406455,-37.2980175111443,1.44109420672161));
#4502=CARTESIAN_POINT('Ctrl Pts',(14.5305880755544,-37.319134209051,1.76169162082848));
#4503=CARTESIAN_POINT('Ctrl Pts',(15.0148408278418,-37.2869865818148,1.90782671931788));
#4504=CARTESIAN_POINT('Ctrl Pts',(15.4990935801291,-37.2548389545786,2.05396181780729));
#4505=CARTESIAN_POINT('Ctrl Pts',(16.0009116101121,-37.2125500095364,1.99669075219403));
#4506=CARTESIAN_POINT('Ctrl Pts',(16.5027296400951,-37.1702610644942,1.93941968658077));
#4507=CARTESIAN_POINT('Ctrl Pts',(16.9439426894195,-37.1629624213495,1.69008569379309));
#4508=CARTESIAN_POINT('Ctrl Pts',(17.3851557387438,-37.1556637782049,1.4407517010054));
#4509=CARTESIAN_POINT('Ctrl Pts',(17.6995971087459,-37.2215567982425,1.04873843619563));
#4510=CARTESIAN_POINT('Ctrl Pts',(18.014038478748,-37.2874498182801,0.656725171385866));
#4511=CARTESIAN_POINT('Ctrl Pts',(18.1606501566067,-37.4502393562548,0.199675669376779));
#4512=CARTESIAN_POINT('Ctrl Pts',(18.3072618344653,-37.6130288942294,-0.257373832632308));
#4513=CARTESIAN_POINT('Ctrl Pts',(18.2782265361845,-37.8772282611606,-0.688935312623524));
#4514=CARTESIAN_POINT('Ctrl Pts',(18.2491912379036,-38.1414276280917,-1.12049679261474));
#4515=CARTESIAN_POINT('Ctrl Pts',(18.0714807172804,-38.4914646746641,-1.44109420672161));
#4516=CARTESIAN_POINT('Ctrl Pts',(17.8937701966571,-38.8415017212364,-1.76169162082848));
#4517=CARTESIAN_POINT('Ctrl Pts',(17.6238031586555,-39.2448030929517,-1.90782671931788));
#4518=CARTESIAN_POINT('Ctrl Pts',(17.3538361206539,-39.6481044646669,-2.05396181780729));
#4519=CARTESIAN_POINT('Ctrl Pts',(17.0663038049566,-40.0615471541882,-1.99669075219403));
#4520=CARTESIAN_POINT('Ctrl Pts',(16.7787714892593,-40.4749898437094,-1.93941968658077));
#4521=CARTESIAN_POINT('Ctrl Pts',(16.5518441542207,-40.8534422313332,-1.69008569379309));
#4522=CARTESIAN_POINT('Ctrl Pts',(16.324916819182,-41.2318946189569,-1.4407517010054));
#4523=CARTESIAN_POINT('Ctrl Pts',(16.2247611634656,-41.5371553433983,-1.04873843619563));
#4524=CARTESIAN_POINT('Ctrl Pts',(16.1246055077493,-41.8424160678397,-0.656725171385866));
#4525=CARTESIAN_POINT('Ctrl Pts',(16.1922795441763,-42.0507802743441,-0.199675669376779));
#4526=CARTESIAN_POINT('Ctrl Pts',(16.2599535806034,-42.2591444808485,0.257373832632308));
#4527=CARTESIAN_POINT('Ctrl Pts',(16.5032745931699,-42.3660988583964,0.688935312623524));
#4528=CARTESIAN_POINT('Ctrl Pts',(16.7465956057365,-42.4730532359443,1.12049679261474));
#4529=CARTESIAN_POINT('Ctrl Pts',(17.1385918406455,-42.494169933851,1.44109420672161));
#4530=CARTESIAN_POINT('Ctrl Pts',(17.5305880755544,-42.5152866317577,1.76169162082848));
#4531=CARTESIAN_POINT('Ctrl Pts',(18.0148408278417,-42.4831390045215,1.90782671931788));
#4532=CARTESIAN_POINT('Ctrl Pts',(18.4990935801291,-42.4509913772853,2.05396181780729));
#4533=CARTESIAN_POINT('Ctrl Pts',(19.0009116101121,-42.4087024322431,1.99669075219403));
#4534=CARTESIAN_POINT('Ctrl Pts',(19.5027296400951,-42.3664134872009,1.93941968658077));
#4535=CARTESIAN_POINT('Ctrl Pts',(19.9439426894194,-42.3591148440562,1.69008569379309));
#4536=CARTESIAN_POINT('Ctrl Pts',(20.3851557387438,-42.3518162009115,1.4407517010054));
#4537=CARTESIAN_POINT('Ctrl Pts',(20.6995971087459,-42.4177092209491,1.04873843619563));
#4538=CARTESIAN_POINT('Ctrl Pts',(21.014038478748,-42.4836022409868,0.656725171385866));
#4539=CARTESIAN_POINT('Ctrl Pts',(21.1606501566066,-42.6463917789614,0.199675669376779));
#4540=CARTESIAN_POINT('Ctrl Pts',(21.3072618344653,-42.8091813169361,-0.257373832632308));
#4541=CARTESIAN_POINT('Ctrl Pts',(21.2782265361844,-43.0733806838672,-0.688935312623524));
#4542=CARTESIAN_POINT('Ctrl Pts',(21.2491912379036,-43.3375800507984,-1.12049679261474));
#4543=CARTESIAN_POINT('Ctrl Pts',(21.0714807172803,-43.6876170973707,-1.44109420672161));
#4544=CARTESIAN_POINT('Ctrl Pts',(20.8937701966571,-44.0376541439431,-1.76169162082848));
#4545=CARTESIAN_POINT('Ctrl Pts',(20.6238031586555,-44.4409555156583,-1.90782671931788));
#4546=CARTESIAN_POINT('Ctrl Pts',(20.3538361206538,-44.8442568873736,-2.05396181780729));
#4547=CARTESIAN_POINT('Ctrl Pts',(20.0663038049566,-45.2576995768948,-1.99669075219403));
#4548=CARTESIAN_POINT('Ctrl Pts',(19.7787714892593,-45.6711422664161,-1.93941968658077));
#4549=CARTESIAN_POINT('Ctrl Pts',(19.5518441542206,-46.0495946540398,-1.69008569379309));
#4550=CARTESIAN_POINT('Ctrl Pts',(4.55184415422078,-19.3686903861425,-0.976082217833403));
#4551=CARTESIAN_POINT('Ctrl Pts',(4.4660500642644,-19.6656594567264,-0.80664966398524));
#4552=CARTESIAN_POINT('Ctrl Pts',(4.46302775611024,-19.9148402168055,-0.557333680706485));
#4553=CARTESIAN_POINT('Ctrl Pts',(4.46000544795609,-20.1640209768846,-0.30801769742773));
#4554=CARTESIAN_POINT('Ctrl Pts',(4.56157448367832,-20.3528158964217,-0.0281983728666175));
#4555=CARTESIAN_POINT('Ctrl Pts',(4.66314351940055,-20.5416108159588,0.251620951694495));
#4556=CARTESIAN_POINT('Ctrl Pts',(4.87040786268996,-20.66938252122,0.506521968549832));
#4557=CARTESIAN_POINT('Ctrl Pts',(5.07767220597936,-20.7971542264811,0.761422985405168));
#4558=CARTESIAN_POINT('Ctrl Pts',(5.37080156859517,-20.8753517397202,0.940919422010711));
#4559=CARTESIAN_POINT('Ctrl Pts',(5.66393093121099,-20.9535492529593,1.12041585861625));
#4560=CARTESIAN_POINT('Ctrl Pts',(6.00608840476948,-21.0034403731477,1.18895624432295));
#4561=CARTESIAN_POINT('Ctrl Pts',(6.34824587832798,-21.0533314933362,1.25749663002964));
#4562=CARTESIAN_POINT('Ctrl Pts',(6.69288393578292,-21.1017904477443,1.2015057008556));
#4563=CARTESIAN_POINT('Ctrl Pts',(7.03752199323787,-21.1502494021524,1.14551477168157));
#4564=CARTESIAN_POINT('Ctrl Pts',(7.33760179747996,-21.2244340760476,0.976082217833403));
#4565=CARTESIAN_POINT('Ctrl Pts',(7.63768160172206,-21.2986187499427,0.80664966398524));
#4566=CARTESIAN_POINT('Ctrl Pts',(7.85498962416192,-21.4205917343427,0.557333680706485));
#4567=CARTESIAN_POINT('Ctrl Pts',(8.07229764660179,-21.5425647187427,0.308017697427731));
#4568=CARTESIAN_POINT('Ctrl Pts',(8.18501432516527,-21.7249235436846,0.0281983728666177));
#4569=CARTESIAN_POINT('Ctrl Pts',(8.29773100372875,-21.9072823686265,-0.251620951694495));
#4570=CARTESIAN_POINT('Ctrl Pts',(8.30475237472506,-22.1506644078444,-0.506521968549832));
#4571=CARTESIAN_POINT('Ctrl Pts',(8.31177374572137,-22.3940464470623,-0.761422985405168));
#4572=CARTESIAN_POINT('Ctrl Pts',(8.23293009739127,-22.6870026783022,-0.940919422010711));
#4573=CARTESIAN_POINT('Ctrl Pts',(8.15408644906117,-22.9799589095422,-1.12041585861625));
#4574=CARTESIAN_POINT('Ctrl Pts',(8.02621468978838,-23.3012215338328,-1.18895624432295));
#4575=CARTESIAN_POINT('Ctrl Pts',(7.8983429305156,-23.6224841581234,-1.25749663002964));
#4576=CARTESIAN_POINT('Ctrl Pts',(7.76799058734637,-23.9451789481943,-1.2015057008556));
#4577=CARTESIAN_POINT('Ctrl Pts',(7.63763824417713,-24.2678737382653,-1.14551477168157));
#4578=CARTESIAN_POINT('Ctrl Pts',(7.55184415422075,-24.5648428088492,-0.976082217833403));
#4579=CARTESIAN_POINT('Ctrl Pts',(7.46605006426437,-24.8618118794331,-0.80664966398524));
#4580=CARTESIAN_POINT('Ctrl Pts',(7.46302775611021,-25.1109926395121,-0.557333680706485));
#4581=CARTESIAN_POINT('Ctrl Pts',(7.46000544795606,-25.3601733995912,-0.30801769742773));
#4582=CARTESIAN_POINT('Ctrl Pts',(7.56157448367829,-25.5489683191283,-0.0281983728666175));
#4583=CARTESIAN_POINT('Ctrl Pts',(7.66314351940052,-25.7377632386655,0.251620951694495));
#4584=CARTESIAN_POINT('Ctrl Pts',(7.87040786268992,-25.8655349439266,0.506521968549832));
#4585=CARTESIAN_POINT('Ctrl Pts',(8.07767220597933,-25.9933066491878,0.761422985405168));
#4586=CARTESIAN_POINT('Ctrl Pts',(8.37080156859514,-26.0715041624269,0.940919422010711));
#4587=CARTESIAN_POINT('Ctrl Pts',(8.66393093121095,-26.1497016756659,1.12041585861625));
#4588=CARTESIAN_POINT('Ctrl Pts',(9.00608840476945,-26.1995927958544,1.18895624432295));
#4589=CARTESIAN_POINT('Ctrl Pts',(9.34824587832795,-26.2494839160429,1.25749663002964));
#4590=CARTESIAN_POINT('Ctrl Pts',(9.69288393578289,-26.297942870451,1.2015057008556));
#4591=CARTESIAN_POINT('Ctrl Pts',(10.0375219932378,-26.346401824859,1.14551477168157));
#4592=CARTESIAN_POINT('Ctrl Pts',(10.3376017974799,-26.4205864987542,0.976082217833403));
#4593=CARTESIAN_POINT('Ctrl Pts',(10.637681601722,-26.4947711726494,0.80664966398524));
#4594=CARTESIAN_POINT('Ctrl Pts',(10.8549896241619,-26.6167441570493,0.557333680706485));
#4595=CARTESIAN_POINT('Ctrl Pts',(11.0722976466018,-26.7387171414493,0.308017697427731));
#4596=CARTESIAN_POINT('Ctrl Pts',(11.1850143251652,-26.9210759663912,0.0281983728666177));
#4597=CARTESIAN_POINT('Ctrl Pts',(11.2977310037287,-27.1034347913331,-0.251620951694495));
#4598=CARTESIAN_POINT('Ctrl Pts',(11.304752374725,-27.346816830551,-0.506521968549832));
#4599=CARTESIAN_POINT('Ctrl Pts',(11.3117737457213,-27.5901988697689,-0.761422985405168));
#4600=CARTESIAN_POINT('Ctrl Pts',(11.2329300973912,-27.8831551010089,-0.940919422010711));
#4601=CARTESIAN_POINT('Ctrl Pts',(11.1540864490611,-28.1761113322489,-1.12041585861625));
#4602=CARTESIAN_POINT('Ctrl Pts',(11.0262146897884,-28.4973739565395,-1.18895624432295));
#4603=CARTESIAN_POINT('Ctrl Pts',(10.8983429305156,-28.8186365808301,-1.25749663002964));
#4604=CARTESIAN_POINT('Ctrl Pts',(10.7679905873463,-29.141331370901,-1.2015057008556));
#4605=CARTESIAN_POINT('Ctrl Pts',(10.6376382441771,-29.4640261609719,-1.14551477168157));
#4606=CARTESIAN_POINT('Ctrl Pts',(10.5518441542207,-29.7609952315558,-0.976082217833403));
#4607=CARTESIAN_POINT('Ctrl Pts',(10.4660500642643,-30.0579643021397,-0.80664966398524));
#4608=CARTESIAN_POINT('Ctrl Pts',(10.4630277561102,-30.3071450622188,-0.557333680706485));
#4609=CARTESIAN_POINT('Ctrl Pts',(10.460005447956,-30.5563258222979,-0.30801769742773));
#4610=CARTESIAN_POINT('Ctrl Pts',(10.5615744836783,-30.745120741835,-0.0281983728666175));
#4611=CARTESIAN_POINT('Ctrl Pts',(10.6631435194005,-30.9339156613721,0.251620951694495));
#4612=CARTESIAN_POINT('Ctrl Pts',(10.8704078626899,-31.0616873666333,0.506521968549832));
#4613=CARTESIAN_POINT('Ctrl Pts',(11.0776722059793,-31.1894590718944,0.761422985405168));
#4614=CARTESIAN_POINT('Ctrl Pts',(11.3708015685951,-31.2676565851335,0.940919422010711));
#4615=CARTESIAN_POINT('Ctrl Pts',(11.6639309312109,-31.3458540983726,1.12041585861625));
#4616=CARTESIAN_POINT('Ctrl Pts',(12.0060884047694,-31.395745218561,1.18895624432295));
#4617=CARTESIAN_POINT('Ctrl Pts',(12.3482458783279,-31.4456363387495,1.25749663002964));
#4618=CARTESIAN_POINT('Ctrl Pts',(12.6928839357829,-31.4940952931576,1.2015057008556));
#4619=CARTESIAN_POINT('Ctrl Pts',(13.0375219932378,-31.5425542475657,1.14551477168157));
#4620=CARTESIAN_POINT('Ctrl Pts',(13.3376017974799,-31.6167389214609,0.976082217833403));
#4621=CARTESIAN_POINT('Ctrl Pts',(13.637681601722,-31.690923595356,0.80664966398524));
#4622=CARTESIAN_POINT('Ctrl Pts',(13.8549896241619,-31.812896579756,0.557333680706485));
#4623=CARTESIAN_POINT('Ctrl Pts',(14.0722976466017,-31.934869564156,0.308017697427731));
#4624=CARTESIAN_POINT('Ctrl Pts',(14.1850143251652,-32.1172283890979,0.0281983728666177));
#4625=CARTESIAN_POINT('Ctrl Pts',(14.2977310037287,-32.2995872140398,-0.251620951694495));
#4626=CARTESIAN_POINT('Ctrl Pts',(14.304752374725,-32.5429692532577,-0.506521968549832));
#4627=CARTESIAN_POINT('Ctrl Pts',(14.3117737457213,-32.7863512924756,-0.761422985405168));
#4628=CARTESIAN_POINT('Ctrl Pts',(14.2329300973912,-33.0793075237155,-0.940919422010711));
#4629=CARTESIAN_POINT('Ctrl Pts',(14.1540864490611,-33.3722637549555,-1.12041585861625));
#4630=CARTESIAN_POINT('Ctrl Pts',(14.0262146897883,-33.6935263792461,-1.18895624432295));
#4631=CARTESIAN_POINT('Ctrl Pts',(13.8983429305155,-34.0147890035367,-1.25749663002964));
#4632=CARTESIAN_POINT('Ctrl Pts',(13.7679905873463,-34.3374837936076,-1.2015057008556));
#4633=CARTESIAN_POINT('Ctrl Pts',(13.6376382441771,-34.6601785836786,-1.14551477168157));
#4634=CARTESIAN_POINT('Ctrl Pts',(13.5518441542207,-34.9571476542625,-0.976082217833403));
#4635=CARTESIAN_POINT('Ctrl Pts',(13.4660500642643,-35.2541167248464,-0.80664966398524));
#4636=CARTESIAN_POINT('Ctrl Pts',(13.4630277561101,-35.5032974849254,-0.557333680706485));
#4637=CARTESIAN_POINT('Ctrl Pts',(13.460005447956,-35.7524782450045,-0.30801769742773));
#4638=CARTESIAN_POINT('Ctrl Pts',(13.5615744836782,-35.9412731645416,-0.0281983728666175));
#4639=CARTESIAN_POINT('Ctrl Pts',(13.6631435194005,-36.1300680840788,0.251620951694495));
#4640=CARTESIAN_POINT('Ctrl Pts',(13.8704078626899,-36.2578397893399,0.506521968549832));
#4641=CARTESIAN_POINT('Ctrl Pts',(14.0776722059793,-36.3856114946011,0.761422985405168));
#4642=CARTESIAN_POINT('Ctrl Pts',(14.3708015685951,-36.4638090078402,0.940919422010711));
#4643=CARTESIAN_POINT('Ctrl Pts',(14.6639309312109,-36.5420065210792,1.12041585861625));
#4644=CARTESIAN_POINT('Ctrl Pts',(15.0060884047694,-36.5918976412677,1.18895624432295));
#4645=CARTESIAN_POINT('Ctrl Pts',(15.3482458783279,-36.6417887614562,1.25749663002964));
#4646=CARTESIAN_POINT('Ctrl Pts',(15.6928839357828,-36.6902477158643,1.2015057008556));
#4647=CARTESIAN_POINT('Ctrl Pts',(16.0375219932378,-36.7387066702723,1.14551477168157));
#4648=CARTESIAN_POINT('Ctrl Pts',(16.3376017974799,-36.8128913441675,0.976082217833403));
#4649=CARTESIAN_POINT('Ctrl Pts',(16.637681601722,-36.8870760180627,0.80664966398524));
#4650=CARTESIAN_POINT('Ctrl Pts',(16.8549896241618,-37.0090490024626,0.557333680706485));
#4651=CARTESIAN_POINT('Ctrl Pts',(17.0722976466017,-37.1310219868626,0.308017697427731));
#4652=CARTESIAN_POINT('Ctrl Pts',(17.1850143251652,-37.3133808118045,0.0281983728666177));
#4653=CARTESIAN_POINT('Ctrl Pts',(17.2977310037287,-37.4957396367464,-0.251620951694495));
#4654=CARTESIAN_POINT('Ctrl Pts',(17.304752374725,-37.7391216759643,-0.506521968549832));
#4655=CARTESIAN_POINT('Ctrl Pts',(17.3117737457213,-37.9825037151822,-0.761422985405168));
#4656=CARTESIAN_POINT('Ctrl Pts',(17.2329300973912,-38.2754599464222,-0.940919422010711));
#4657=CARTESIAN_POINT('Ctrl Pts',(17.1540864490611,-38.5684161776622,-1.12041585861625));
#4658=CARTESIAN_POINT('Ctrl Pts',(17.0262146897883,-38.8896788019527,-1.18895624432295));
#4659=CARTESIAN_POINT('Ctrl Pts',(16.8983429305155,-39.2109414262433,-1.25749663002964));
#4660=CARTESIAN_POINT('Ctrl Pts',(16.7679905873463,-39.5336362163143,-1.2015057008556));
#4661=CARTESIAN_POINT('Ctrl Pts',(16.637638244177,-39.8563310063852,-1.14551477168157));
#4662=CARTESIAN_POINT('Ctrl Pts',(16.5518441542207,-40.1533000769691,-0.976082217833403));
#4663=CARTESIAN_POINT('Ctrl Pts',(16.4660500642643,-40.450269147553,-0.80664966398524));
#4664=CARTESIAN_POINT('Ctrl Pts',(16.4630277561101,-40.6994499076321,-0.557333680706485));
#4665=CARTESIAN_POINT('Ctrl Pts',(16.460005447956,-40.9486306677112,-0.30801769742773));
#4666=CARTESIAN_POINT('Ctrl Pts',(16.5615744836782,-41.1374255872483,-0.0281983728666175));
#4667=CARTESIAN_POINT('Ctrl Pts',(16.6631435194004,-41.3262205067854,0.251620951694495));
#4668=CARTESIAN_POINT('Ctrl Pts',(16.8704078626898,-41.4539922120466,0.506521968549832));
#4669=CARTESIAN_POINT('Ctrl Pts',(17.0776722059792,-41.5817639173077,0.761422985405168));
#4670=CARTESIAN_POINT('Ctrl Pts',(17.370801568595,-41.6599614305468,0.940919422010711));
#4671=CARTESIAN_POINT('Ctrl Pts',(17.6639309312109,-41.7381589437859,1.12041585861625));
#4672=CARTESIAN_POINT('Ctrl Pts',(18.0060884047694,-41.7880500639744,1.18895624432295));
#4673=CARTESIAN_POINT('Ctrl Pts',(18.3482458783279,-41.8379411841628,1.25749663002964));
#4674=CARTESIAN_POINT('Ctrl Pts',(18.6928839357828,-41.8864001385709,1.2015057008556));
#4675=CARTESIAN_POINT('Ctrl Pts',(19.0375219932377,-41.934859092979,1.14551477168157));
#4676=CARTESIAN_POINT('Ctrl Pts',(19.3376017974798,-42.0090437668742,0.976082217833403));
#4677=CARTESIAN_POINT('Ctrl Pts',(19.6376816017219,-42.0832284407693,0.80664966398524));
#4678=CARTESIAN_POINT('Ctrl Pts',(19.8549896241618,-42.2052014251693,0.557333680706485));
#4679=CARTESIAN_POINT('Ctrl Pts',(20.0722976466017,-42.3271744095693,0.308017697427731));
#4680=CARTESIAN_POINT('Ctrl Pts',(20.1850143251651,-42.5095332345112,0.0281983728666177));
#4681=CARTESIAN_POINT('Ctrl Pts',(20.2977310037286,-42.6918920594531,-0.251620951694495));
#4682=CARTESIAN_POINT('Ctrl Pts',(20.3047523747249,-42.935274098671,-0.506521968549832));
#4683=CARTESIAN_POINT('Ctrl Pts',(20.3117737457212,-43.1786561378889,-0.761422985405168));
#4684=CARTESIAN_POINT('Ctrl Pts',(20.2329300973911,-43.4716123691288,-0.940919422010711));
#4685=CARTESIAN_POINT('Ctrl Pts',(20.154086449061,-43.7645686003688,-1.12041585861625));
#4686=CARTESIAN_POINT('Ctrl Pts',(20.0262146897883,-44.0858312246594,-1.18895624432295));
#4687=CARTESIAN_POINT('Ctrl Pts',(19.8983429305155,-44.40709384895,-1.25749663002964));
#4688=CARTESIAN_POINT('Ctrl Pts',(19.7679905873462,-44.7297886390209,-1.2015057008556));
#4689=CARTESIAN_POINT('Ctrl Pts',(19.637638244177,-45.0524834290919,-1.14551477168157));
#4690=CARTESIAN_POINT('Ctrl Pts',(19.5518441542206,-45.3494524996758,-0.976082217833403));
#4691=CARTESIAN_POINT('Ctrl Pts',(3.62216201968442,-19.1056780894973,-1.2339885196899));
#4692=CARTESIAN_POINT('Ctrl Pts',(3.48538897159447,-19.4320798752826,-0.910806095028249));
#4693=CARTESIAN_POINT('Ctrl Pts',(3.49420839053257,-19.6744238110373,-0.497425511654571));
#4694=CARTESIAN_POINT('Ctrl Pts',(3.50302780947066,-19.916767746792,-0.0840449282808927));
#4695=CARTESIAN_POINT('Ctrl Pts',(3.67691385823109,-20.0638104193845,0.337658719487502));
#4696=CARTESIAN_POINT('Ctrl Pts',(3.85079990699151,-20.2108530919771,0.759362367255897));
#4697=CARTESIAN_POINT('Ctrl Pts',(4.17653327792288,-20.2702266722385,1.10586550012264));
#4698=CARTESIAN_POINT('Ctrl Pts',(4.50226664885425,-20.3296002524999,1.45236863298939));
#4699=CARTESIAN_POINT('Ctrl Pts',(4.93655280986403,-20.3263008501883,1.65504205590818));
#4700=CARTESIAN_POINT('Ctrl Pts',(5.3708389708738,-20.3230014478767,1.85771547882697));
#4701=CARTESIAN_POINT('Ctrl Pts',(5.84888317848182,-20.2944383255823,1.87641723476232));
#4702=CARTESIAN_POINT('Ctrl Pts',(6.32692738608983,-20.265875203288,1.89511899069768));
#4703=CARTESIAN_POINT('Ctrl Pts',(6.77526807902992,-20.2544614131831,1.72614496752462));
#4704=CARTESIAN_POINT('Ctrl Pts',(7.22360877197,-20.2430476230782,1.55717094435156));
#4705=CARTESIAN_POINT('Ctrl Pts',(7.57466753434566,-20.2877995817719,1.2339885196899));
#4706=CARTESIAN_POINT('Ctrl Pts',(7.92572629672132,-20.3325515404656,0.910806095028249));
#4707=CARTESIAN_POINT('Ctrl Pts',(8.13119259206894,-20.46136134919,0.497425511654571));
#4708=CARTESIAN_POINT('Ctrl Pts',(8.33665888741656,-20.5901711579143,0.084044928280893));
#4709=CARTESIAN_POINT('Ctrl Pts',(8.37705855294184,-20.8142822298008,-0.337658719487502));
#4710=CARTESIAN_POINT('Ctrl Pts',(8.41745821846713,-21.0383933016873,-0.759362367255897));
#4711=CARTESIAN_POINT('Ctrl Pts',(8.30601056182147,-21.350173465905,-1.10586550012264));
#4712=CARTESIAN_POINT('Ctrl Pts',(8.19456290517582,-21.6619536301226,-1.45236863298939));
#4713=CARTESIAN_POINT('Ctrl Pts',(7.97456245845175,-22.0364067769132,-1.65504205590818));
#4714=CARTESIAN_POINT('Ctrl Pts',(7.75456201172769,-22.4108599237039,-1.85771547882697));
#4715=CARTESIAN_POINT('Ctrl Pts',(7.49080351840538,-22.8105767904773,-1.87641723476232));
#4716=CARTESIAN_POINT('Ctrl Pts',(7.22704502508308,-23.2102936572507,-1.89511899069768));
#4717=CARTESIAN_POINT('Ctrl Pts',(6.99299004642871,-23.5928611918346,-1.72614496752462));
#4718=CARTESIAN_POINT('Ctrl Pts',(6.75893506777434,-23.9754287264186,-1.55717094435156));
#4719=CARTESIAN_POINT('Ctrl Pts',(6.62216201968439,-24.3018305122039,-1.2339885196899));
#4720=CARTESIAN_POINT('Ctrl Pts',(6.48538897159444,-24.6282322979892,-0.910806095028249));
#4721=CARTESIAN_POINT('Ctrl Pts',(6.49420839053254,-24.8705762337439,-0.497425511654571));
#4722=CARTESIAN_POINT('Ctrl Pts',(6.50302780947063,-25.1129201694986,-0.0840449282808927));
#4723=CARTESIAN_POINT('Ctrl Pts',(6.67691385823105,-25.2599628420912,0.337658719487502));
#4724=CARTESIAN_POINT('Ctrl Pts',(6.85079990699148,-25.4070055146837,0.759362367255897));
#4725=CARTESIAN_POINT('Ctrl Pts',(7.17653327792285,-25.4663790949451,1.10586550012264));
#4726=CARTESIAN_POINT('Ctrl Pts',(7.50226664885422,-25.5257526752066,1.45236863298939));
#4727=CARTESIAN_POINT('Ctrl Pts',(7.936552809864,-25.5224532728949,1.65504205590818));
#4728=CARTESIAN_POINT('Ctrl Pts',(8.37083897087377,-25.5191538705833,1.85771547882697));
#4729=CARTESIAN_POINT('Ctrl Pts',(8.84888317848179,-25.490590748289,1.87641723476232));
#4730=CARTESIAN_POINT('Ctrl Pts',(9.3269273860898,-25.4620276259946,1.89511899069768));
#4731=CARTESIAN_POINT('Ctrl Pts',(9.77526807902988,-25.4506138358897,1.72614496752462));
#4732=CARTESIAN_POINT('Ctrl Pts',(10.22360877197,-25.4392000457848,1.55717094435156));
#4733=CARTESIAN_POINT('Ctrl Pts',(10.5746675343456,-25.4839520044785,1.2339885196899));
#4734=CARTESIAN_POINT('Ctrl Pts',(10.9257262967213,-25.5287039631723,0.910806095028249));
#4735=CARTESIAN_POINT('Ctrl Pts',(11.1311925920689,-25.6575137718966,0.497425511654571));
#4736=CARTESIAN_POINT('Ctrl Pts',(11.3366588874165,-25.786323580621,0.084044928280893));
#4737=CARTESIAN_POINT('Ctrl Pts',(11.3770585529418,-26.0104346525075,-0.337658719487502));
#4738=CARTESIAN_POINT('Ctrl Pts',(11.4174582184671,-26.234545724394,-0.759362367255897));
#4739=CARTESIAN_POINT('Ctrl Pts',(11.3060105618214,-26.5463258886116,-1.10586550012264));
#4740=CARTESIAN_POINT('Ctrl Pts',(11.1945629051758,-26.8581060528292,-1.45236863298939));
#4741=CARTESIAN_POINT('Ctrl Pts',(10.9745624584517,-27.2325591996199,-1.65504205590818));
#4742=CARTESIAN_POINT('Ctrl Pts',(10.7545620117277,-27.6070123464106,-1.85771547882697));
#4743=CARTESIAN_POINT('Ctrl Pts',(10.4908035184054,-28.0067292131839,-1.87641723476232));
#4744=CARTESIAN_POINT('Ctrl Pts',(10.227045025083,-28.4064460799573,-1.89511899069768));
#4745=CARTESIAN_POINT('Ctrl Pts',(9.99299004642868,-28.7890136145413,-1.72614496752462));
#4746=CARTESIAN_POINT('Ctrl Pts',(9.75893506777431,-29.1715811491253,-1.55717094435156));
#4747=CARTESIAN_POINT('Ctrl Pts',(9.62216201968436,-29.4979829349106,-1.2339885196899));
#4748=CARTESIAN_POINT('Ctrl Pts',(9.48538897159441,-29.8243847206959,-0.910806095028249));
#4749=CARTESIAN_POINT('Ctrl Pts',(9.4942083905325,-30.0667286564506,-0.497425511654571));
#4750=CARTESIAN_POINT('Ctrl Pts',(9.5030278094706,-30.3090725922053,-0.0840449282808927));
#4751=CARTESIAN_POINT('Ctrl Pts',(9.67691385823102,-30.4561152647978,0.337658719487502));
#4752=CARTESIAN_POINT('Ctrl Pts',(9.85079990699145,-30.6031579373903,0.759362367255897));
#4753=CARTESIAN_POINT('Ctrl Pts',(10.1765332779228,-30.6625315176518,1.10586550012264));
#4754=CARTESIAN_POINT('Ctrl Pts',(10.5022666488542,-30.7219050979132,1.45236863298939));
#4755=CARTESIAN_POINT('Ctrl Pts',(10.936552809864,-30.7186056956016,1.65504205590818));
#4756=CARTESIAN_POINT('Ctrl Pts',(11.3708389708737,-30.71530629329,1.85771547882697));
#4757=CARTESIAN_POINT('Ctrl Pts',(11.8488831784818,-30.6867431709956,1.87641723476232));
#4758=CARTESIAN_POINT('Ctrl Pts',(12.3269273860898,-30.6581800487013,1.89511899069768));
#4759=CARTESIAN_POINT('Ctrl Pts',(12.7752680790299,-30.6467662585964,1.72614496752462));
#4760=CARTESIAN_POINT('Ctrl Pts',(13.2236087719699,-30.6353524684915,1.55717094435156));
#4761=CARTESIAN_POINT('Ctrl Pts',(13.5746675343456,-30.6801044271852,1.2339885196899));
#4762=CARTESIAN_POINT('Ctrl Pts',(13.9257262967213,-30.7248563858789,0.910806095028249));
#4763=CARTESIAN_POINT('Ctrl Pts',(14.1311925920689,-30.8536661946033,0.497425511654571));
#4764=CARTESIAN_POINT('Ctrl Pts',(14.3366588874165,-30.9824760033276,0.084044928280893));
#4765=CARTESIAN_POINT('Ctrl Pts',(14.3770585529418,-31.2065870752141,-0.337658719487502));
#4766=CARTESIAN_POINT('Ctrl Pts',(14.4174582184671,-31.4306981471006,-0.759362367255897));
#4767=CARTESIAN_POINT('Ctrl Pts',(14.3060105618214,-31.7424783113183,-1.10586550012264));
#4768=CARTESIAN_POINT('Ctrl Pts',(14.1945629051758,-32.0542584755359,-1.45236863298939));
#4769=CARTESIAN_POINT('Ctrl Pts',(13.9745624584517,-32.4287116223265,-1.65504205590818));
#4770=CARTESIAN_POINT('Ctrl Pts',(13.7545620117276,-32.8031647691172,-1.85771547882697));
#4771=CARTESIAN_POINT('Ctrl Pts',(13.4908035184053,-33.2028816358906,-1.87641723476232));
#4772=CARTESIAN_POINT('Ctrl Pts',(13.227045025083,-33.602598502664,-1.89511899069768));
#4773=CARTESIAN_POINT('Ctrl Pts',(12.9929900464286,-33.9851660372479,-1.72614496752462));
#4774=CARTESIAN_POINT('Ctrl Pts',(12.7589350677743,-34.3677335718319,-1.55717094435156));
#4775=CARTESIAN_POINT('Ctrl Pts',(12.6221620196843,-34.6941353576172,-1.2339885196899));
#4776=CARTESIAN_POINT('Ctrl Pts',(12.4853889715944,-35.0205371434025,-0.910806095028249));
#4777=CARTESIAN_POINT('Ctrl Pts',(12.4942083905325,-35.2628810791572,-0.497425511654571));
#4778=CARTESIAN_POINT('Ctrl Pts',(12.5030278094706,-35.5052250149119,-0.0840449282808927));
#4779=CARTESIAN_POINT('Ctrl Pts',(12.676913858231,-35.6522676875044,0.337658719487502));
#4780=CARTESIAN_POINT('Ctrl Pts',(12.8507999069914,-35.799310360097,0.759362367255897));
#4781=CARTESIAN_POINT('Ctrl Pts',(13.1765332779228,-35.8586839403584,1.10586550012264));
#4782=CARTESIAN_POINT('Ctrl Pts',(13.5022666488542,-35.9180575206199,1.45236863298939));
#4783=CARTESIAN_POINT('Ctrl Pts',(13.9365528098639,-35.9147581183082,1.65504205590818));
#4784=CARTESIAN_POINT('Ctrl Pts',(14.3708389708737,-35.9114587159966,1.85771547882697));
#4785=CARTESIAN_POINT('Ctrl Pts',(14.8488831784817,-35.8828955937023,1.87641723476232));
#4786=CARTESIAN_POINT('Ctrl Pts',(15.3269273860897,-35.8543324714079,1.89511899069768));
#4787=CARTESIAN_POINT('Ctrl Pts',(15.7752680790298,-35.842918681303,1.72614496752462));
#4788=CARTESIAN_POINT('Ctrl Pts',(16.2236087719699,-35.8315048911981,1.55717094435156));
#4789=CARTESIAN_POINT('Ctrl Pts',(16.5746675343456,-35.8762568498918,1.2339885196899));
#4790=CARTESIAN_POINT('Ctrl Pts',(16.9257262967212,-35.9210088085856,0.910806095028249));
#4791=CARTESIAN_POINT('Ctrl Pts',(17.1311925920688,-36.0498186173099,0.497425511654571));
#4792=CARTESIAN_POINT('Ctrl Pts',(17.3366588874165,-36.1786284260343,0.084044928280893));
#4793=CARTESIAN_POINT('Ctrl Pts',(17.3770585529417,-36.4027394979208,-0.337658719487502));
#4794=CARTESIAN_POINT('Ctrl Pts',(17.417458218467,-36.6268505698073,-0.759362367255897));
#4795=CARTESIAN_POINT('Ctrl Pts',(17.3060105618214,-36.9386307340249,-1.10586550012264));
#4796=CARTESIAN_POINT('Ctrl Pts',(17.1945629051757,-37.2504108982425,-1.45236863298939));
#4797=CARTESIAN_POINT('Ctrl Pts',(16.9745624584517,-37.6248640450332,-1.65504205590818));
#4798=CARTESIAN_POINT('Ctrl Pts',(16.7545620117276,-37.9993171918239,-1.85771547882697));
#4799=CARTESIAN_POINT('Ctrl Pts',(16.4908035184053,-38.3990340585972,-1.87641723476232));
#4800=CARTESIAN_POINT('Ctrl Pts',(16.227045025083,-38.7987509253706,-1.89511899069768));
#4801=CARTESIAN_POINT('Ctrl Pts',(15.9929900464286,-39.1813184599546,-1.72614496752462));
#4802=CARTESIAN_POINT('Ctrl Pts',(15.7589350677742,-39.5638859945386,-1.55717094435156));
#4803=CARTESIAN_POINT('Ctrl Pts',(15.6221620196843,-39.8902877803239,-1.2339885196899));
#4804=CARTESIAN_POINT('Ctrl Pts',(15.4853889715943,-40.2166895661092,-0.910806095028249));
#4805=CARTESIAN_POINT('Ctrl Pts',(15.4942083905324,-40.4590335018639,-0.497425511654571));
#4806=CARTESIAN_POINT('Ctrl Pts',(15.5030278094705,-40.7013774376186,-0.0840449282808927));
#4807=CARTESIAN_POINT('Ctrl Pts',(15.676913858231,-40.8484201102111,0.337658719487502));
#4808=CARTESIAN_POINT('Ctrl Pts',(15.8507999069914,-40.9954627828037,0.759362367255897));
#4809=CARTESIAN_POINT('Ctrl Pts',(16.1765332779228,-41.0548363630651,1.10586550012264));
#4810=CARTESIAN_POINT('Ctrl Pts',(16.5022666488541,-41.1142099433265,1.45236863298939));
#4811=CARTESIAN_POINT('Ctrl Pts',(16.9365528098639,-41.1109105410149,1.65504205590818));
#4812=CARTESIAN_POINT('Ctrl Pts',(17.3708389708737,-41.1076111387033,1.85771547882697));
#4813=CARTESIAN_POINT('Ctrl Pts',(17.8488831784817,-41.0790480164089,1.87641723476232));
#4814=CARTESIAN_POINT('Ctrl Pts',(18.3269273860897,-41.0504848941146,1.89511899069768));
#4815=CARTESIAN_POINT('Ctrl Pts',(18.7752680790298,-41.0390711040097,1.72614496752462));
#4816=CARTESIAN_POINT('Ctrl Pts',(19.2236087719699,-41.0276573139048,1.55717094435156));
#4817=CARTESIAN_POINT('Ctrl Pts',(19.5746675343455,-41.0724092725985,1.2339885196899));
#4818=CARTESIAN_POINT('Ctrl Pts',(19.9257262967212,-41.1171612312922,0.910806095028249));
#4819=CARTESIAN_POINT('Ctrl Pts',(20.1311925920688,-41.2459710400166,0.497425511654571));
#4820=CARTESIAN_POINT('Ctrl Pts',(20.3366588874164,-41.374780848741,0.084044928280893));
#4821=CARTESIAN_POINT('Ctrl Pts',(20.3770585529417,-41.5988919206274,-0.337658719487502));
#4822=CARTESIAN_POINT('Ctrl Pts',(20.417458218467,-41.823002992514,-0.759362367255897));
#4823=CARTESIAN_POINT('Ctrl Pts',(20.3060105618213,-42.1347831567316,-1.10586550012264));
#4824=CARTESIAN_POINT('Ctrl Pts',(20.1945629051757,-42.4465633209492,-1.45236863298939));
#4825=CARTESIAN_POINT('Ctrl Pts',(19.9745624584516,-42.8210164677398,-1.65504205590818));
#4826=CARTESIAN_POINT('Ctrl Pts',(19.7545620117276,-43.1954696145305,-1.85771547882697));
#4827=CARTESIAN_POINT('Ctrl Pts',(19.4908035184053,-43.5951864813039,-1.87641723476232));
#4828=CARTESIAN_POINT('Ctrl Pts',(19.227045025083,-43.9949033480773,-1.89511899069768));
#4829=CARTESIAN_POINT('Ctrl Pts',(18.9929900464286,-44.3774708826612,-1.72614496752462));
#4830=CARTESIAN_POINT('Ctrl Pts',(18.7589350677742,-44.7600384172452,-1.55717094435156));
#4831=CARTESIAN_POINT('Ctrl Pts',(18.6221620196843,-45.0864402030305,-1.2339885196899));
#4832=CARTESIAN_POINT('Ctrl Pts',(2.69247988514806,-18.842665792852,-1.4918948215464));
#4833=CARTESIAN_POINT('Ctrl Pts',(2.50472787892454,-19.1985002938387,-1.01496252607126));
#4834=CARTESIAN_POINT('Ctrl Pts',(2.52538902495489,-19.434007405269,-0.437517342602656));
#4835=CARTESIAN_POINT('Ctrl Pts',(2.54605017098523,-19.6695145166993,0.139927840865946));
#4836=CARTESIAN_POINT('Ctrl Pts',(2.79225323278385,-19.7748049423473,0.703515811841622));
#4837=CARTESIAN_POINT('Ctrl Pts',(3.03845629458247,-19.8800953679953,1.2671037828173));
#4838=CARTESIAN_POINT('Ctrl Pts',(3.48265869315581,-19.871070823257,1.70520903169545));
#4839=CARTESIAN_POINT('Ctrl Pts',(3.92686109172914,-19.8620462785187,2.1433142805736));
#4840=CARTESIAN_POINT('Ctrl Pts',(4.50230405113288,-19.7772499606563,2.36916468980564));
#4841=CARTESIAN_POINT('Ctrl Pts',(5.07774701053662,-19.692453642794,2.59501509903768));
#4842=CARTESIAN_POINT('Ctrl Pts',(5.69167795219416,-19.5854362780169,2.5638782252017));
#4843=CARTESIAN_POINT('Ctrl Pts',(6.30560889385169,-19.4784189132398,2.53274135136572));
#4844=CARTESIAN_POINT('Ctrl Pts',(6.85765222227691,-19.4071323786218,2.25078423419363));
#4845=CARTESIAN_POINT('Ctrl Pts',(7.40969555070213,-19.3358458440039,1.96882711702155));
#4846=CARTESIAN_POINT('Ctrl Pts',(7.81173327121136,-19.3511650874962,1.4918948215464));
#4847=CARTESIAN_POINT('Ctrl Pts',(8.21377099172059,-19.3664843309885,1.01496252607126));
#4848=CARTESIAN_POINT('Ctrl Pts',(8.40739555997595,-19.5021309640373,0.437517342602656));
#4849=CARTESIAN_POINT('Ctrl Pts',(8.60102012823132,-19.637777597086,-0.139927840865945));
#4850=CARTESIAN_POINT('Ctrl Pts',(8.56910278071841,-19.9036409159171,-0.703515811841622));
#4851=CARTESIAN_POINT('Ctrl Pts',(8.5371854332055,-20.1695042347482,-1.2671037828173));
#4852=CARTESIAN_POINT('Ctrl Pts',(8.30726874891788,-20.5496825239655,-1.70520903169545));
#4853=CARTESIAN_POINT('Ctrl Pts',(8.07735206463027,-20.9298608131829,-2.1433142805736));
#4854=CARTESIAN_POINT('Ctrl Pts',(7.71619481951224,-21.3858108755242,-2.36916468980564));
#4855=CARTESIAN_POINT('Ctrl Pts',(7.35503757439421,-21.8417609378656,-2.59501509903768));
#4856=CARTESIAN_POINT('Ctrl Pts',(6.95539234702238,-22.3199320471218,-2.5638782252017));
#4857=CARTESIAN_POINT('Ctrl Pts',(6.55574711965056,-22.7981031563779,-2.53274135136572));
#4858=CARTESIAN_POINT('Ctrl Pts',(6.21798950551105,-23.2405434354749,-2.25078423419363));
#4859=CARTESIAN_POINT('Ctrl Pts',(5.88023189137154,-23.6829837145719,-1.96882711702155));
#4860=CARTESIAN_POINT('Ctrl Pts',(5.69247988514803,-24.0388182155586,-1.4918948215464));
#4861=CARTESIAN_POINT('Ctrl Pts',(5.50472787892451,-24.3946527165454,-1.01496252607126));
#4862=CARTESIAN_POINT('Ctrl Pts',(5.52538902495486,-24.6301598279757,-0.437517342602656));
#4863=CARTESIAN_POINT('Ctrl Pts',(5.5460501709852,-24.865666939406,0.139927840865946));
#4864=CARTESIAN_POINT('Ctrl Pts',(5.79225323278382,-24.970957365054,0.703515811841622));
#4865=CARTESIAN_POINT('Ctrl Pts',(6.03845629458244,-25.0762477907019,1.2671037828173));
#4866=CARTESIAN_POINT('Ctrl Pts',(6.48265869315577,-25.0672232459636,1.70520903169545));
#4867=CARTESIAN_POINT('Ctrl Pts',(6.92686109172911,-25.0581987012253,2.1433142805736));
#4868=CARTESIAN_POINT('Ctrl Pts',(7.50230405113285,-24.973402383363,2.36916468980564));
#4869=CARTESIAN_POINT('Ctrl Pts',(8.07774701053659,-24.8886060655007,2.59501509903768));
#4870=CARTESIAN_POINT('Ctrl Pts',(8.69167795219413,-24.7815887007236,2.5638782252017));
#4871=CARTESIAN_POINT('Ctrl Pts',(9.30560889385166,-24.6745713359464,2.53274135136572));
#4872=CARTESIAN_POINT('Ctrl Pts',(9.85765222227688,-24.6032848013285,2.25078423419363));
#4873=CARTESIAN_POINT('Ctrl Pts',(10.4096955507021,-24.5319982667106,1.96882711702155));
#4874=CARTESIAN_POINT('Ctrl Pts',(10.8117332712113,-24.5473175102029,1.4918948215464));
#4875=CARTESIAN_POINT('Ctrl Pts',(11.2137709917206,-24.5626367536952,1.01496252607126));
#4876=CARTESIAN_POINT('Ctrl Pts',(11.4073955599759,-24.6982833867439,0.437517342602656));
#4877=CARTESIAN_POINT('Ctrl Pts',(11.6010201282313,-24.8339300197927,-0.139927840865945));
#4878=CARTESIAN_POINT('Ctrl Pts',(11.5691027807184,-25.0997933386238,-0.703515811841622));
#4879=CARTESIAN_POINT('Ctrl Pts',(11.5371854332055,-25.3656566574548,-1.2671037828173));
#4880=CARTESIAN_POINT('Ctrl Pts',(11.3072687489179,-25.7458349466722,-1.70520903169545));
#4881=CARTESIAN_POINT('Ctrl Pts',(11.0773520646302,-26.1260132358895,-2.1433142805736));
#4882=CARTESIAN_POINT('Ctrl Pts',(10.7161948195122,-26.5819632982309,-2.36916468980564));
#4883=CARTESIAN_POINT('Ctrl Pts',(10.3550375743942,-27.0379133605723,-2.59501509903768));
#4884=CARTESIAN_POINT('Ctrl Pts',(9.95539234702235,-27.5160844698284,-2.5638782252017));
#4885=CARTESIAN_POINT('Ctrl Pts',(9.55574711965053,-27.9942555790846,-2.53274135136572));
#4886=CARTESIAN_POINT('Ctrl Pts',(9.21798950551102,-28.4366958581816,-2.25078423419363));
#4887=CARTESIAN_POINT('Ctrl Pts',(8.88023189137151,-28.8791361372786,-1.96882711702155));
#4888=CARTESIAN_POINT('Ctrl Pts',(8.692479885148,-29.2349706382653,-1.4918948215464));
#4889=CARTESIAN_POINT('Ctrl Pts',(8.50472787892448,-29.590805139252,-1.01496252607126));
#4890=CARTESIAN_POINT('Ctrl Pts',(8.52538902495483,-29.8263122506823,-0.437517342602656));
#4891=CARTESIAN_POINT('Ctrl Pts',(8.54605017098517,-30.0618193621126,0.139927840865946));
#4892=CARTESIAN_POINT('Ctrl Pts',(8.79225323278379,-30.1671097877606,0.703515811841622));
#4893=CARTESIAN_POINT('Ctrl Pts',(9.03845629458241,-30.2724002134086,1.2671037828173));
#4894=CARTESIAN_POINT('Ctrl Pts',(9.48265869315574,-30.2633756686703,1.70520903169545));
#4895=CARTESIAN_POINT('Ctrl Pts',(9.92686109172908,-30.254351123932,2.1433142805736));
#4896=CARTESIAN_POINT('Ctrl Pts',(10.5023040511328,-30.1695548060697,2.36916468980564));
#4897=CARTESIAN_POINT('Ctrl Pts',(11.0777470105366,-30.0847584882073,2.59501509903768));
#4898=CARTESIAN_POINT('Ctrl Pts',(11.6916779521941,-29.9777411234302,2.5638782252017));
#4899=CARTESIAN_POINT('Ctrl Pts',(12.3056088938516,-29.8707237586531,2.53274135136572));
#4900=CARTESIAN_POINT('Ctrl Pts',(12.8576522222768,-29.7994372240352,2.25078423419363));
#4901=CARTESIAN_POINT('Ctrl Pts',(13.4096955507021,-29.7281506894172,1.96882711702155));
#4902=CARTESIAN_POINT('Ctrl Pts',(13.8117332712113,-29.7434699329095,1.4918948215464));
#4903=CARTESIAN_POINT('Ctrl Pts',(14.2137709917205,-29.7587891764018,1.01496252607126));
#4904=CARTESIAN_POINT('Ctrl Pts',(14.4073955599759,-29.8944358094506,0.437517342602656));
#4905=CARTESIAN_POINT('Ctrl Pts',(14.6010201282313,-30.0300824424993,-0.139927840865945));
#4906=CARTESIAN_POINT('Ctrl Pts',(14.5691027807183,-30.2959457613304,-0.703515811841622));
#4907=CARTESIAN_POINT('Ctrl Pts',(14.5371854332054,-30.5618090801615,-1.2671037828173));
#4908=CARTESIAN_POINT('Ctrl Pts',(14.3072687489178,-30.9419873693788,-1.70520903169545));
#4909=CARTESIAN_POINT('Ctrl Pts',(14.0773520646302,-31.3221656585962,-2.1433142805736));
#4910=CARTESIAN_POINT('Ctrl Pts',(13.7161948195122,-31.7781157209375,-2.36916468980564));
#4911=CARTESIAN_POINT('Ctrl Pts',(13.3550375743941,-32.2340657832789,-2.59501509903768));
#4912=CARTESIAN_POINT('Ctrl Pts',(12.9553923470223,-32.7122368925351,-2.5638782252017));
#4913=CARTESIAN_POINT('Ctrl Pts',(12.5557471196505,-33.1904080017912,-2.53274135136572));
#4914=CARTESIAN_POINT('Ctrl Pts',(12.217989505511,-33.6328482808882,-2.25078423419363));
#4915=CARTESIAN_POINT('Ctrl Pts',(11.8802318913715,-34.0752885599852,-1.96882711702155));
#4916=CARTESIAN_POINT('Ctrl Pts',(11.692479885148,-34.4311230609719,-1.4918948215464));
#4917=CARTESIAN_POINT('Ctrl Pts',(11.5047278789244,-34.7869575619587,-1.01496252607126));
#4918=CARTESIAN_POINT('Ctrl Pts',(11.5253890249548,-35.022464673389,-0.437517342602656));
#4919=CARTESIAN_POINT('Ctrl Pts',(11.5460501709851,-35.2579717848193,0.139927840865946));
#4920=CARTESIAN_POINT('Ctrl Pts',(11.7922532327838,-35.3632622104672,0.703515811841622));
#4921=CARTESIAN_POINT('Ctrl Pts',(12.0384562945824,-35.4685526361152,1.2671037828173));
#4922=CARTESIAN_POINT('Ctrl Pts',(12.4826586931557,-35.4595280913769,1.70520903169545));
#4923=CARTESIAN_POINT('Ctrl Pts',(12.926861091729,-35.4505035466386,2.1433142805736));
#4924=CARTESIAN_POINT('Ctrl Pts',(13.5023040511328,-35.3657072287763,2.36916468980564));
#4925=CARTESIAN_POINT('Ctrl Pts',(14.0777470105365,-35.280910910914,2.59501509903768));
#4926=CARTESIAN_POINT('Ctrl Pts',(14.6916779521941,-35.1738935461369,2.5638782252017));
#4927=CARTESIAN_POINT('Ctrl Pts',(15.3056088938516,-35.0668761813597,2.53274135136572));
#4928=CARTESIAN_POINT('Ctrl Pts',(15.8576522222768,-34.9955896467418,2.25078423419363));
#4929=CARTESIAN_POINT('Ctrl Pts',(16.409695550702,-34.9243031121239,1.96882711702155));
#4930=CARTESIAN_POINT('Ctrl Pts',(16.8117332712113,-34.9396223556162,1.4918948215464));
#4931=CARTESIAN_POINT('Ctrl Pts',(17.2137709917205,-34.9549415991085,1.01496252607126));
#4932=CARTESIAN_POINT('Ctrl Pts',(17.4073955599759,-35.0905882321572,0.437517342602656));
#4933=CARTESIAN_POINT('Ctrl Pts',(17.6010201282312,-35.226234865206,-0.139927840865945));
#4934=CARTESIAN_POINT('Ctrl Pts',(17.5691027807183,-35.4920981840371,-0.703515811841622));
#4935=CARTESIAN_POINT('Ctrl Pts',(17.5371854332054,-35.7579615028681,-1.2671037828173));
#4936=CARTESIAN_POINT('Ctrl Pts',(17.3072687489178,-36.1381397920855,-1.70520903169545));
#4937=CARTESIAN_POINT('Ctrl Pts',(17.0773520646302,-36.5183180813028,-2.1433142805736));
#4938=CARTESIAN_POINT('Ctrl Pts',(16.7161948195121,-36.9742681436442,-2.36916468980564));
#4939=CARTESIAN_POINT('Ctrl Pts',(16.3550375743941,-37.4302182059856,-2.59501509903768));
#4940=CARTESIAN_POINT('Ctrl Pts',(15.9553923470223,-37.9083893152417,-2.5638782252017));
#4941=CARTESIAN_POINT('Ctrl Pts',(15.5557471196505,-38.3865604244979,-2.53274135136572));
#4942=CARTESIAN_POINT('Ctrl Pts',(15.217989505511,-38.8290007035949,-2.25078423419363));
#4943=CARTESIAN_POINT('Ctrl Pts',(14.8802318913715,-39.2714409826919,-1.96882711702155));
#4944=CARTESIAN_POINT('Ctrl Pts',(14.6924798851479,-39.6272754836786,-1.4918948215464));
#4945=CARTESIAN_POINT('Ctrl Pts',(14.5047278789244,-39.9831099846653,-1.01496252607126));
#4946=CARTESIAN_POINT('Ctrl Pts',(14.5253890249548,-40.2186170960956,-0.437517342602656));
#4947=CARTESIAN_POINT('Ctrl Pts',(14.5460501709851,-40.4541242075259,0.139927840865946));
#4948=CARTESIAN_POINT('Ctrl Pts',(14.7922532327837,-40.5594146331739,0.703515811841622));
#4949=CARTESIAN_POINT('Ctrl Pts',(15.0384562945823,-40.6647050588219,1.2671037828173));
#4950=CARTESIAN_POINT('Ctrl Pts',(15.4826586931557,-40.6556805140836,1.70520903169545));
#4951=CARTESIAN_POINT('Ctrl Pts',(15.926861091729,-40.6466559693453,2.1433142805736));
#4952=CARTESIAN_POINT('Ctrl Pts',(16.5023040511328,-40.5618596514829,2.36916468980564));
#4953=CARTESIAN_POINT('Ctrl Pts',(17.0777470105365,-40.4770633336206,2.59501509903768));
#4954=CARTESIAN_POINT('Ctrl Pts',(17.691677952194,-40.3700459688435,2.5638782252017));
#4955=CARTESIAN_POINT('Ctrl Pts',(18.3056088938516,-40.2630286040664,2.53274135136572));
#4956=CARTESIAN_POINT('Ctrl Pts',(18.8576522222768,-40.1917420694485,2.25078423419363));
#4957=CARTESIAN_POINT('Ctrl Pts',(19.409695550702,-40.1204555348305,1.96882711702155));
#4958=CARTESIAN_POINT('Ctrl Pts',(19.8117332712112,-40.1357747783228,1.4918948215464));
#4959=CARTESIAN_POINT('Ctrl Pts',(20.2137709917205,-40.1510940218152,1.01496252607126));
#4960=CARTESIAN_POINT('Ctrl Pts',(20.4073955599758,-40.2867406548639,0.437517342602656));
#4961=CARTESIAN_POINT('Ctrl Pts',(20.6010201282312,-40.4223872879126,-0.139927840865945));
#4962=CARTESIAN_POINT('Ctrl Pts',(20.5691027807183,-40.6882506067437,-0.703515811841622));
#4963=CARTESIAN_POINT('Ctrl Pts',(20.5371854332054,-40.9541139255748,-1.2671037828173));
#4964=CARTESIAN_POINT('Ctrl Pts',(20.3072687489178,-41.3342922147921,-1.70520903169545));
#4965=CARTESIAN_POINT('Ctrl Pts',(20.0773520646301,-41.7144705040095,-2.1433142805736));
#4966=CARTESIAN_POINT('Ctrl Pts',(19.7161948195121,-42.1704205663508,-2.36916468980564));
#4967=CARTESIAN_POINT('Ctrl Pts',(19.3550375743941,-42.6263706286922,-2.59501509903768));
#4968=CARTESIAN_POINT('Ctrl Pts',(18.9553923470223,-43.1045417379484,-2.5638782252017));
#4969=CARTESIAN_POINT('Ctrl Pts',(18.5557471196504,-43.5827128472045,-2.53274135136572));
#4970=CARTESIAN_POINT('Ctrl Pts',(18.2179895055109,-44.0251531263015,-2.25078423419363));
#4971=CARTESIAN_POINT('Ctrl Pts',(17.8802318913714,-44.4675934053985,-1.96882711702155));
#4972=CARTESIAN_POINT('Ctrl Pts',(17.6924798851479,-44.8234279063853,-1.4918948215464));
#4973=CARTESIAN_POINT('Ctrl Pts',(2.69247988514806,-19.542807947216,-2.20589829750609));
#4974=CARTESIAN_POINT('Ctrl Pts',(2.3635946338423,-19.9801257652426,-1.64906456309142));
#4975=CARTESIAN_POINT('Ctrl Pts',(2.28712243231041,-20.2717128410352,-0.928922098091803));
#4976=CARTESIAN_POINT('Ctrl Pts',(2.21065023077853,-20.5632999168279,-0.208779633092189));
#4977=CARTESIAN_POINT('Ctrl Pts',(2.42295829328197,-20.6881596294431,0.532038515331462));
#4978=CARTESIAN_POINT('Ctrl Pts',(2.63526635578541,-20.8130193420583,1.27285666375511));
#4979=CARTESIAN_POINT('Ctrl Pts',(3.1155254236359,-20.7831774696068,1.88762237576914));
#4980=CARTESIAN_POINT('Ctrl Pts',(3.5957844914864,-20.7533355971552,2.50238808778318));
#4981=CARTESIAN_POINT('Ctrl Pts',(4.27009432318328,-20.6114584639605,2.86933947451654));
#4982=CARTESIAN_POINT('Ctrl Pts',(4.94440415488017,-20.4695813307658,3.2362908612499));
#4983=CARTESIAN_POINT('Ctrl Pts',(5.70043037526654,-20.280525218564,3.28274870019663));
#4984=CARTESIAN_POINT('Ctrl Pts',(6.45645659565292,-20.0914691063622,3.32920653914337));
#4985=CARTESIAN_POINT('Ctrl Pts',(7.1656798966062,-19.929434672294,3.04596928553206));
#4986=CARTESIAN_POINT('Ctrl Pts',(7.87490319755949,-19.7674002382258,2.76273203192075));
#4987=CARTESIAN_POINT('Ctrl Pts',(8.41807416315096,-19.7012361646782,2.20589829750609));
#4988=CARTESIAN_POINT('Ctrl Pts',(8.96124512874244,-19.6350720911307,1.64906456309142));
#4989=CARTESIAN_POINT('Ctrl Pts',(9.25200304456004,-19.7146387598171,0.928922098091803));
#4990=CARTESIAN_POINT('Ctrl Pts',(9.54276096037763,-19.7942054285035,0.20877963309219));
#4991=CARTESIAN_POINT('Ctrl Pts',(9.5447386121599,-20.0404994603673,-0.532038515331461));
#4992=CARTESIAN_POINT('Ctrl Pts',(9.54671626394218,-20.2867934922312,-1.27285666375511));
#4993=CARTESIAN_POINT('Ctrl Pts',(9.28074291037739,-20.6877891091618,-1.88762237576914));
#4994=CARTESIAN_POINT('Ctrl Pts',(9.01476955681261,-21.0887847260924,-2.50238808778318));
#4995=CARTESIAN_POINT('Ctrl Pts',(8.55474543940143,-21.6018156037661,-2.86933947451654));
#4996=CARTESIAN_POINT('Ctrl Pts',(8.09472132199027,-22.1148464814399,-3.2362908612499));
#4997=CARTESIAN_POINT('Ctrl Pts',(7.5529808158896,-22.6750563381207,-3.28274870019663));
#4998=CARTESIAN_POINT('Ctrl Pts',(7.01124030978894,-23.2352661948015,-3.32920653914337));
#4999=CARTESIAN_POINT('Ctrl Pts',(6.51630272312137,-23.7684543733488,-3.04596928553206));
#5000=CARTESIAN_POINT('Ctrl Pts',(6.02136513645379,-24.3016425518961,-2.76273203192075));
#5001=CARTESIAN_POINT('Ctrl Pts',(5.69247988514803,-24.7389603699227,-2.20589829750609));
#5002=CARTESIAN_POINT('Ctrl Pts',(5.36359463384226,-25.1762781879492,-1.64906456309142));
#5003=CARTESIAN_POINT('Ctrl Pts',(5.28712243231038,-25.4678652637419,-0.928922098091803));
#5004=CARTESIAN_POINT('Ctrl Pts',(5.2106502307785,-25.7594523395345,-0.208779633092189));
#5005=CARTESIAN_POINT('Ctrl Pts',(5.42295829328193,-25.8843120521498,0.532038515331462));
#5006=CARTESIAN_POINT('Ctrl Pts',(5.63526635578538,-26.009171764765,1.27285666375511));
#5007=CARTESIAN_POINT('Ctrl Pts',(6.11552542363587,-25.9793298923134,1.88762237576914));
#5008=CARTESIAN_POINT('Ctrl Pts',(6.59578449148637,-25.9494880198619,2.50238808778318));
#5009=CARTESIAN_POINT('Ctrl Pts',(7.27009432318325,-25.8076108866672,2.86933947451654));
#5010=CARTESIAN_POINT('Ctrl Pts',(7.94440415488013,-25.6657337534725,3.2362908612499));
#5011=CARTESIAN_POINT('Ctrl Pts',(8.70043037526651,-25.4766776412707,3.28274870019663));
#5012=CARTESIAN_POINT('Ctrl Pts',(9.45645659565288,-25.2876215290689,3.32920653914337));
#5013=CARTESIAN_POINT('Ctrl Pts',(10.1656798966062,-25.1255870950007,3.04596928553206));
#5014=CARTESIAN_POINT('Ctrl Pts',(10.8749031975595,-24.9635526609324,2.76273203192075));
#5015=CARTESIAN_POINT('Ctrl Pts',(11.4180741631509,-24.8973885873849,2.20589829750609));
#5016=CARTESIAN_POINT('Ctrl Pts',(11.9612451287424,-24.8312245138374,1.64906456309142));
#5017=CARTESIAN_POINT('Ctrl Pts',(12.25200304456,-24.9107911825238,0.928922098091803));
#5018=CARTESIAN_POINT('Ctrl Pts',(12.5427609603776,-24.9903578512102,0.20877963309219));
#5019=CARTESIAN_POINT('Ctrl Pts',(12.5447386121599,-25.236651883074,-0.532038515331461));
#5020=CARTESIAN_POINT('Ctrl Pts',(12.5467162639421,-25.4829459149378,-1.27285666375511));
#5021=CARTESIAN_POINT('Ctrl Pts',(12.2807429103774,-25.8839415318684,-1.88762237576914));
#5022=CARTESIAN_POINT('Ctrl Pts',(12.0147695568126,-26.284937148799,-2.50238808778318));
#5023=CARTESIAN_POINT('Ctrl Pts',(11.5547454394014,-26.7979680264728,-2.86933947451654));
#5024=CARTESIAN_POINT('Ctrl Pts',(11.0947213219902,-27.3109989041465,-3.2362908612499));
#5025=CARTESIAN_POINT('Ctrl Pts',(10.5529808158896,-27.8712087608274,-3.28274870019663));
#5026=CARTESIAN_POINT('Ctrl Pts',(10.0112403097889,-28.4314186175082,-3.32920653914337));
#5027=CARTESIAN_POINT('Ctrl Pts',(9.51630272312133,-28.9646067960555,-3.04596928553206));
#5028=CARTESIAN_POINT('Ctrl Pts',(9.02136513645376,-29.4977949746027,-2.76273203192075));
#5029=CARTESIAN_POINT('Ctrl Pts',(8.692479885148,-29.9351127926293,-2.20589829750609));
#5030=CARTESIAN_POINT('Ctrl Pts',(8.36359463384224,-30.3724306106559,-1.64906456309142));
#5031=CARTESIAN_POINT('Ctrl Pts',(8.28712243231035,-30.6640176864485,-0.928922098091803));
#5032=CARTESIAN_POINT('Ctrl Pts',(8.21065023077846,-30.9556047622412,-0.208779633092189));
#5033=CARTESIAN_POINT('Ctrl Pts',(8.4229582932819,-31.0804644748564,0.532038515331462));
#5034=CARTESIAN_POINT('Ctrl Pts',(8.63526635578534,-31.2053241874716,1.27285666375511));
#5035=CARTESIAN_POINT('Ctrl Pts',(9.11552542363584,-31.1754823150201,1.88762237576914));
#5036=CARTESIAN_POINT('Ctrl Pts',(9.59578449148634,-31.1456404425685,2.50238808778318));
#5037=CARTESIAN_POINT('Ctrl Pts',(10.2700943231832,-31.0037633093738,2.86933947451654));
#5038=CARTESIAN_POINT('Ctrl Pts',(10.9444041548801,-30.8618861761791,3.2362908612499));
#5039=CARTESIAN_POINT('Ctrl Pts',(11.7004303752665,-30.6728300639773,3.28274870019663));
#5040=CARTESIAN_POINT('Ctrl Pts',(12.4564565956529,-30.4837739517755,3.32920653914337));
#5041=CARTESIAN_POINT('Ctrl Pts',(13.1656798966061,-30.3217395177073,3.04596928553206));
#5042=CARTESIAN_POINT('Ctrl Pts',(13.8749031975594,-30.1597050836391,2.76273203192075));
#5043=CARTESIAN_POINT('Ctrl Pts',(14.4180741631509,-30.0935410100915,2.20589829750609));
#5044=CARTESIAN_POINT('Ctrl Pts',(14.9612451287424,-30.027376936544,1.64906456309142));
#5045=CARTESIAN_POINT('Ctrl Pts',(15.25200304456,-30.1069436052304,0.928922098091803));
#5046=CARTESIAN_POINT('Ctrl Pts',(15.5427609603776,-30.1865102739168,0.20877963309219));
#5047=CARTESIAN_POINT('Ctrl Pts',(15.5447386121598,-30.4328043057806,-0.532038515331461));
#5048=CARTESIAN_POINT('Ctrl Pts',(15.5467162639421,-30.6790983376445,-1.27285666375511));
#5049=CARTESIAN_POINT('Ctrl Pts',(15.2807429103773,-31.0800939545751,-1.88762237576914));
#5050=CARTESIAN_POINT('Ctrl Pts',(15.0147695568125,-31.4810895715057,-2.50238808778318));
#5051=CARTESIAN_POINT('Ctrl Pts',(14.5547454394014,-31.9941204491794,-2.86933947451654));
#5052=CARTESIAN_POINT('Ctrl Pts',(14.0947213219902,-32.5071513268532,-3.2362908612499));
#5053=CARTESIAN_POINT('Ctrl Pts',(13.5529808158895,-33.067361183534,-3.28274870019663));
#5054=CARTESIAN_POINT('Ctrl Pts',(13.0112403097889,-33.6275710402148,-3.32920653914337));
#5055=CARTESIAN_POINT('Ctrl Pts',(12.5163027231213,-34.1607592187621,-3.04596928553206));
#5056=CARTESIAN_POINT('Ctrl Pts',(12.0213651364537,-34.6939473973094,-2.76273203192075));
#5057=CARTESIAN_POINT('Ctrl Pts',(11.692479885148,-35.131265215336,-2.20589829750609));
#5058=CARTESIAN_POINT('Ctrl Pts',(11.3635946338422,-35.5685830333625,-1.64906456309142));
#5059=CARTESIAN_POINT('Ctrl Pts',(11.2871224323103,-35.8601701091552,-0.928922098091803));
#5060=CARTESIAN_POINT('Ctrl Pts',(11.2106502307784,-36.1517571849478,-0.208779633092189));
#5061=CARTESIAN_POINT('Ctrl Pts',(11.4229582932819,-36.2766168975631,0.532038515331462));
#5062=CARTESIAN_POINT('Ctrl Pts',(11.6352663557853,-36.4014766101783,1.27285666375511));
#5063=CARTESIAN_POINT('Ctrl Pts',(12.1155254236358,-36.3716347377267,1.88762237576914));
#5064=CARTESIAN_POINT('Ctrl Pts',(12.5957844914863,-36.3417928652752,2.50238808778318));
#5065=CARTESIAN_POINT('Ctrl Pts',(13.2700943231832,-36.1999157320805,2.86933947451654));
#5066=CARTESIAN_POINT('Ctrl Pts',(13.9444041548801,-36.0580385988858,3.2362908612499));
#5067=CARTESIAN_POINT('Ctrl Pts',(14.7004303752664,-35.868982486684,3.28274870019663));
#5068=CARTESIAN_POINT('Ctrl Pts',(15.4564565956528,-35.6799263744822,3.32920653914337));
#5069=CARTESIAN_POINT('Ctrl Pts',(16.1656798966061,-35.517891940414,3.04596928553206));
#5070=CARTESIAN_POINT('Ctrl Pts',(16.8749031975594,-35.3558575063457,2.76273203192075));
#5071=CARTESIAN_POINT('Ctrl Pts',(17.4180741631509,-35.2896934327982,2.20589829750609));
#5072=CARTESIAN_POINT('Ctrl Pts',(17.9612451287423,-35.2235293592507,1.64906456309142));
#5073=CARTESIAN_POINT('Ctrl Pts',(18.2520030445599,-35.3030960279371,0.928922098091803));
#5074=CARTESIAN_POINT('Ctrl Pts',(18.5427609603775,-35.3826626966235,0.20877963309219));
#5075=CARTESIAN_POINT('Ctrl Pts',(18.5447386121598,-35.6289567284873,-0.532038515331461));
#5076=CARTESIAN_POINT('Ctrl Pts',(18.5467162639421,-35.8752507603511,-1.27285666375511));
#5077=CARTESIAN_POINT('Ctrl Pts',(18.2807429103773,-36.2762463772817,-1.88762237576914));
#5078=CARTESIAN_POINT('Ctrl Pts',(18.0147695568125,-36.6772419942123,-2.50238808778318));
#5079=CARTESIAN_POINT('Ctrl Pts',(17.5547454394013,-37.1902728718861,-2.86933947451654));
#5080=CARTESIAN_POINT('Ctrl Pts',(17.0947213219902,-37.7033037495598,-3.2362908612499));
#5081=CARTESIAN_POINT('Ctrl Pts',(16.5529808158895,-38.2635136062407,-3.28274870019663));
#5082=CARTESIAN_POINT('Ctrl Pts',(16.0112403097889,-38.8237234629215,-3.32920653914337));
#5083=CARTESIAN_POINT('Ctrl Pts',(15.5163027231213,-39.3569116414688,-3.04596928553206));
#5084=CARTESIAN_POINT('Ctrl Pts',(15.0213651364537,-39.890099820016,-2.76273203192075));
#5085=CARTESIAN_POINT('Ctrl Pts',(14.6924798851479,-40.3274176380426,-2.20589829750609));
#5086=CARTESIAN_POINT('Ctrl Pts',(14.3635946338422,-40.7647354560692,-1.64906456309142));
#5087=CARTESIAN_POINT('Ctrl Pts',(14.2871224323103,-41.0563225318618,-0.928922098091803));
#5088=CARTESIAN_POINT('Ctrl Pts',(14.2106502307784,-41.3479096076545,-0.208779633092189));
#5089=CARTESIAN_POINT('Ctrl Pts',(14.4229582932818,-41.4727693202697,0.532038515331462));
#5090=CARTESIAN_POINT('Ctrl Pts',(14.6352663557853,-41.5976290328849,1.27285666375511));
#5091=CARTESIAN_POINT('Ctrl Pts',(15.1155254236358,-41.5677871604334,1.88762237576914));
#5092=CARTESIAN_POINT('Ctrl Pts',(15.5957844914863,-41.5379452879818,2.50238808778318));
#5093=CARTESIAN_POINT('Ctrl Pts',(16.2700943231832,-41.3960681547871,2.86933947451654));
#5094=CARTESIAN_POINT('Ctrl Pts',(16.94440415488,-41.2541910215924,3.2362908612499));
#5095=CARTESIAN_POINT('Ctrl Pts',(17.7004303752664,-41.0651349093906,3.28274870019663));
#5096=CARTESIAN_POINT('Ctrl Pts',(18.4564565956528,-40.8760787971888,3.32920653914337));
#5097=CARTESIAN_POINT('Ctrl Pts',(19.1656798966061,-40.7140443631206,3.04596928553206));
#5098=CARTESIAN_POINT('Ctrl Pts',(19.8749031975594,-40.5520099290524,2.76273203192075));
#5099=CARTESIAN_POINT('Ctrl Pts',(20.4180741631508,-40.4858458555049,2.20589829750609));
#5100=CARTESIAN_POINT('Ctrl Pts',(20.9612451287423,-40.4196817819573,1.64906456309142));
#5101=CARTESIAN_POINT('Ctrl Pts',(21.2520030445599,-40.4992484506437,0.928922098091803));
#5102=CARTESIAN_POINT('Ctrl Pts',(21.5427609603775,-40.5788151193301,0.20877963309219));
#5103=CARTESIAN_POINT('Ctrl Pts',(21.5447386121598,-40.8251091511939,-0.532038515331461));
#5104=CARTESIAN_POINT('Ctrl Pts',(21.546716263942,-41.0714031830578,-1.27285666375511));
#5105=CARTESIAN_POINT('Ctrl Pts',(21.2807429103773,-41.4723987999884,-1.88762237576914));
#5106=CARTESIAN_POINT('Ctrl Pts',(21.0147695568125,-41.873394416919,-2.50238808778318));
#5107=CARTESIAN_POINT('Ctrl Pts',(20.5547454394013,-42.3864252945927,-2.86933947451654));
#5108=CARTESIAN_POINT('Ctrl Pts',(20.0947213219901,-42.8994561722665,-3.2362908612499));
#5109=CARTESIAN_POINT('Ctrl Pts',(19.5529808158895,-43.4596660289473,-3.28274870019663));
#5110=CARTESIAN_POINT('Ctrl Pts',(19.0112403097888,-44.0198758856281,-3.32920653914337));
#5111=CARTESIAN_POINT('Ctrl Pts',(18.5163027231212,-44.5530640641754,-3.04596928553206));
#5112=CARTESIAN_POINT('Ctrl Pts',(18.0213651364537,-45.0862522427227,-2.76273203192075));
#5113=CARTESIAN_POINT('Ctrl Pts',(17.6924798851479,-45.5235700607493,-2.20589829750609));
#5114=CARTESIAN_POINT('Ctrl Pts',(3.62216201968442,-19.8058202438613,-1.94799199564959));
#5115=CARTESIAN_POINT('Ctrl Pts',(3.34425572651223,-20.2137053466864,-1.54490813204841));
#5116=CARTESIAN_POINT('Ctrl Pts',(3.25594179788809,-20.5121292468035,-0.988830267143717));
#5117=CARTESIAN_POINT('Ctrl Pts',(3.16762786926396,-20.8105531469205,-0.432752402239027));
#5118=CARTESIAN_POINT('Ctrl Pts',(3.3076189187292,-20.9771651064803,0.166181422977342));
#5119=CARTESIAN_POINT('Ctrl Pts',(3.44760996819445,-21.1437770660401,0.765115248193711));
#5120=CARTESIAN_POINT('Ctrl Pts',(3.80940000840298,-21.1823333185883,1.28827884419634));
#5121=CARTESIAN_POINT('Ctrl Pts',(4.17119004861151,-21.2208895711365,1.81144244019896));
#5122=CARTESIAN_POINT('Ctrl Pts',(4.70434308191443,-21.1605093534924,2.15521684061908));
#5123=CARTESIAN_POINT('Ctrl Pts',(5.23749611521735,-21.1001291358485,2.49899124103919));
#5124=CARTESIAN_POINT('Ctrl Pts',(5.8576356015542,-20.9895272661294,2.59528770975726));
#5125=CARTESIAN_POINT('Ctrl Pts',(6.47777508789106,-20.8789253964104,2.69158417847533));
#5126=CARTESIAN_POINT('Ctrl Pts',(7.08329575335921,-20.7767637068552,2.52133001886304));
#5127=CARTESIAN_POINT('Ctrl Pts',(7.68881641882736,-20.6746020173,2.35107585925076));
#5128=CARTESIAN_POINT('Ctrl Pts',(8.18100842628526,-20.6378706589539,1.94799199564959));
#5129=CARTESIAN_POINT('Ctrl Pts',(8.67320043374317,-20.6011393006078,1.54490813204841));
#5130=CARTESIAN_POINT('Ctrl Pts',(8.97580007665302,-20.6738691449698,0.988830267143717));
#5131=CARTESIAN_POINT('Ctrl Pts',(9.27839971956287,-20.7465989893318,0.432752402239027));
#5132=CARTESIAN_POINT('Ctrl Pts',(9.35269438438334,-20.9511407742511,-0.166181422977342));
#5133=CARTESIAN_POINT('Ctrl Pts',(9.4269890492038,-21.1556825591703,-0.765115248193711));
#5134=CARTESIAN_POINT('Ctrl Pts',(9.27948472328098,-21.4882800511012,-1.28827884419634));
#5135=CARTESIAN_POINT('Ctrl Pts',(9.13198039735816,-21.8208775430321,-1.81144244019896));
#5136=CARTESIAN_POINT('Ctrl Pts',(8.81311307834095,-22.2524115051551,-2.15521684061908));
#5137=CARTESIAN_POINT('Ctrl Pts',(8.49424575932375,-22.6839454672782,-2.49899124103919));
#5138=CARTESIAN_POINT('Ctrl Pts',(8.0883919872726,-23.1657010814762,-2.59528770975726));
#5139=CARTESIAN_POINT('Ctrl Pts',(7.68253821522146,-23.6474566956743,-2.69158417847533));
#5140=CARTESIAN_POINT('Ctrl Pts',(7.29130326403902,-24.1207721297085,-2.52133001886305));
#5141=CARTESIAN_POINT('Ctrl Pts',(6.90006831285659,-24.5940875637428,-2.35107585925076));
#5142=CARTESIAN_POINT('Ctrl Pts',(6.62216201968439,-25.0019726665679,-1.94799199564959));
#5143=CARTESIAN_POINT('Ctrl Pts',(6.34425572651219,-25.4098577693931,-1.54490813204841));
#5144=CARTESIAN_POINT('Ctrl Pts',(6.25594179788806,-25.7082816695101,-0.988830267143717));
#5145=CARTESIAN_POINT('Ctrl Pts',(6.16762786926392,-26.0067055696272,-0.432752402239027));
#5146=CARTESIAN_POINT('Ctrl Pts',(6.30761891872917,-26.1733175291869,0.166181422977342));
#5147=CARTESIAN_POINT('Ctrl Pts',(6.44760996819441,-26.3399294887468,0.765115248193711));
#5148=CARTESIAN_POINT('Ctrl Pts',(6.80940000840295,-26.3784857412949,1.28827884419634));
#5149=CARTESIAN_POINT('Ctrl Pts',(7.17119004861148,-26.4170419938431,1.81144244019896));
#5150=CARTESIAN_POINT('Ctrl Pts',(7.7043430819144,-26.3566617761991,2.15521684061908));
#5151=CARTESIAN_POINT('Ctrl Pts',(8.23749611521731,-26.2962815585551,2.49899124103919));
#5152=CARTESIAN_POINT('Ctrl Pts',(8.85763560155417,-26.1856796888361,2.59528770975726));
#5153=CARTESIAN_POINT('Ctrl Pts',(9.47777508789103,-26.0750778191171,2.69158417847533));
#5154=CARTESIAN_POINT('Ctrl Pts',(10.0832957533592,-25.9729161295619,2.52133001886304));
#5155=CARTESIAN_POINT('Ctrl Pts',(10.6888164188273,-25.8707544400067,2.35107585925076));
#5156=CARTESIAN_POINT('Ctrl Pts',(11.1810084262852,-25.8340230816606,1.94799199564959));
#5157=CARTESIAN_POINT('Ctrl Pts',(11.6732004337431,-25.7972917233145,1.54490813204841));
#5158=CARTESIAN_POINT('Ctrl Pts',(11.975800076653,-25.8700215676765,0.988830267143717));
#5159=CARTESIAN_POINT('Ctrl Pts',(12.2783997195628,-25.9427514120385,0.432752402239027));
#5160=CARTESIAN_POINT('Ctrl Pts',(12.3526943843833,-26.1472931969577,-0.166181422977342));
#5161=CARTESIAN_POINT('Ctrl Pts',(12.4269890492038,-26.351834981877,-0.765115248193711));
#5162=CARTESIAN_POINT('Ctrl Pts',(12.279484723281,-26.6844324738078,-1.28827884419634));
#5163=CARTESIAN_POINT('Ctrl Pts',(12.1319803973581,-27.0170299657387,-1.81144244019896));
#5164=CARTESIAN_POINT('Ctrl Pts',(11.8131130783409,-27.4485639278618,-2.15521684061908));
#5165=CARTESIAN_POINT('Ctrl Pts',(11.4942457593237,-27.8800978899848,-2.49899124103919));
#5166=CARTESIAN_POINT('Ctrl Pts',(11.0883919872726,-28.3618535041829,-2.59528770975726));
#5167=CARTESIAN_POINT('Ctrl Pts',(10.6825382152214,-28.8436091183809,-2.69158417847533));
#5168=CARTESIAN_POINT('Ctrl Pts',(10.291303264039,-29.3169245524152,-2.52133001886305));
#5169=CARTESIAN_POINT('Ctrl Pts',(9.90006831285655,-29.7902399864494,-2.35107585925076));
#5170=CARTESIAN_POINT('Ctrl Pts',(9.62216201968436,-30.1981250892746,-1.94799199564959));
#5171=CARTESIAN_POINT('Ctrl Pts',(9.34425572651217,-30.6060101920997,-1.54490813204841));
#5172=CARTESIAN_POINT('Ctrl Pts',(9.25594179788803,-30.9044340922168,-0.988830267143717));
#5173=CARTESIAN_POINT('Ctrl Pts',(9.16762786926389,-31.2028579923338,-0.432752402239027));
#5174=CARTESIAN_POINT('Ctrl Pts',(9.30761891872914,-31.3694699518936,0.166181422977342));
#5175=CARTESIAN_POINT('Ctrl Pts',(9.44760996819438,-31.5360819114534,0.765115248193711));
#5176=CARTESIAN_POINT('Ctrl Pts',(9.80940000840292,-31.5746381640016,1.28827884419634));
#5177=CARTESIAN_POINT('Ctrl Pts',(10.1711900486115,-31.6131944165497,1.81144244019896));
#5178=CARTESIAN_POINT('Ctrl Pts',(10.7043430819144,-31.5528141989058,2.15521684061908));
#5179=CARTESIAN_POINT('Ctrl Pts',(11.2374961152173,-31.4924339812617,2.49899124103919));
#5180=CARTESIAN_POINT('Ctrl Pts',(11.8576356015541,-31.3818321115427,2.59528770975726));
#5181=CARTESIAN_POINT('Ctrl Pts',(12.477775087891,-31.2712302418237,2.69158417847533));
#5182=CARTESIAN_POINT('Ctrl Pts',(13.0832957533591,-31.1690685522685,2.52133001886304));
#5183=CARTESIAN_POINT('Ctrl Pts',(13.6888164188273,-31.0669068627133,2.35107585925076));
#5184=CARTESIAN_POINT('Ctrl Pts',(14.1810084262852,-31.0301755043672,1.94799199564959));
#5185=CARTESIAN_POINT('Ctrl Pts',(14.6732004337431,-30.9934441460211,1.54490813204841));
#5186=CARTESIAN_POINT('Ctrl Pts',(14.975800076653,-31.0661739903831,0.988830267143717));
#5187=CARTESIAN_POINT('Ctrl Pts',(15.2783997195628,-31.1389038347451,0.432752402239027));
#5188=CARTESIAN_POINT('Ctrl Pts',(15.3526943843833,-31.3434456196644,-0.166181422977342));
#5189=CARTESIAN_POINT('Ctrl Pts',(15.4269890492037,-31.5479874045836,-0.765115248193711));
#5190=CARTESIAN_POINT('Ctrl Pts',(15.2794847232809,-31.8805848965145,-1.28827884419634));
#5191=CARTESIAN_POINT('Ctrl Pts',(15.1319803973581,-32.2131823884454,-1.81144244019896));
#5192=CARTESIAN_POINT('Ctrl Pts',(14.8131130783409,-32.6447163505684,-2.15521684061908));
#5193=CARTESIAN_POINT('Ctrl Pts',(14.4942457593237,-33.0762503126915,-2.49899124103919));
#5194=CARTESIAN_POINT('Ctrl Pts',(14.0883919872725,-33.5580059268895,-2.59528770975726));
#5195=CARTESIAN_POINT('Ctrl Pts',(13.6825382152214,-34.0397615410876,-2.69158417847533));
#5196=CARTESIAN_POINT('Ctrl Pts',(13.291303264039,-34.5130769751218,-2.52133001886305));
#5197=CARTESIAN_POINT('Ctrl Pts',(12.9000683128565,-34.9863924091561,-2.35107585925076));
#5198=CARTESIAN_POINT('Ctrl Pts',(12.6221620196843,-35.3942775119812,-1.94799199564959));
#5199=CARTESIAN_POINT('Ctrl Pts',(12.3442557265121,-35.8021626148064,-1.54490813204841));
#5200=CARTESIAN_POINT('Ctrl Pts',(12.255941797888,-36.1005865149234,-0.988830267143717));
#5201=CARTESIAN_POINT('Ctrl Pts',(12.1676278692639,-36.3990104150405,-0.432752402239027));
#5202=CARTESIAN_POINT('Ctrl Pts',(12.3076189187291,-36.5656223746002,0.166181422977342));
#5203=CARTESIAN_POINT('Ctrl Pts',(12.4476099681944,-36.73223433416,0.765115248193711));
#5204=CARTESIAN_POINT('Ctrl Pts',(12.8094000084029,-36.7707905867082,1.28827884419634));
#5205=CARTESIAN_POINT('Ctrl Pts',(13.1711900486114,-36.8093468392564,1.81144244019896));
#5206=CARTESIAN_POINT('Ctrl Pts',(13.7043430819143,-36.7489666216124,2.15521684061908));
#5207=CARTESIAN_POINT('Ctrl Pts',(14.2374961152173,-36.6885864039684,2.49899124103919));
#5208=CARTESIAN_POINT('Ctrl Pts',(14.8576356015541,-36.5779845342494,2.59528770975726));
#5209=CARTESIAN_POINT('Ctrl Pts',(15.477775087891,-36.4673826645304,2.69158417847533));
#5210=CARTESIAN_POINT('Ctrl Pts',(16.0832957533591,-36.3652209749752,2.52133001886304));
#5211=CARTESIAN_POINT('Ctrl Pts',(16.6888164188273,-36.26305928542,2.35107585925076));
#5212=CARTESIAN_POINT('Ctrl Pts',(17.1810084262852,-36.2263279270739,1.94799199564959));
#5213=CARTESIAN_POINT('Ctrl Pts',(17.6732004337431,-36.1895965687278,1.54490813204841));
#5214=CARTESIAN_POINT('Ctrl Pts',(17.9758000766529,-36.2623264130898,0.988830267143717));
#5215=CARTESIAN_POINT('Ctrl Pts',(18.2783997195628,-36.3350562574518,0.432752402239027));
#5216=CARTESIAN_POINT('Ctrl Pts',(18.3526943843832,-36.539598042371,-0.166181422977342));
#5217=CARTESIAN_POINT('Ctrl Pts',(18.4269890492037,-36.7441398272903,-0.765115248193711));
#5218=CARTESIAN_POINT('Ctrl Pts',(18.2794847232809,-37.0767373192211,-1.28827884419634));
#5219=CARTESIAN_POINT('Ctrl Pts',(18.1319803973581,-37.409334811152,-1.81144244019896));
#5220=CARTESIAN_POINT('Ctrl Pts',(17.8131130783409,-37.8408687732751,-2.15521684061908));
#5221=CARTESIAN_POINT('Ctrl Pts',(17.4942457593237,-38.2724027353981,-2.49899124103919));
#5222=CARTESIAN_POINT('Ctrl Pts',(17.0883919872725,-38.7541583495962,-2.59528770975726));
#5223=CARTESIAN_POINT('Ctrl Pts',(16.6825382152214,-39.2359139637942,-2.69158417847533));
#5224=CARTESIAN_POINT('Ctrl Pts',(16.2913032640389,-39.7092293978285,-2.52133001886305));
#5225=CARTESIAN_POINT('Ctrl Pts',(15.9000683128565,-40.1825448318627,-2.35107585925076));
#5226=CARTESIAN_POINT('Ctrl Pts',(15.6221620196843,-40.5904299346879,-1.94799199564959));
#5227=CARTESIAN_POINT('Ctrl Pts',(15.3442557265121,-40.998315037513,-1.54490813204841));
#5228=CARTESIAN_POINT('Ctrl Pts',(15.255941797888,-41.2967389376301,-0.988830267143717));
#5229=CARTESIAN_POINT('Ctrl Pts',(15.1676278692638,-41.5951628377471,-0.432752402239027));
#5230=CARTESIAN_POINT('Ctrl Pts',(15.3076189187291,-41.7617747973069,0.166181422977342));
#5231=CARTESIAN_POINT('Ctrl Pts',(15.4476099681943,-41.9283867568667,0.765115248193711));
#5232=CARTESIAN_POINT('Ctrl Pts',(15.8094000084029,-41.9669430094149,1.28827884419634));
#5233=CARTESIAN_POINT('Ctrl Pts',(16.1711900486114,-42.0054992619631,1.81144244019896));
#5234=CARTESIAN_POINT('Ctrl Pts',(16.7043430819143,-41.945119044319,2.15521684061908));
#5235=CARTESIAN_POINT('Ctrl Pts',(17.2374961152172,-41.884738826675,2.49899124103919));
#5236=CARTESIAN_POINT('Ctrl Pts',(17.8576356015541,-41.774136956956,2.59528770975726));
#5237=CARTESIAN_POINT('Ctrl Pts',(18.4777750878909,-41.6635350872371,2.69158417847533));
#5238=CARTESIAN_POINT('Ctrl Pts',(19.0832957533591,-41.5613733976818,2.52133001886304));
#5239=CARTESIAN_POINT('Ctrl Pts',(19.6888164188272,-41.4592117081266,2.35107585925076));
#5240=CARTESIAN_POINT('Ctrl Pts',(20.1810084262851,-41.4224803497805,1.94799199564959));
#5241=CARTESIAN_POINT('Ctrl Pts',(20.673200433743,-41.3857489914344,1.54490813204841));
#5242=CARTESIAN_POINT('Ctrl Pts',(20.9758000766529,-41.4584788357964,0.988830267143717));
#5243=CARTESIAN_POINT('Ctrl Pts',(21.2783997195627,-41.5312086801584,0.432752402239027));
#5244=CARTESIAN_POINT('Ctrl Pts',(21.3526943843832,-41.7357504650777,-0.166181422977342));
#5245=CARTESIAN_POINT('Ctrl Pts',(21.4269890492037,-41.940292249997,-0.765115248193711));
#5246=CARTESIAN_POINT('Ctrl Pts',(21.2794847232809,-42.2728897419278,-1.28827884419634));
#5247=CARTESIAN_POINT('Ctrl Pts',(21.131980397358,-42.6054872338587,-1.81144244019896));
#5248=CARTESIAN_POINT('Ctrl Pts',(20.8131130783408,-43.0370211959817,-2.15521684061908));
#5249=CARTESIAN_POINT('Ctrl Pts',(20.4942457593236,-43.4685551581048,-2.49899124103919));
#5250=CARTESIAN_POINT('Ctrl Pts',(20.0883919872725,-43.9503107723028,-2.59528770975726));
#5251=CARTESIAN_POINT('Ctrl Pts',(19.6825382152213,-44.4320663865008,-2.69158417847533));
#5252=CARTESIAN_POINT('Ctrl Pts',(19.2913032640389,-44.9053818205351,-2.52133001886305));
#5253=CARTESIAN_POINT('Ctrl Pts',(18.9000683128565,-45.3786972545694,-2.35107585925076));
#5254=CARTESIAN_POINT('Ctrl Pts',(18.6221620196843,-45.7865823573945,-1.94799199564959));
#5255=CARTESIAN_POINT('',(4.2032568854171,-20.2749544279031,1.13384235805382));
#5256=CARTESIAN_POINT('',(3.23546955922298,-20.8337067011995,-0.275782109461829));
#5257=CARTESIAN_POINT('Ctrl Pts',(4.20325688541709,-20.2749544279031,1.13384235805383));
#5258=CARTESIAN_POINT('Ctrl Pts',(4.17353067602025,-20.2921168629003,1.00157233741796));
#5259=CARTESIAN_POINT('Ctrl Pts',(4.1267106773264,-20.3191484017499,0.826930627992248));
#5260=CARTESIAN_POINT('Ctrl Pts',(3.98429110156123,-20.4013743821558,0.245673499496276));
#5261=CARTESIAN_POINT('Ctrl Pts',(3.95326965129557,-20.4192846248171,0.063434900146937));
#5262=CARTESIAN_POINT('Ctrl Pts',(3.87127320952701,-20.4666252925448,-0.303997345944323));
#5263=CARTESIAN_POINT('Ctrl Pts',(3.83289404529189,-20.4887835133472,-0.445928116938839));
#5264=CARTESIAN_POINT('Ctrl Pts',(3.76001379967537,-20.5308609427725,-0.580444950877261));
#5265=CARTESIAN_POINT('Ctrl Pts',(3.73627207202441,-20.5445682356228,-0.614841199081482));
#5266=CARTESIAN_POINT('Ctrl Pts',(3.68747821159276,-20.5727393840778,-0.658095559969579));
#5267=CARTESIAN_POINT('Ctrl Pts',(3.66574669183764,-20.5852860829322,-0.67126084025885));
#5268=CARTESIAN_POINT('Ctrl Pts',(3.62032504182814,-20.6115102847922,-0.685243879141505));
#5269=CARTESIAN_POINT('Ctrl Pts',(3.59837730297536,-20.6241818176628,-0.686792486479322));
#5270=CARTESIAN_POINT('Ctrl Pts',(3.55016879873963,-20.6520150105605,-0.68047811375245));
#5271=CARTESIAN_POINT('Ctrl Pts',(3.52485041998139,-20.6666325833848,-0.670963714902961));
#5272=CARTESIAN_POINT('Ctrl Pts',(3.46539099876758,-20.7009614962285,-0.637810386100254));
#5273=CARTESIAN_POINT('Ctrl Pts',(3.43258170225768,-20.7199039523579,-0.609116109766831));
#5274=CARTESIAN_POINT('Ctrl Pts',(3.36695703423207,-20.757792372108,-0.536557857713739));
#5275=CARTESIAN_POINT('Ctrl Pts',(3.33473510032454,-20.7763957143233,-0.488582718568797));
#5276=CARTESIAN_POINT('Ctrl Pts',(3.29324460446342,-20.8003502632775,-0.412780370862962));
#5277=CARTESIAN_POINT('Ctrl Pts',(3.28021410458973,-20.8078734258878,-0.38607598492762));
#5278=CARTESIAN_POINT('Ctrl Pts',(3.25633438200707,-20.8216603901491,-0.331726097207036));
#5279=CARTESIAN_POINT('Ctrl Pts',(3.24541906679483,-20.8279623503246,-0.303953413725008));
#5280=CARTESIAN_POINT('Ctrl Pts',(3.23546955922298,-20.8337067011995,-0.275782109461826));
#5281=CARTESIAN_POINT('',(18.798465077288,-44.7175311486928,-1.53746850370033));
#5282=CARTESIAN_POINT('Ctrl Pts',(4.2032568854171,-20.2749544279031,1.13384235805382));
#5283=CARTESIAN_POINT('Ctrl Pts',(4.24461700886028,-20.2820537271614,1.17645708943624));
#5284=CARTESIAN_POINT('Ctrl Pts',(4.28785838370013,-20.2884806648945,1.21788038932571));
#5285=CARTESIAN_POINT('Ctrl Pts',(4.33277900087509,-20.2941850472034,1.25785531692514));
#5286=CARTESIAN_POINT('Ctrl Pts',(4.37777282801695,-20.2998987263045,1.29789539418882));
#5287=CARTESIAN_POINT('Ctrl Pts',(4.42445090390001,-20.3048873562845,1.33648171343798));
#5288=CARTESIAN_POINT('Ctrl Pts',(4.4725682388037,-20.3091157007804,1.37338328451688));
#5289=CARTESIAN_POINT('Ctrl Pts',(4.5206565890512,-20.3133414982293,1.41026262702987));
#5290=CARTESIAN_POINT('Ctrl Pts',(4.57018182638758,-20.3168078525493,1.44545870665561));
#5291=CARTESIAN_POINT('Ctrl Pts',(4.62086588701489,-20.3194963391104,1.47877717452078));
#5292=CARTESIAN_POINT('Ctrl Pts',(4.67156701372341,-20.3221857309251,1.51210686121238));
#5293=CARTESIAN_POINT('Ctrl Pts',(4.72342700590654,-20.3240967190121,1.54355727141904));
#5294=CARTESIAN_POINT('Ctrl Pts',(4.77614434033978,-20.3252282718733,1.57297724251041));
#5295=CARTESIAN_POINT('Ctrl Pts',(4.82886167477302,-20.3263598247345,1.60239721360178));
#5296=CARTESIAN_POINT('Ctrl Pts',(4.88243556544018,-20.3267119951369,1.62978652591198));
#5297=CARTESIAN_POINT('Ctrl Pts',(4.93655280986403,-20.3263008501883,1.65504205590817));
#5298=CARTESIAN_POINT('Ctrl Pts',(4.99059318650869,-20.3258902892273,1.68026171311514));
#5299=CARTESIAN_POINT('Ctrl Pts',(5.04595605131711,-20.3251645199386,1.70359676647101));
#5300=CARTESIAN_POINT('Ctrl Pts',(5.10236312310759,-20.3241201576957,1.72487226661214));
#5301=CARTESIAN_POINT('Ctrl Pts',(5.15878989379679,-20.3230754307329,1.74615519674227));
#5302=CARTESIAN_POINT('Ctrl Pts',(5.21626093600896,-20.3217118741235,1.76537666733536));
#5303=CARTESIAN_POINT('Ctrl Pts',(5.27446758778795,-20.3200331541901,1.78240346403954));
#5304=CARTESIAN_POINT('Ctrl Pts',(5.33272590071357,-20.3183529443137,1.79944537282823));
#5305=CARTESIAN_POINT('Ctrl Pts',(5.3917203532243,-20.3163570229522,1.81428839412964));
#5306=CARTESIAN_POINT('Ctrl Pts',(5.4511221884305,-20.3140561535612,1.82684686809475));
#5307=CARTESIAN_POINT('Ctrl Pts',(5.51047877834456,-20.3117570367003,1.83939577649979));
#5308=CARTESIAN_POINT('Ctrl Pts',(5.57024130034645,-20.3091534753514,1.84966349840266));
#5309=CARTESIAN_POINT('Ctrl Pts',(5.6300746296415,-20.3062628967142,1.85761563656239));
#5310=CARTESIAN_POINT('Ctrl Pts',(5.68987388180331,-20.3033739643607,1.86556324570669));
#5311=CARTESIAN_POINT('Ctrl Pts',(5.74974304733144,-20.300198402808,1.87119797990082));
#5312=CARTESIAN_POINT('Ctrl Pts',(5.80935283862858,-20.2967595360185,1.87453687269572));
#5313=CARTESIAN_POINT('Ctrl Pts',(5.82254342932584,-20.2959985757249,1.8752757105155));
#5314=CARTESIAN_POINT('Ctrl Pts',(5.83572136684984,-20.2952247433012,1.87590232633985));
#5315=CARTESIAN_POINT('Ctrl Pts',(5.84888317848182,-20.2944383255823,1.87641723476232));
#5316=CARTESIAN_POINT('Ctrl Pts',(5.90836858545831,-20.2908840748935,1.87874438682333));
#5317=CARTESIAN_POINT('Ctrl Pts',(5.96835659021567,-20.2874879798102,1.87880825693467));
#5318=CARTESIAN_POINT('Ctrl Pts',(6.02852369732613,-20.2842727601632,1.87655505226089));
#5319=CARTESIAN_POINT('Ctrl Pts',(6.08871181644296,-20.2810564176731,1.87430106070614));
#5320=CARTESIAN_POINT('Ctrl Pts',(6.14907837120147,-20.2780211361157,1.86972820122922));
#5321=CARTESIAN_POINT('Ctrl Pts',(6.20928772635011,-20.2751861548528,1.86283322829492));
#5322=CARTESIAN_POINT('Ctrl Pts',(6.26955052013898,-20.2723486574104,1.8559321357472));
#5323=CARTESIAN_POINT('Ctrl Pts',(6.32965499818605,-20.2697118625066,1.84670481534537));
#5324=CARTESIAN_POINT('Ctrl Pts',(6.38926509597254,-20.2672907526587,1.83519995710464));
#5325=CARTESIAN_POINT('Ctrl Pts',(6.44882978983705,-20.264871486926,1.82370386190416));
#5326=CARTESIAN_POINT('Ctrl Pts',(6.50790004501559,-20.2626676060139,1.80993391118304));
#5327=CARTESIAN_POINT('Ctrl Pts',(6.56615344995033,-20.2606891971314,1.79398881938349));
#5328=CARTESIAN_POINT('Ctrl Pts',(6.624373677573,-20.2587119150207,1.7780528088606));
#5329=CARTESIAN_POINT('Ctrl Pts',(6.68177726190263,-20.2569598574367,1.75994451788707));
#5330=CARTESIAN_POINT('Ctrl Pts',(6.73806677323732,-20.2554379551772,1.73980808434991));
#5331=CARTESIAN_POINT('Ctrl Pts',(6.75052264480493,-20.255101185171,1.73535224836872));
#5332=CARTESIAN_POINT('Ctrl Pts',(6.76292408311165,-20.2547756647794,1.73079726584414));
#5333=CARTESIAN_POINT('Ctrl Pts',(6.77526807902992,-20.2544614131831,1.72614496752461));
#5334=CARTESIAN_POINT('Ctrl Pts',(6.8310573306498,-20.2530411387843,1.70511869343335));
#5335=CARTESIAN_POINT('Ctrl Pts',(6.88646819440133,-20.2522876572929,1.68189873004129));
#5336=CARTESIAN_POINT('Ctrl Pts',(6.94118196331999,-20.2522209239189,1.65656309537197));
#5337=CARTESIAN_POINT('Ctrl Pts',(6.99591483978929,-20.2521541672398,1.63121861280326));
#5338=CARTESIAN_POINT('Ctrl Pts',(7.04994933840857,-20.2527746999987,1.60375713415829));
#5339=CARTESIAN_POINT('Ctrl Pts',(7.10297435817382,-20.2540875967032,1.57430602553659));
#5340=CARTESIAN_POINT('Ctrl Pts',(7.1560464401433,-20.2554016586654,1.5448287776679));
#5341=CARTESIAN_POINT('Ctrl Pts',(7.20810648127216,-20.2574093215818,1.51335869953408));
#5342=CARTESIAN_POINT('Ctrl Pts',(7.25886231563989,-20.2601002231023,1.48006918735993));
#5343=CARTESIAN_POINT('Ctrl Pts',(7.30957949021628,-20.2627890750122,1.44680503119875));
#5344=CARTESIAN_POINT('Ctrl Pts',(7.35899377471803,-20.2661600713697,1.41172471547131));
#5345=CARTESIAN_POINT('Ctrl Pts',(7.40684422911068,-20.2701878087831,1.37504051469708));
#5346=CARTESIAN_POINT('Ctrl Pts',(7.45466743102822,-20.2742132522618,1.33837720683351));
#5347=CARTESIAN_POINT('Ctrl Pts',(7.50092805869645,-20.2788945837058,1.30011245980337));
#5348=CARTESIAN_POINT('Ctrl Pts',(7.54540514539138,-20.2841925879918,1.26048896755347));
#5349=CARTESIAN_POINT('Ctrl Pts',(7.55524713666923,-20.2853649424747,1.25172099073438));
#5350=CARTESIAN_POINT('Ctrl Pts',(7.5650019652858,-20.2865674429003,1.2428865800128));
#5351=CARTESIAN_POINT('Ctrl Pts',(7.57466753434566,-20.2877995817719,1.2339885196899));
#5352=CARTESIAN_POINT('Ctrl Pts',(7.61835151381923,-20.2933682895055,1.19377333090042));
#5353=CARTESIAN_POINT('Ctrl Pts',(7.66088951452129,-20.3000469589609,1.15186853252888));
#5354=CARTESIAN_POINT('Ctrl Pts',(7.70201667224603,-20.3078244592172,1.1084685010314));
#5355=CARTESIAN_POINT('Ctrl Pts',(7.74315819270392,-20.3156046755901,1.06505331305083));
#5356=CARTESIAN_POINT('Ctrl Pts',(7.78288720787508,-20.3244844830689,1.02014229787602));
#5357=CARTESIAN_POINT('Ctrl Pts',(7.8209637992374,-20.334427858936,0.97396820682318));
#5358=CARTESIAN_POINT('Ctrl Pts',(7.85907418536895,-20.3443800600178,0.92775313408853));
#5359=CARTESIAN_POINT('Ctrl Pts',(7.89552862651523,-20.3553976202851,0.880273333152214));
#5360=CARTESIAN_POINT('Ctrl Pts',(7.93012136692561,-20.3674202884528,0.83179256319971));
#5361=CARTESIAN_POINT('Ctrl Pts',(7.96468775867802,-20.379433799174,0.783348720163393));
#5362=CARTESIAN_POINT('Ctrl Pts',(7.99739485206479,-20.3924506968192,0.733906126191045));
#5363=CARTESIAN_POINT('Ctrl Pts',(8.0280797616722,-20.4063889661352,0.68374857230742));
#5364=CARTESIAN_POINT('Ctrl Pts',(8.05874719517115,-20.4203192971289,0.633619584871035));
#5365=CARTESIAN_POINT('Ctrl Pts',(8.0873944899417,-20.4351696910629,0.582777184219427));
#5366=CARTESIAN_POINT('Ctrl Pts',(8.11390660288973,-20.4508397777779,0.531514551846599));
#5367=CARTESIAN_POINT('Ctrl Pts',(8.11977326376511,-20.4543072903381,0.520171039532054));
#5368=CARTESIAN_POINT('Ctrl Pts',(8.1255355657252,-20.4578148771029,0.508806964005077));
#5369=CARTESIAN_POINT('Ctrl Pts',(8.13119259206894,-20.46136134919,0.49742551165457));
#5370=CARTESIAN_POINT('Ctrl Pts',(8.15675978021637,-20.4773897912725,0.445986519513652));
#5371=CARTESIAN_POINT('Ctrl Pts',(8.18067882422748,-20.4948181203855,0.393696645408831));
#5372=CARTESIAN_POINT('Ctrl Pts',(8.20277709273188,-20.5135819549554,0.340828125587841));
#5373=CARTESIAN_POINT('Ctrl Pts',(8.22488307855853,-20.5323523423717,0.287941142627803));
#5374=CARTESIAN_POINT('Ctrl Pts',(8.24516655941384,-20.5524590343221,0.234475768276538));
#5375=CARTESIAN_POINT('Ctrl Pts',(8.26349134892837,-20.5738061183028,0.180724039814232));
#5376=CARTESIAN_POINT('Ctrl Pts',(8.28183240255724,-20.5951721488266,0.126924604159598));
#5377=CARTESIAN_POINT('Ctrl Pts',(8.2982109611232,-20.6177805253058,0.0728390372979704));
#5378=CARTESIAN_POINT('Ctrl Pts',(8.31253307602321,-20.6415064445685,0.0187692206340316));
#5379=CARTESIAN_POINT('Ctrl Pts',(8.32684428203008,-20.6652142922321,-0.0352594120388522));
#5380=CARTESIAN_POINT('Ctrl Pts',(8.339102027964,-20.6900376261338,-0.0892715721457783));
#5381=CARTESIAN_POINT('Ctrl Pts',(8.34925864520913,-20.7158279105711,-0.142968160449627));
#5382=CARTESIAN_POINT('Ctrl Pts',(8.35940947791238,-20.7416035065568,-0.196634166704727));
#5383=CARTESIAN_POINT('Ctrl Pts',(8.36746160014214,-20.7683445289011,-0.249984259986978));
#5384=CARTESIAN_POINT('Ctrl Pts',(8.37341437361217,-20.7958845557979,-0.302732839445703));
#5385=CARTESIAN_POINT('Ctrl Pts',(8.37473161691483,-20.801978675819,-0.314405165524747));
#5386=CARTESIAN_POINT('Ctrl Pts',(8.37594624412355,-20.8081118638264,-0.326048111329758));
#5387=CARTESIAN_POINT('Ctrl Pts',(8.37705855294184,-20.8142822298008,-0.337658719487504));
#5388=CARTESIAN_POINT('Ctrl Pts',(8.38208568329347,-20.842169479781,-0.390133391728609));
#5389=CARTESIAN_POINT('Ctrl Pts',(8.38532738969146,-20.871535875331,-0.442451690707123));
#5390=CARTESIAN_POINT('Ctrl Pts',(8.38672339583334,-20.9022521666488,-0.494317440111339));
#5391=CARTESIAN_POINT('Ctrl Pts',(8.3881198894989,-20.9329791849392,-0.54620130245975));
#5392=CARTESIAN_POINT('Ctrl Pts',(8.3876692117264,-20.9650567489548,-0.597631562887862));
#5393=CARTESIAN_POINT('Ctrl Pts',(8.38535091254483,-20.9983221257512,-0.648314739716445));
#5394=CARTESIAN_POINT('Ctrl Pts',(8.38303055576349,-21.0316170271372,-0.69904290025303));
#5395=CARTESIAN_POINT('Ctrl Pts',(8.37883922391101,-21.0661014353867,-0.749021923207224));
#5396=CARTESIAN_POINT('Ctrl Pts',(8.37279802773292,-21.101584117782,-0.797971596269669));
#5397=CARTESIAN_POINT('Ctrl Pts',(8.36676143302354,-21.1370397736666,-0.846883985260829));
#5398=CARTESIAN_POINT('Ctrl Pts',(8.35887791922486,-21.1734916692967,-0.894767940777761));
#5399=CARTESIAN_POINT('Ctrl Pts',(8.34920937659625,-21.2107280151238,-0.941368295643095));
#5400=CARTESIAN_POINT('Ctrl Pts',(8.33954634053429,-21.2479431535748,-0.987942110007974));
#5401=CARTESIAN_POINT('Ctrl Pts',(8.3281005770854,-21.2859412854642,-1.03323325565063));
#5402=CARTESIAN_POINT('Ctrl Pts',(8.31497167467398,-21.3244981230677,-1.07702027911484));
#5403=CARTESIAN_POINT('Ctrl Pts',(8.31206648117728,-21.3330300681115,-1.08670957162552));
#5404=CARTESIAN_POINT('Ctrl Pts',(8.30907900829624,-21.3415893397368,-1.09632535949929));
#5405=CARTESIAN_POINT('Ctrl Pts',(8.30601056182147,-21.350173465905,-1.10586550012264));
#5406=CARTESIAN_POINT('Ctrl Pts',(8.2921425782613,-21.3889698149884,-1.14898260006691));
#5407=CARTESIAN_POINT('Ctrl Pts',(8.27674396642908,-21.4290982032865,-1.19096704316453));
#5408=CARTESIAN_POINT('Ctrl Pts',(8.25986467402369,-21.47036574314,-1.23155737439074));
#5409=CARTESIAN_POINT('Ctrl Pts',(8.24297948690575,-21.511647694752,-1.27216188087552));
#5410=CARTESIAN_POINT('Ctrl Pts',(8.22461268059718,-21.5540691404009,-1.31137063355186));
#5411=CARTESIAN_POINT('Ctrl Pts',(8.20484862275808,-21.5974068306545,-1.34894683398735));
#5412=CARTESIAN_POINT('Ctrl Pts',(8.18506702338624,-21.6407829851505,-1.38655638507153));
#5413=CARTESIAN_POINT('Ctrl Pts',(8.16388591234771,-21.6850764469865,-1.42252990566971));
#5414=CARTESIAN_POINT('Ctrl Pts',(8.1414219230224,-21.7300408334262,-1.45666435205228));
#5415=CARTESIAN_POINT('Ctrl Pts',(8.11897504410718,-21.7749709713145,-1.49077279885092));
#5416=CARTESIAN_POINT('Ctrl Pts',(8.09524758180244,-21.8205703748796,-1.52304454512955));
#5417=CARTESIAN_POINT('Ctrl Pts',(8.07038362784117,-21.8665797955301,-1.55331889475944));
#5418=CARTESIAN_POINT('Ctrl Pts',(8.04553383475438,-21.9125630122376,-1.58357600210897));
#5419=CARTESIAN_POINT('Ctrl Pts',(8.01954926787334,-21.9589551262024,-1.61183773325823));
#5420=CARTESIAN_POINT('Ctrl Pts',(7.99259571310654,-22.0054936305649,-1.63799064371839));
#5421=CARTESIAN_POINT('Ctrl Pts',(7.98663136897745,-22.0157917770496,-1.64377781944758));
#5422=CARTESIAN_POINT('Ctrl Pts',(7.98061964812713,-22.0260970990538,-1.64946192467182));
#5423=CARTESIAN_POINT('Ctrl Pts',(7.97456245845175,-22.0364067769132,-1.65504205590818));
#5424=CARTESIAN_POINT('Ctrl Pts',(7.94718671390738,-22.0830018354371,-1.68026171311512));
#5425=CARTESIAN_POINT('Ctrl Pts',(7.91887674686191,-22.1305845981431,-1.70359676647099));
#5426=CARTESIAN_POINT('Ctrl Pts',(7.88976876673361,-22.1789123741453,-1.72487226661212));
#5427=CARTESIAN_POINT('Ctrl Pts',(7.86065062129931,-22.227257027534,-1.74615519674214));
#5428=CARTESIAN_POINT('Ctrl Pts',(7.83073422553015,-22.2763466317668,-1.76537666733516));
#5429=CARTESIAN_POINT('Ctrl Pts',(7.80017708553268,-22.3259157109097,-1.78240346403927));
#5430=CARTESIAN_POINT('Ctrl Pts',(7.76959282463327,-22.3755287849466,-1.79944537282796));
#5431=CARTESIAN_POINT('Ctrl Pts',(7.7383670797749,-22.4256215188224,-1.81428839412937));
#5432=CARTESIAN_POINT('Ctrl Pts',(7.70667355082844,-22.4759145824468,-1.82684686809449));
#5433=CARTESIAN_POINT('Ctrl Pts',(7.67500416226361,-22.526169338764,-1.83939577649957));
#5434=CARTESIAN_POINT('Ctrl Pts',(7.64286815099418,-22.5766234203374,-1.84966349840248));
#5435=CARTESIAN_POINT('Ctrl Pts',(7.61044817181519,-22.6269953141814,-1.85761563656225));
#5436=CARTESIAN_POINT('Ctrl Pts',(7.57804665692642,-22.677338519504,-1.86556324570655));
#5437=CARTESIAN_POINT('Ctrl Pts',(7.54536195718654,-22.7275989569782,-1.87119797990071));
#5438=CARTESIAN_POINT('Ctrl Pts',(7.51257891553807,-22.7775031171609,-1.87453687269564));
#5439=CARTESIAN_POINT('Ctrl Pts',(7.50532460924368,-22.7885460236493,-1.87527571051545));
#5440=CARTESIAN_POINT('Ctrl Pts',(7.49806548194417,-22.7995715361032,-1.87590232633983));
#5441=CARTESIAN_POINT('Ctrl Pts',(7.49080351840538,-22.8105767904773,-1.87641723476232));
#5442=CARTESIAN_POINT('Ctrl Pts',(7.45798274352922,-22.8603155387289,-1.87874438682333));
#5443=CARTESIAN_POINT('Ctrl Pts',(7.42504763653484,-22.9105686272294,-1.87880825693467));
#5444=CARTESIAN_POINT('Ctrl Pts',(7.3921796210866,-22.9610672606356,-1.8765550522609));
#5445=CARTESIAN_POINT('Ctrl Pts',(7.35930012722452,-23.0115835295518,-1.87430106070616));
#5446=CARTESIAN_POINT('Ctrl Pts',(7.32648821890885,-23.0623448587329,-1.86972820122924));
#5447=CARTESIAN_POINT('Ctrl Pts',(7.29392837554156,-23.1130701992057,-1.86283322829495));
#5448=CARTESIAN_POINT('Ctrl Pts',(7.26133963377882,-23.1638405608087,-1.85593213574724));
#5449=CARTESIAN_POINT('Ctrl Pts',(7.22900386338403,-23.2145741682268,-1.8467048153454));
#5450=CARTESIAN_POINT('Ctrl Pts',(7.19710207185721,-23.264987472308,-1.83519995710469));
#5451=CARTESIAN_POINT('Ctrl Pts',(7.16522457934186,-23.3153623774971,-1.82370386190419));
#5452=CARTESIAN_POINT('Ctrl Pts',(7.13378083489573,-23.3654167786337,-1.80993391118305));
#5453=CARTESIAN_POINT('Ctrl Pts',(7.10294078007701,-23.414876502723,-1.79398881938346));
#5454=CARTESIAN_POINT('Ctrl Pts',(7.07211828972738,-23.4643080578029,-1.77805280886061));
#5455=CARTESIAN_POINT('Ctrl Pts',(7.041899171186,-23.5131449913085,-1.75994451788714));
#5456=CARTESIAN_POINT('Ctrl Pts',(7.01243640949997,-23.5611321869611,-1.73980808435003));
#5457=CARTESIAN_POINT('Ctrl Pts',(7.00591682233549,-23.5717509031619,-1.73535224836881));
#5458=CARTESIAN_POINT('Ctrl Pts',(6.99943419425352,-23.5823281035833,-1.73079726584419));
#5459=CARTESIAN_POINT('Ctrl Pts',(6.99299004642871,-23.5928611918346,-1.72614496752462));
#5460=CARTESIAN_POINT('Ctrl Pts',(6.96386542690896,-23.6404659637964,-1.70511869343326));
#5461=CARTESIAN_POINT('Ctrl Pts',(6.93550746092023,-23.6880764387054,-1.68189873004107));
#5462=CARTESIAN_POINT('Ctrl Pts',(6.90809278366361,-23.735426585839,-1.6565630953716));
#5463=CARTESIAN_POINT('Ctrl Pts',(6.88066853244884,-23.7827932689443,-1.63121861280275));
#5464=CARTESIAN_POINT('Ctrl Pts',(6.85418868027218,-23.829898783809,-1.60375713415761));
#5465=CARTESIAN_POINT('Ctrl Pts',(6.82881317228806,-23.8764762463144,-1.57430602553571));
#5466=CARTESIAN_POINT('Ctrl Pts',(6.80341514234476,-23.9230950485127,-1.54482877766699));
#5467=CARTESIAN_POINT('Ctrl Pts',(6.77912380886821,-23.9691841981106,-1.51335869953315));
#5468=CARTESIAN_POINT('Ctrl Pts',(6.7560762807602,-24.0144854908235,-1.48006918735899));
#5469=CARTESIAN_POINT('Ctrl Pts',(6.73304630753319,-24.0597522783696,-1.44680503119794));
#5470=CARTESIAN_POINT('Ctrl Pts',(6.71125853376405,-24.1042318022364,-1.41172471547066));
#5471=CARTESIAN_POINT('Ctrl Pts',(6.69082142948761,-24.1476853800295,-1.3750405146966));
#5472=CARTESIAN_POINT('Ctrl Pts',(6.67039596484308,-24.1911142095195,-1.33837720683323));
#5473=CARTESIAN_POINT('Ctrl Pts',(6.65131980296306,-24.233517753997,-1.30011245980331));
#5474=CARTESIAN_POINT('Ctrl Pts',(6.63366946591674,-24.2746850431039,-1.26048896755363));
#5475=CARTESIAN_POINT('Ctrl Pts',(6.62976375904222,-24.2837946348158,-1.25172099073449));
#5476=CARTESIAN_POINT('Ctrl Pts',(6.6259277406506,-24.2928438144202,-1.24288658001286));
#5477=CARTESIAN_POINT('Ctrl Pts',(6.62216201968439,-24.3018305122039,-1.2339885196899));
#5478=CARTESIAN_POINT('Ctrl Pts',(6.60514267231111,-24.3424463020333,-1.19377333090037));
#5479=CARTESIAN_POINT('Ctrl Pts',(6.58965756937198,-24.3826246259952,-1.15186853252877));
#5480=CARTESIAN_POINT('Ctrl Pts',(6.57582950330943,-24.4221305394985,-1.10846850103124));
#5481=CARTESIAN_POINT('Ctrl Pts',(6.56199660810645,-24.4616502495516,-1.06505331305081));
#5482=CARTESIAN_POINT('Ctrl Pts',(6.54982223937827,-24.5004964896965,-1.02014229787617));
#5483=CARTESIAN_POINT('Ctrl Pts',(6.53939515979743,-24.5384434730392,-0.973968206823508));
#5484=CARTESIAN_POINT('Ctrl Pts',(6.52895882569208,-24.5764241361179,-0.927753134089022));
#5485=CARTESIAN_POINT('Ctrl Pts',(6.52027309219813,-24.6135033883649,-0.880273333152876));
#5486=CARTESIAN_POINT('Ctrl Pts',(6.51338865804746,-24.6494729144305,-0.831792563200549));
#5487=CARTESIAN_POINT('Ctrl Pts',(6.50650946764445,-24.6854150431657,-0.783348720164519));
#5488=CARTESIAN_POINT('Ctrl Pts',(6.50142888499027,-24.720248665745,-0.733906126192465));
#5489=CARTESIAN_POINT('Ctrl Pts',(6.49815732549905,-24.7537917116357,-0.683748572309139));
#5490=CARTESIAN_POINT('Ctrl Pts',(6.49488762927314,-24.7873156536116,-0.633619584872594));
#5491=CARTESIAN_POINT('Ctrl Pts',(6.49342480029085,-24.8195501355998,-0.582777184220826));
#5492=CARTESIAN_POINT('Ctrl Pts',(6.4937394369915,-24.8503453422784,-0.531514551847826));
#5493=CARTESIAN_POINT('Ctrl Pts',(6.49380906051888,-24.8571597759122,-0.520171039532874));
#5494=CARTESIAN_POINT('Ctrl Pts',(6.49396556878318,-24.8639038691766,-0.508806964005485));
#5495=CARTESIAN_POINT('Ctrl Pts',(6.49420839053254,-24.8705762337439,-0.497425511654569));
#5496=CARTESIAN_POINT('Ctrl Pts',(6.49530583448538,-24.9007322892242,-0.445986519513661));
#5497=CARTESIAN_POINT('Ctrl Pts',(6.49843968823718,-24.9301609535285,-0.393696645408851));
#5498=CARTESIAN_POINT('Ctrl Pts',(6.50364051139493,-24.9586805327179,-0.34082812558787));
#5499=CARTESIAN_POINT('Ctrl Pts',(6.508843150823,-24.9872100717278,-0.287941142627552));
#5500=CARTESIAN_POINT('Ctrl Pts',(6.51611431641051,-25.014829427401,-0.234475768275999));
#5501=CARTESIAN_POINT('Ctrl Pts',(6.52543903867732,-25.0413727026301,-0.180724039813404));
#5502=CARTESIAN_POINT('Ctrl Pts',(6.5347720370746,-25.0679395362668,-0.126924604158596));
#5503=CARTESIAN_POINT('Ctrl Pts',(6.54616218616096,-25.093427972302,-0.0728390372967965));
#5504=CARTESIAN_POINT('Ctrl Pts',(6.55954837752067,-25.1176942472727,-0.0187692206326862));
#5505=CARTESIAN_POINT('Ctrl Pts',(6.57292437286312,-25.1419420390654,0.0352594120404618));
#5506=CARTESIAN_POINT('Ctrl Pts',(6.58829313766177,-25.1649692253883,0.0892715721476517));
#5507=CARTESIAN_POINT('Ctrl Pts',(6.60554987053284,-25.1866602561578,0.142968160451755));
#5508=CARTESIAN_POINT('Ctrl Pts',(6.62279677510259,-25.2083389331412,0.196634166706848));
#5509=CARTESIAN_POINT('Ctrl Pts',(6.64192911866103,-25.2286827867186,0.249984259989086));
#5510=CARTESIAN_POINT('Ctrl Pts',(6.66280309483961,-25.247608053215,0.302732839447797));
#5511=CARTESIAN_POINT('Ctrl Pts',(6.66742213594002,-25.2517958793884,0.314405165526138));
#5512=CARTESIAN_POINT('Ctrl Pts',(6.67212631895598,-25.2559143714107,0.326048111330451));
#5513=CARTESIAN_POINT('Ctrl Pts',(6.67691385823105,-25.2599628420912,0.337658719487501));
#5514=CARTESIAN_POINT('Ctrl Pts',(6.69855135997981,-25.2782600896739,0.39013339172883));
#5515=CARTESIAN_POINT('Ctrl Pts',(6.72236255134487,-25.2957506875413,0.442451690707569));
#5516=CARTESIAN_POINT('Ctrl Pts',(6.7482656368653,-25.312317809983,0.494317440112001));
#5517=CARTESIAN_POINT('Ctrl Pts',(6.77417776845468,-25.3288907181188,0.546201302460738));
#5518=CARTESIAN_POINT('Ctrl Pts',(6.80218309267025,-25.3445392017269,0.59763156288917));
#5519=CARTESIAN_POINT('Ctrl Pts',(6.8321509036334,-25.3591641841403,0.648314739718059));
#5520=CARTESIAN_POINT('Ctrl Pts',(6.86214531244092,-25.3738021469148,0.699042900254681));
#5521=CARTESIAN_POINT('Ctrl Pts',(6.89410535194574,-25.3874145511796,0.749021923208903));
#5522=CARTESIAN_POINT('Ctrl Pts',(6.92785485438357,-25.3999240630178,0.797971596271375));
#5523=CARTESIAN_POINT('Ctrl Pts',(6.96157865044198,-25.4124240465893,0.84688398526218));
#5524=CARTESIAN_POINT('Ctrl Pts',(6.9970886749729,-25.4238226711835,0.894767940778771));
#5525=CARTESIAN_POINT('Ctrl Pts',(7.03417056771735,-25.434067640563,0.941368295643777));
#5526=CARTESIAN_POINT('Ctrl Pts',(7.07123134105188,-25.4443067750811,0.987942110008198));
#5527=CARTESIAN_POINT('Ctrl Pts',(7.10986157028853,-25.4533935191132,1.03323325565042));
#5528=CARTESIAN_POINT('Ctrl Pts',(7.14981722234809,-25.4613019749028,1.07702027911423));
#5529=CARTESIAN_POINT('Ctrl Pts',(7.15865870024823,-25.4630519760537,1.08670957162511));
#5530=CARTESIAN_POINT('Ctrl Pts',(7.16756498335432,-25.4647443844583,1.09632535949909));
#5531=CARTESIAN_POINT('Ctrl Pts',(7.17653327792285,-25.4663790949451,1.10586550012264));
#5532=CARTESIAN_POINT('Ctrl Pts',(7.21706589358342,-25.4737672434245,1.14898260006703));
#5533=CARTESIAN_POINT('Ctrl Pts',(7.2595174031787,-25.4804958485438,1.19096704316477));
#5534=CARTESIAN_POINT('Ctrl Pts',(7.30369578724639,-25.4865117224496,1.23155737439109));
#5535=CARTESIAN_POINT('Ctrl Pts',(7.34788959961906,-25.4925296972638,1.2721618808758));
#5536=CARTESIAN_POINT('Ctrl Pts',(7.39381105237047,-25.4978342992387,1.31137063355205));
#5537=CARTESIAN_POINT('Ctrl Pts',(7.4412246219909,-25.5023869681949,1.34894683398747));
#5538=CARTESIAN_POINT('Ctrl Pts',(7.48868027338876,-25.5069436778594,1.38655638507158));
#5539=CARTESIAN_POINT('Ctrl Pts',(7.53763009207947,-25.5107470285377,1.42252990566968));
#5540=CARTESIAN_POINT('Ctrl Pts',(7.58780238766435,-25.5137748363314,1.45666435205219));
#5541=CARTESIAN_POINT('Ctrl Pts',(7.63793646792892,-25.5168003378994,1.49077279885092));
#5542=CARTESIAN_POINT('Ctrl Pts',(7.68929044096624,-25.5190514545587,1.52304454512963));
#5543=CARTESIAN_POINT('Ctrl Pts',(7.74156774504371,-25.5205233491149,1.5533188947596));
#5544=CARTESIAN_POINT('Ctrl Pts',(7.7938152754032,-25.5219944053767,1.58357600210892));
#5545=CARTESIAN_POINT('Ctrl Pts',(7.84698430807213,-25.5226871673338,1.61183773325798));
#5546=CARTESIAN_POINT('Ctrl Pts',(7.90076461248722,-25.5226139563647,1.63799064371799));
#5547=CARTESIAN_POINT('Ctrl Pts',(7.91266524101966,-25.5225977560744,1.64377781944732));
#5548=CARTESIAN_POINT('Ctrl Pts',(7.92459577209495,-25.5225441140996,1.64946192467169));
#5549=CARTESIAN_POINT('Ctrl Pts',(7.936552809864,-25.5224532728949,1.65504205590817));
#5550=CARTESIAN_POINT('Ctrl Pts',(7.99059318650879,-25.5220427119339,1.6802617131152));
#5551=CARTESIAN_POINT('Ctrl Pts',(8.04595605131735,-25.5213169426452,1.70359676647112));
#5552=CARTESIAN_POINT('Ctrl Pts',(8.10236312310797,-25.5202725804024,1.7248722666123));
#5553=CARTESIAN_POINT('Ctrl Pts',(8.15878989379704,-25.5192278534395,1.74615519674236));
#5554=CARTESIAN_POINT('Ctrl Pts',(8.21626093600908,-25.5178642968302,1.7653766673354));
#5555=CARTESIAN_POINT('Ctrl Pts',(8.27446758778794,-25.5161855768968,1.78240346403954));
#5556=CARTESIAN_POINT('Ctrl Pts',(8.33272590071357,-25.5145053670204,1.79944537282824));
#5557=CARTESIAN_POINT('Ctrl Pts',(8.39172035322431,-25.5125094456588,1.81428839412965));
#5558=CARTESIAN_POINT('Ctrl Pts',(8.45112218843054,-25.5102085762678,1.82684686809477));
#5559=CARTESIAN_POINT('Ctrl Pts',(8.51047877834426,-25.5079094594069,1.83939577649973));
#5560=CARTESIAN_POINT('Ctrl Pts',(8.57024130034582,-25.5053058980581,1.84966349840256));
#5561=CARTESIAN_POINT('Ctrl Pts',(8.63007462964054,-25.5024153194209,1.85761563656227));
#5562=CARTESIAN_POINT('Ctrl Pts',(8.68987388180219,-25.4995263870674,1.86556324570657));
#5563=CARTESIAN_POINT('Ctrl Pts',(8.74974304733016,-25.4963508255147,1.87119797990072));
#5564=CARTESIAN_POINT('Ctrl Pts',(8.80935283862714,-25.4929119587252,1.87453687269564));
#5565=CARTESIAN_POINT('Ctrl Pts',(8.82254342932487,-25.4921509984316,1.87527571051545));
#5566=CARTESIAN_POINT('Ctrl Pts',(8.83572136684934,-25.4913771660079,1.87590232633983));
#5567=CARTESIAN_POINT('Ctrl Pts',(8.84888317848179,-25.490590748289,1.87641723476232));
#5568=CARTESIAN_POINT('Ctrl Pts',(8.90836858545845,-25.4870364976001,1.87874438682334));
#5569=CARTESIAN_POINT('Ctrl Pts',(8.968356590216,-25.4836404025168,1.87880825693467));
#5570=CARTESIAN_POINT('Ctrl Pts',(9.02852369732664,-25.4804251828698,1.87655505226086));
#5571=CARTESIAN_POINT('Ctrl Pts',(9.08871181644355,-25.4772088403798,1.8743010607061));
#5572=CARTESIAN_POINT('Ctrl Pts',(9.14907837120213,-25.4741735588223,1.86972820122916));
#5573=CARTESIAN_POINT('Ctrl Pts',(9.20928772635084,-25.4713385775594,1.86283322829483));
#5574=CARTESIAN_POINT('Ctrl Pts',(9.26955052013971,-25.468501080117,1.85593213574709));
#5575=CARTESIAN_POINT('Ctrl Pts',(9.32965499818679,-25.4658642852132,1.84670481534523));
#5576=CARTESIAN_POINT('Ctrl Pts',(9.38926509597328,-25.4634431753654,1.83519995710449));
#5577=CARTESIAN_POINT('Ctrl Pts',(9.44882978983824,-25.4610239096326,1.82370386190391));
#5578=CARTESIAN_POINT('Ctrl Pts',(9.5079000450172,-25.4588200287205,1.80993391118265));
#5579=CARTESIAN_POINT('Ctrl Pts',(9.56615344995236,-25.456841619838,1.79398881938292));
#5580=CARTESIAN_POINT('Ctrl Pts',(9.62437367757489,-25.4548643377273,1.77805280886001));
#5581=CARTESIAN_POINT('Ctrl Pts',(9.68177726190438,-25.4531122801433,1.75994451788648));
#5582=CARTESIAN_POINT('Ctrl Pts',(9.73806677323893,-25.4515903778838,1.73980808434933));
#5583=CARTESIAN_POINT('Ctrl Pts',(9.75052264480599,-25.4512536078776,1.73535224836833));
#5584=CARTESIAN_POINT('Ctrl Pts',(9.76292408311216,-25.4509280874861,1.73079726584394));
#5585=CARTESIAN_POINT('Ctrl Pts',(9.77526807902988,-25.4506138358897,1.72614496752462));
#5586=CARTESIAN_POINT('Ctrl Pts',(9.83105733064982,-25.449193561491,1.70511869343333));
#5587=CARTESIAN_POINT('Ctrl Pts',(9.8864681944014,-25.4484400799996,1.68189873004125));
#5588=CARTESIAN_POINT('Ctrl Pts',(9.94118196332011,-25.4483733466256,1.65656309537189));
#5589=CARTESIAN_POINT('Ctrl Pts',(9.99591483978936,-25.4483065899465,1.63121861280321));
#5590=CARTESIAN_POINT('Ctrl Pts',(10.0499493384086,-25.4489271227054,1.60375713415827));
#5591=CARTESIAN_POINT('Ctrl Pts',(10.1029743581738,-25.4502400194099,1.57430602553659));
#5592=CARTESIAN_POINT('Ctrl Pts',(10.1560464401432,-25.451554081372,1.54482877766791));
#5593=CARTESIAN_POINT('Ctrl Pts',(10.2081064812721,-25.4535617442885,1.51335869953411));
#5594=CARTESIAN_POINT('Ctrl Pts',(10.2588623156398,-25.4562526458089,1.48006918735998));
#5595=CARTESIAN_POINT('Ctrl Pts',(10.3095794902161,-25.4589414977189,1.44680503119883));
#5596=CARTESIAN_POINT('Ctrl Pts',(10.3589937747178,-25.4623124940763,1.41172471547144));
#5597=CARTESIAN_POINT('Ctrl Pts',(10.4068442291104,-25.4663402314897,1.37504051469726));
#5598=CARTESIAN_POINT('Ctrl Pts',(10.4546674310282,-25.4703656749685,1.33837720683351));
#5599=CARTESIAN_POINT('Ctrl Pts',(10.5009280586967,-25.4750470064124,1.30011245980319));
#5600=CARTESIAN_POINT('Ctrl Pts',(10.5454051453918,-25.4803450106985,1.26048896755308));
#5601=CARTESIAN_POINT('Ctrl Pts',(10.5552471366695,-25.4815173651814,1.25172099073412));
#5602=CARTESIAN_POINT('Ctrl Pts',(10.5650019652859,-25.482719865607,1.24288658001267));
#5603=CARTESIAN_POINT('Ctrl Pts',(10.5746675343456,-25.4839520044785,1.2339885196899));
#5604=CARTESIAN_POINT('Ctrl Pts',(10.6183515138194,-25.4895207122121,1.19377333090027));
#5605=CARTESIAN_POINT('Ctrl Pts',(10.6608895145216,-25.4961993816676,1.15186853252856));
#5606=CARTESIAN_POINT('Ctrl Pts',(10.7020166722465,-25.5039768819239,1.10846850103091));
#5607=CARTESIAN_POINT('Ctrl Pts',(10.7431581927042,-25.5117570982968,1.06505331305044));
#5608=CARTESIAN_POINT('Ctrl Pts',(10.7828872078753,-25.5206369057756,1.02014229787575));
#5609=CARTESIAN_POINT('Ctrl Pts',(10.8209637992375,-25.5305802816427,0.973968206823044));
#5610=CARTESIAN_POINT('Ctrl Pts',(10.859074185369,-25.5405324827245,0.927753134088394));
#5611=CARTESIAN_POINT('Ctrl Pts',(10.8955286265153,-25.5515500429918,0.880273333152076));
#5612=CARTESIAN_POINT('Ctrl Pts',(10.9301213669257,-25.5635727111595,0.831792563199574));
#5613=CARTESIAN_POINT('Ctrl Pts',(10.9646877586782,-25.5755862218807,0.783348720163117));
#5614=CARTESIAN_POINT('Ctrl Pts',(10.997394852065,-25.5886031195259,0.733906126190626));
#5615=CARTESIAN_POINT('Ctrl Pts',(11.0280797616725,-25.6025413888421,0.683748572306851));
#5616=CARTESIAN_POINT('Ctrl Pts',(11.0587471951712,-25.6164717198356,0.633619584870804));
#5617=CARTESIAN_POINT('Ctrl Pts',(11.0873944899416,-25.6313221137695,0.582777184219545));
#5618=CARTESIAN_POINT('Ctrl Pts',(11.1139066028895,-25.6469922004844,0.531514551847072));
#5619=CARTESIAN_POINT('Ctrl Pts',(11.1197732637649,-25.6504597130446,0.520171039532368));
#5620=CARTESIAN_POINT('Ctrl Pts',(11.1255355657251,-25.6539672998095,0.508806964005237));
#5621=CARTESIAN_POINT('Ctrl Pts',(11.1311925920689,-25.6575137718966,0.497425511654571));
#5622=CARTESIAN_POINT('Ctrl Pts',(11.1567597802163,-25.6735422139791,0.445986519513735));
#5623=CARTESIAN_POINT('Ctrl Pts',(11.1806788242274,-25.6909705430921,0.393696645409006));
#5624=CARTESIAN_POINT('Ctrl Pts',(11.2027770927317,-25.709734377662,0.340828125588102));
#5625=CARTESIAN_POINT('Ctrl Pts',(11.2248830785586,-25.7285047650784,0.287941142627488));
#5626=CARTESIAN_POINT('Ctrl Pts',(11.2451665594142,-25.7486114570291,0.234475768275634));
#5627=CARTESIAN_POINT('Ctrl Pts',(11.2634913489288,-25.76995854101,0.180724039812736));
#5628=CARTESIAN_POINT('Ctrl Pts',(11.2818324025577,-25.7913245715339,0.126924604158014));
#5629=CARTESIAN_POINT('Ctrl Pts',(11.2982109611237,-25.8139329480131,0.0728390372962978));
#5630=CARTESIAN_POINT('Ctrl Pts',(11.3125330760236,-25.8376588672759,0.0187692206322746));
#5631=CARTESIAN_POINT('Ctrl Pts',(11.3268442820305,-25.8613667149396,-0.0352594120405529));
#5632=CARTESIAN_POINT('Ctrl Pts',(11.3391020279643,-25.8861900488413,-0.0892715721474228));
#5633=CARTESIAN_POINT('Ctrl Pts',(11.3492586452094,-25.9119803332785,-0.142968160451209));
#5634=CARTESIAN_POINT('Ctrl Pts',(11.3594094779127,-25.9377559292644,-0.196634166706611));
#5635=CARTESIAN_POINT('Ctrl Pts',(11.3674616001424,-25.9644969516088,-0.249984259989154));
#5636=CARTESIAN_POINT('Ctrl Pts',(11.3734143736124,-25.9920369785058,-0.302732839448165));
#5637=CARTESIAN_POINT('Ctrl Pts',(11.374731616915,-25.9981310985265,-0.314405165526383));
#5638=CARTESIAN_POINT('Ctrl Pts',(11.3759462441236,-26.0042642865335,-0.326048111330576));
#5639=CARTESIAN_POINT('Ctrl Pts',(11.3770585529418,-26.0104346525075,-0.337658719487504));
#5640=CARTESIAN_POINT('Ctrl Pts',(11.3820856832934,-26.0383219024876,-0.390133391728687));
#5641=CARTESIAN_POINT('Ctrl Pts',(11.3853273896914,-26.0676882980378,-0.442451690707274));
#5642=CARTESIAN_POINT('Ctrl Pts',(11.3867233958333,-26.0984045893556,-0.494317440111565));
#5643=CARTESIAN_POINT('Ctrl Pts',(11.3881198894989,-26.1291316076458,-0.54620130245979));
#5644=CARTESIAN_POINT('Ctrl Pts',(11.3876692117264,-26.1612091716614,-0.597631562887722));
#5645=CARTESIAN_POINT('Ctrl Pts',(11.3853509125448,-26.1944745484577,-0.648314739716127));
#5646=CARTESIAN_POINT('Ctrl Pts',(11.3830305557635,-26.2277694498437,-0.699042900252813));
#5647=CARTESIAN_POINT('Ctrl Pts',(11.378839223911,-26.2622538580933,-0.749021923207109));
#5648=CARTESIAN_POINT('Ctrl Pts',(11.3727980277329,-26.2977365404886,-0.797971596269648));
#5649=CARTESIAN_POINT('Ctrl Pts',(11.3667614330235,-26.3331921963733,-0.846883985261025));
#5650=CARTESIAN_POINT('Ctrl Pts',(11.3588779192248,-26.3696440920036,-0.894767940778162));
#5651=CARTESIAN_POINT('Ctrl Pts',(11.3492093765961,-26.4068804378309,-0.941368295643691));
#5652=CARTESIAN_POINT('Ctrl Pts',(11.3395463405341,-26.4440955762819,-0.987942110008597));
#5653=CARTESIAN_POINT('Ctrl Pts',(11.3281005770852,-26.4820937081714,-1.03323325565127));
#5654=CARTESIAN_POINT('Ctrl Pts',(11.3149716746738,-26.5206505457749,-1.07702027911551));
#5655=CARTESIAN_POINT('Ctrl Pts',(11.3120664811771,-26.5291824908185,-1.08670957162596));
#5656=CARTESIAN_POINT('Ctrl Pts',(11.3090790082961,-26.5377417624436,-1.09632535949951));
#5657=CARTESIAN_POINT('Ctrl Pts',(11.3060105618214,-26.5463258886116,-1.10586550012264));
#5658=CARTESIAN_POINT('Ctrl Pts',(11.2921425782613,-26.5851222376949,-1.14898260006675));
#5659=CARTESIAN_POINT('Ctrl Pts',(11.2767439664292,-26.6252506259928,-1.19096704316423));
#5660=CARTESIAN_POINT('Ctrl Pts',(11.2598646740238,-26.6665181658462,-1.2315573743903));
#5661=CARTESIAN_POINT('Ctrl Pts',(11.2429794869062,-26.7078001174575,-1.27216188087439));
#5662=CARTESIAN_POINT('Ctrl Pts',(11.224612680598,-26.7502215631056,-1.31137063355007));
#5663=CARTESIAN_POINT('Ctrl Pts',(11.2048486227593,-26.7935592533584,-1.34894683398498));
#5664=CARTESIAN_POINT('Ctrl Pts',(11.1850670233875,-26.8369354078544,-1.38655638506922));
#5665=CARTESIAN_POINT('Ctrl Pts',(11.1638859123491,-26.8812288696903,-1.42252990566746));
#5666=CARTESIAN_POINT('Ctrl Pts',(11.1414219230238,-26.9261932561299,-1.4566643520501));
#5667=CARTESIAN_POINT('Ctrl Pts',(11.1189750441086,-26.9711233940183,-1.49077279884888));
#5668=CARTESIAN_POINT('Ctrl Pts',(11.0952475818039,-27.0167227975835,-1.52304454512765));
#5669=CARTESIAN_POINT('Ctrl Pts',(11.0703836278426,-27.062732218234,-1.55331889475767));
#5670=CARTESIAN_POINT('Ctrl Pts',(11.0455338347557,-27.1087154349417,-1.5835760021074));
#5671=CARTESIAN_POINT('Ctrl Pts',(11.0195492678746,-27.1551075489067,-1.61183773325684));
#5672=CARTESIAN_POINT('Ctrl Pts',(10.9925957131078,-27.2016460532694,-1.63799064371718));
#5673=CARTESIAN_POINT('Ctrl Pts',(10.9866313689783,-27.2119441997548,-1.64377781944678));
#5674=CARTESIAN_POINT('Ctrl Pts',(10.9806196481275,-27.2222495217598,-1.64946192467143));
#5675=CARTESIAN_POINT('Ctrl Pts',(10.9745624584517,-27.2325591996199,-1.65504205590817));
#5676=CARTESIAN_POINT('Ctrl Pts',(10.9471867139073,-27.2791542581438,-1.68026171311514));
#5677=CARTESIAN_POINT('Ctrl Pts',(10.9188767468618,-27.3267370208498,-1.70359676647102));
#5678=CARTESIAN_POINT('Ctrl Pts',(10.8897687667335,-27.375064796852,-1.72487226661215));
#5679=CARTESIAN_POINT('Ctrl Pts',(10.860650621299,-27.4234094502411,-1.74615519674231));
#5680=CARTESIAN_POINT('Ctrl Pts',(10.8307342255297,-27.4724990544741,-1.76537666733542));
#5681=CARTESIAN_POINT('Ctrl Pts',(10.800177085532,-27.5220681336174,-1.78240346403961));
#5682=CARTESIAN_POINT('Ctrl Pts',(10.7695928246326,-27.5716812076544,-1.7994453728283));
#5683=CARTESIAN_POINT('Ctrl Pts',(10.7383670797741,-27.6217739415302,-1.81428839412971));
#5684=CARTESIAN_POINT('Ctrl Pts',(10.7066735508276,-27.6720670051547,-1.82684686809482));
#5685=CARTESIAN_POINT('Ctrl Pts',(10.6750041622627,-27.722321761472,-1.83939577649987));
#5686=CARTESIAN_POINT('Ctrl Pts',(10.6428681509933,-27.7727758430455,-1.84966349840274));
#5687=CARTESIAN_POINT('Ctrl Pts',(10.6104481718142,-27.8231477368895,-1.85761563656247));
#5688=CARTESIAN_POINT('Ctrl Pts',(10.5780466569254,-27.8734909422121,-1.86556324570674));
#5689=CARTESIAN_POINT('Ctrl Pts',(10.5453619571855,-27.9237513796864,-1.87119797990086));
#5690=CARTESIAN_POINT('Ctrl Pts',(10.512578915537,-27.9736555398692,-1.87453687269574));
#5691=CARTESIAN_POINT('Ctrl Pts',(10.5053246092429,-27.9846984463571,-1.87527571051551));
#5692=CARTESIAN_POINT('Ctrl Pts',(10.4980654819438,-27.9957239588104,-1.87590232633986));
#5693=CARTESIAN_POINT('Ctrl Pts',(10.4908035184054,-28.0067292131839,-1.87641723476232));
#5694=CARTESIAN_POINT('Ctrl Pts',(10.4579827435293,-28.0564679614354,-1.87874438682332));
#5695=CARTESIAN_POINT('Ctrl Pts',(10.4250476365349,-28.1067210499358,-1.87880825693467));
#5696=CARTESIAN_POINT('Ctrl Pts',(10.3921796210867,-28.157219683342,-1.87655505226091));
#5697=CARTESIAN_POINT('Ctrl Pts',(10.359300127225,-28.2077359522577,-1.8743010607062));
#5698=CARTESIAN_POINT('Ctrl Pts',(10.3264882189097,-28.2584972814382,-1.86972820122937));
#5699=CARTESIAN_POINT('Ctrl Pts',(10.2939283755428,-28.3092226219104,-1.86283322829521));
#5700=CARTESIAN_POINT('Ctrl Pts',(10.26133963378,-28.3599929835134,-1.85593213574756));
#5701=CARTESIAN_POINT('Ctrl Pts',(10.2290038633852,-28.4107265909315,-1.84670481534578));
#5702=CARTESIAN_POINT('Ctrl Pts',(10.1971020718584,-28.4611398950128,-1.83519995710512));
#5703=CARTESIAN_POINT('Ctrl Pts',(10.165224579343,-28.5115148002019,-1.82370386190467));
#5704=CARTESIAN_POINT('Ctrl Pts',(10.1337808348968,-28.5615692013386,-1.80993391118357));
#5705=CARTESIAN_POINT('Ctrl Pts',(10.102940780078,-28.611028925428,-1.79398881938401));
#5706=CARTESIAN_POINT('Ctrl Pts',(10.0721182897286,-28.6604604805075,-1.77805280886132));
#5707=CARTESIAN_POINT('Ctrl Pts',(10.0418991711874,-28.7092974140128,-1.75994451788804));
#5708=CARTESIAN_POINT('Ctrl Pts',(10.0124364095016,-28.7572846096651,-1.73980808435114));
#5709=CARTESIAN_POINT('Ctrl Pts',(10.0059168223365,-28.7679033258668,-1.73535224836956));
#5710=CARTESIAN_POINT('Ctrl Pts',(9.99943419425403,-28.7784805262891,-1.73079726584457));
#5711=CARTESIAN_POINT('Ctrl Pts',(9.99299004642868,-28.7890136145413,-1.72614496752462));
#5712=CARTESIAN_POINT('Ctrl Pts',(9.96386542690912,-28.8366183865028,-1.70511869343339));
#5713=CARTESIAN_POINT('Ctrl Pts',(9.93550746092056,-28.8842288614115,-1.68189873004137));
#5714=CARTESIAN_POINT('Ctrl Pts',(9.90809278366411,-28.9315790085447,-1.65656309537209));
#5715=CARTESIAN_POINT('Ctrl Pts',(9.88066853244946,-28.9789456916498,-1.63121861280338));
#5716=CARTESIAN_POINT('Ctrl Pts',(9.85418868027291,-29.0260512065143,-1.60375713415841));
#5717=CARTESIAN_POINT('Ctrl Pts',(9.82881317228889,-29.0726286690195,-1.57430602553671));
#5718=CARTESIAN_POINT('Ctrl Pts',(9.80341514234551,-29.1192474712179,-1.54482877766797));
#5719=CARTESIAN_POINT('Ctrl Pts',(9.77912380886889,-29.1653366208159,-1.5133586995341));
#5720=CARTESIAN_POINT('Ctrl Pts',(9.7560762807608,-29.2106379135289,-1.48006918735989));
#5721=CARTESIAN_POINT('Ctrl Pts',(9.73304630753345,-29.2559047010756,-1.44680503119842));
#5722=CARTESIAN_POINT('Ctrl Pts',(9.711258533764,-29.3003842249431,-1.41172471547066));
#5723=CARTESIAN_POINT('Ctrl Pts',(9.69082142948729,-29.3438378027368,-1.37504051469608));
#5724=CARTESIAN_POINT('Ctrl Pts',(9.67039596484249,-29.3872666322274,-1.33837720683217));
#5725=CARTESIAN_POINT('Ctrl Pts',(9.65131980296222,-29.4296701767054,-1.30011245980167));
#5726=CARTESIAN_POINT('Ctrl Pts',(9.63366946591571,-29.4708374658129,-1.26048896755137));
#5727=CARTESIAN_POINT('Ctrl Pts',(9.62976375904153,-29.479947057524,-1.25172099073297));
#5728=CARTESIAN_POINT('Ctrl Pts',(9.62592774065024,-29.4889962371276,-1.24288658001209));
#5729=CARTESIAN_POINT('Ctrl Pts',(9.62216201968436,-29.4979829349106,-1.2339885196899));
#5730=CARTESIAN_POINT('Ctrl Pts',(9.6051426723111,-29.5385987247399,-1.19377333090041));
#5731=CARTESIAN_POINT('Ctrl Pts',(9.58965756937199,-29.5787770487018,-1.15186853252886));
#5732=CARTESIAN_POINT('Ctrl Pts',(9.57582950330945,-29.618282962205,-1.10846850103139));
#5733=CARTESIAN_POINT('Ctrl Pts',(9.5619966081064,-29.6578026722583,-1.06505331305076));
#5734=CARTESIAN_POINT('Ctrl Pts',(9.54982223937817,-29.6966489124034,-1.0201422978759));
#5735=CARTESIAN_POINT('Ctrl Pts',(9.53939515979729,-29.7345958957462,-0.973968206823007));
#5736=CARTESIAN_POINT('Ctrl Pts',(9.52895882569192,-29.772576558825,-0.927753134088401));
#5737=CARTESIAN_POINT('Ctrl Pts',(9.52027309219798,-29.8096558110721,-0.880273333152132));
#5738=CARTESIAN_POINT('Ctrl Pts',(9.51338865804731,-29.8456253371378,-0.831792563199677));
#5739=CARTESIAN_POINT('Ctrl Pts',(9.50650946764427,-29.8815674658732,-0.783348720163336));
#5740=CARTESIAN_POINT('Ctrl Pts',(9.5014288849901,-29.9164010884527,-0.733906126190959));
#5741=CARTESIAN_POINT('Ctrl Pts',(9.4981573254989,-29.9499441343436,-0.683748572307306));
#5742=CARTESIAN_POINT('Ctrl Pts',(9.49488762927306,-29.9834680763192,-0.633619584871212));
#5743=CARTESIAN_POINT('Ctrl Pts',(9.49342480029081,-30.015702558307,-0.582777184219908));
#5744=CARTESIAN_POINT('Ctrl Pts',(9.49373943699148,-30.0464977649853,-0.531514551847384));
#5745=CARTESIAN_POINT('Ctrl Pts',(9.49380906051886,-30.053312198619,-0.520171039532578));
#5746=CARTESIAN_POINT('Ctrl Pts',(9.49396556878315,-30.0600562918833,-0.508806964005337));
#5747=CARTESIAN_POINT('Ctrl Pts',(9.49420839053251,-30.0667286564506,-0.497425511654568));
#5748=CARTESIAN_POINT('Ctrl Pts',(9.49530583448534,-30.0968847119308,-0.445986519513711));
#5749=CARTESIAN_POINT('Ctrl Pts',(9.49843968823714,-30.1263133762351,-0.393696645408955));
#5750=CARTESIAN_POINT('Ctrl Pts',(9.50364051139489,-30.1548329554245,-0.34082812558803));
#5751=CARTESIAN_POINT('Ctrl Pts',(9.50884315082298,-30.1833624944346,-0.287941142627382));
#5752=CARTESIAN_POINT('Ctrl Pts',(9.51611431641054,-30.2109818501079,-0.234475768275499));
#5753=CARTESIAN_POINT('Ctrl Pts',(9.52543903867744,-30.2375251253372,-0.180724039812564));
#5754=CARTESIAN_POINT('Ctrl Pts',(9.53477203707472,-30.2640919589739,-0.126924604157851));
#5755=CARTESIAN_POINT('Ctrl Pts',(9.54616218616107,-30.2895803950089,-0.0728390372961486));
#5756=CARTESIAN_POINT('Ctrl Pts',(9.55954837752077,-30.3138466699796,-0.0187692206321375));
#5757=CARTESIAN_POINT('Ctrl Pts',(9.57292437286319,-30.3380944617722,0.0352594120408156));
#5758=CARTESIAN_POINT('Ctrl Pts',(9.58829313766179,-30.361121648095,0.0892715721478093));
#5759=CARTESIAN_POINT('Ctrl Pts',(9.6055498705328,-30.3828126788644,0.142968160451718));
#5760=CARTESIAN_POINT('Ctrl Pts',(9.62279677510249,-30.4044913558477,0.196634166706646));
#5761=CARTESIAN_POINT('Ctrl Pts',(9.64192911866087,-30.4248352094251,0.249984259988728));
#5762=CARTESIAN_POINT('Ctrl Pts',(9.66280309483938,-30.4437604759214,0.30273283944728));
#5763=CARTESIAN_POINT('Ctrl Pts',(9.66742213593985,-30.4479483020949,0.314405165525795));
#5764=CARTESIAN_POINT('Ctrl Pts',(9.67212631895587,-30.4520667941173,0.326048111330278));
#5765=CARTESIAN_POINT('Ctrl Pts',(9.67691385823102,-30.4561152647978,0.3376587194875));
#5766=CARTESIAN_POINT('Ctrl Pts',(9.69855135997969,-30.4744125123805,0.390133391728636));
#5767=CARTESIAN_POINT('Ctrl Pts',(9.72236255134466,-30.4919031102478,0.442451690707181));
#5768=CARTESIAN_POINT('Ctrl Pts',(9.74826563686498,-30.5084702326894,0.494317440111426));
#5769=CARTESIAN_POINT('Ctrl Pts',(9.77417776845419,-30.5250431408252,0.546201302459856));
#5770=CARTESIAN_POINT('Ctrl Pts',(9.80218309266957,-30.5406916244332,0.597631562887992));
#5771=CARTESIAN_POINT('Ctrl Pts',(9.8321509036325,-30.5553166068466,0.648314739716593));
#5772=CARTESIAN_POINT('Ctrl Pts',(9.86214531244,-30.5699545696211,0.699042900253254));
#5773=CARTESIAN_POINT('Ctrl Pts',(9.8941053519448,-30.5835669738859,0.749021923207519));
#5774=CARTESIAN_POINT('Ctrl Pts',(9.92785485438261,-30.5960764857241,0.797971596270033));
#5775=CARTESIAN_POINT('Ctrl Pts',(9.96157865044122,-30.6085764692957,0.846883985261196));
#5776=CARTESIAN_POINT('Ctrl Pts',(9.99708867497237,-30.61997509389,0.894767940778138));
#5777=CARTESIAN_POINT('Ctrl Pts',(10.0341705677171,-30.6302200632696,0.941368295643474));
#5778=CARTESIAN_POINT('Ctrl Pts',(10.071231341052,-30.6404591977878,0.987942110008423));
#5779=CARTESIAN_POINT('Ctrl Pts',(10.1098615702891,-30.64954594182,1.03323325565114));
#5780=CARTESIAN_POINT('Ctrl Pts',(10.1498172223491,-30.6574543976097,1.07702027911541));
#5781=CARTESIAN_POINT('Ctrl Pts',(10.1586587002489,-30.6592043987605,1.0867095716259));
#5782=CARTESIAN_POINT('Ctrl Pts',(10.1675649833546,-30.660896807165,1.09632535949948));
#5783=CARTESIAN_POINT('Ctrl Pts',(10.1765332779228,-30.6625315176518,1.10586550012264));
#5784=CARTESIAN_POINT('Ctrl Pts',(10.2170658935834,-30.6699196661312,1.14898260006707));
#5785=CARTESIAN_POINT('Ctrl Pts',(10.2595174031787,-30.6766482712505,1.19096704316485));
#5786=CARTESIAN_POINT('Ctrl Pts',(10.3036957872465,-30.6826641451563,1.2315573743912));
#5787=CARTESIAN_POINT('Ctrl Pts',(10.347889599619,-30.6886821199705,1.27216188087579));
#5788=CARTESIAN_POINT('Ctrl Pts',(10.3938110523703,-30.6939867219453,1.31137063355195));
#5789=CARTESIAN_POINT('Ctrl Pts',(10.4412246219906,-30.6985393909015,1.34894683398728));
#5790=CARTESIAN_POINT('Ctrl Pts',(10.4886802733886,-30.7030961005661,1.38655638507146));
#5791=CARTESIAN_POINT('Ctrl Pts',(10.5376300920794,-30.7068994512443,1.42252990566964));
#5792=CARTESIAN_POINT('Ctrl Pts',(10.5878023876643,-30.7099272590381,1.45666435205221));
#5793=CARTESIAN_POINT('Ctrl Pts',(10.637936467929,-30.712952760606,1.49077279885102));
#5794=CARTESIAN_POINT('Ctrl Pts',(10.6892904409665,-30.7152038772653,1.5230445451298));
#5795=CARTESIAN_POINT('Ctrl Pts',(10.7415677450441,-30.7166757718216,1.55331889475982));
#5796=CARTESIAN_POINT('Ctrl Pts',(10.7938152754037,-30.7181468280834,1.58357600210919));
#5797=CARTESIAN_POINT('Ctrl Pts',(10.8469843080727,-30.7188395900405,1.61183773325829));
#5798=CARTESIAN_POINT('Ctrl Pts',(10.9007646124879,-30.7187663790714,1.63799064371833));
#5799=CARTESIAN_POINT('Ctrl Pts',(10.9126652410201,-30.718750178781,1.64377781944754));
#5800=CARTESIAN_POINT('Ctrl Pts',(10.9245957720951,-30.7186965368063,1.6494619246718));
#5801=CARTESIAN_POINT('Ctrl Pts',(10.936552809864,-30.7186056956016,1.65504205590817));
#5802=CARTESIAN_POINT('Ctrl Pts',(10.9905931865086,-30.7181951346406,1.68026171311514));
#5803=CARTESIAN_POINT('Ctrl Pts',(11.0459560513171,-30.7174693653519,1.70359676647102));
#5804=CARTESIAN_POINT('Ctrl Pts',(11.1023631231076,-30.716425003109,1.72487226661216));
#5805=CARTESIAN_POINT('Ctrl Pts',(11.1587898937964,-30.7153802761462,1.74615519674216));
#5806=CARTESIAN_POINT('Ctrl Pts',(11.2162609360083,-30.7140167195368,1.76537666733515));
#5807=CARTESIAN_POINT('Ctrl Pts',(11.2744675877869,-30.7123379996035,1.78240346403925));
#5808=CARTESIAN_POINT('Ctrl Pts',(11.3327259007125,-30.7106577897271,1.79944537282797));
#5809=CARTESIAN_POINT('Ctrl Pts',(11.3917203532232,-30.7086618683655,1.8142883941294));
#5810=CARTESIAN_POINT('Ctrl Pts',(11.4511221884294,-30.7063609989745,1.82684686809454));
#5811=CARTESIAN_POINT('Ctrl Pts',(11.5104787783434,-30.7040618821136,1.83939577649959));
#5812=CARTESIAN_POINT('Ctrl Pts',(11.5702413003453,-30.7014583207647,1.84966349840248));
#5813=CARTESIAN_POINT('Ctrl Pts',(11.6300746296403,-30.6985677421276,1.85761563656223));
#5814=CARTESIAN_POINT('Ctrl Pts',(11.6898738818019,-30.6956788097741,1.86556324570655));
#5815=CARTESIAN_POINT('Ctrl Pts',(11.7497430473299,-30.6925032482214,1.8711979799007));
#5816=CARTESIAN_POINT('Ctrl Pts',(11.809352838627,-30.6890643814319,1.87453687269563));
#5817=CARTESIAN_POINT('Ctrl Pts',(11.8225434293247,-30.6883034211383,1.87527571051545));
#5818=CARTESIAN_POINT('Ctrl Pts',(11.8357213668493,-30.6875295887145,1.87590232633983));
#5819=CARTESIAN_POINT('Ctrl Pts',(11.8488831784818,-30.6867431709956,1.87641723476232));
#5820=CARTESIAN_POINT('Ctrl Pts',(11.9083685854582,-30.6831889203068,1.87874438682333));
#5821=CARTESIAN_POINT('Ctrl Pts',(11.9683565902155,-30.6797928252235,1.87880825693467));
#5822=CARTESIAN_POINT('Ctrl Pts',(12.0285236973258,-30.6765776055765,1.87655505226089));
#5823=CARTESIAN_POINT('Ctrl Pts',(12.0887118164422,-30.6733612630865,1.87430106070617));
#5824=CARTESIAN_POINT('Ctrl Pts',(12.1490783712002,-30.6703259815291,1.86972820122931));
#5825=CARTESIAN_POINT('Ctrl Pts',(12.2092877263483,-30.6674910002661,1.86283322829512));
#5826=CARTESIAN_POINT('Ctrl Pts',(12.2695505201372,-30.6646535028237,1.85593213574744));
#5827=CARTESIAN_POINT('Ctrl Pts',(12.3296549981843,-30.6620167079199,1.84670481534564));
#5828=CARTESIAN_POINT('Ctrl Pts',(12.3892650959708,-30.6595955980721,1.83519995710496));
#5829=CARTESIAN_POINT('Ctrl Pts',(12.4488297898355,-30.6571763323394,1.82370386190449));
#5830=CARTESIAN_POINT('Ctrl Pts',(12.5079000450142,-30.6549724514273,1.80993391118336));
#5831=CARTESIAN_POINT('Ctrl Pts',(12.5661534499491,-30.6529940425448,1.7939888193838));
#5832=CARTESIAN_POINT('Ctrl Pts',(12.6243736775717,-30.651016760434,1.77805280886096));
#5833=CARTESIAN_POINT('Ctrl Pts',(12.6817772619013,-30.64926470285,1.75994451788749));
#5834=CARTESIAN_POINT('Ctrl Pts',(12.7380667732359,-30.6477428005906,1.73980808435039));
#5835=CARTESIAN_POINT('Ctrl Pts',(12.750522644804,-30.6474060305843,1.73535224836905));
#5836=CARTESIAN_POINT('Ctrl Pts',(12.7629240831111,-30.6470805101927,1.73079726584431));
#5837=CARTESIAN_POINT('Ctrl Pts',(12.7752680790299,-30.6467662585964,1.72614496752461));
#5838=CARTESIAN_POINT('Ctrl Pts',(12.8310573306496,-30.6453459841976,1.70511869343341));
#5839=CARTESIAN_POINT('Ctrl Pts',(12.8864681944009,-30.6445925027062,1.68189873004143));
#5840=CARTESIAN_POINT('Ctrl Pts',(12.9411819633194,-30.6445257693322,1.6565630953722));
#5841=CARTESIAN_POINT('Ctrl Pts',(12.9959148397886,-30.6444590126531,1.63121861280354));
#5842=CARTESIAN_POINT('Ctrl Pts',(13.0499493384079,-30.645079545412,1.60375713415863));
#5843=CARTESIAN_POINT('Ctrl Pts',(13.1029743581731,-30.6463924421165,1.57430602553699));
#5844=CARTESIAN_POINT('Ctrl Pts',(13.1560464401424,-30.6477065040787,1.54482877766837));
#5845=CARTESIAN_POINT('Ctrl Pts',(13.2081064812712,-30.6497141669951,1.51335869953463));
#5846=CARTESIAN_POINT('Ctrl Pts',(13.2588623156389,-30.6524050685155,1.48006918736057));
#5847=CARTESIAN_POINT('Ctrl Pts',(13.3095794902154,-30.6550939204255,1.44680503119932));
#5848=CARTESIAN_POINT('Ctrl Pts',(13.3589937747173,-30.6584649167829,1.41172471547181));
#5849=CARTESIAN_POINT('Ctrl Pts',(13.4068442291101,-30.6624926541963,1.3750405146975));
#5850=CARTESIAN_POINT('Ctrl Pts',(13.4546674310278,-30.6665180976751,1.33837720683381));
#5851=CARTESIAN_POINT('Ctrl Pts',(13.5009280586962,-30.6711994291191,1.30011245980355));
#5852=CARTESIAN_POINT('Ctrl Pts',(13.5454051453913,-30.6764974334051,1.26048896755351));
#5853=CARTESIAN_POINT('Ctrl Pts',(13.5552471366691,-30.677669787888,1.25172099073441));
#5854=CARTESIAN_POINT('Ctrl Pts',(13.5650019652857,-30.6788722883136,1.24288658001281));
#5855=CARTESIAN_POINT('Ctrl Pts',(13.5746675343456,-30.6801044271852,1.2339885196899));
#5856=CARTESIAN_POINT('Ctrl Pts',(13.6183515138192,-30.6856731349188,1.19377333090038));
#5857=CARTESIAN_POINT('Ctrl Pts',(13.6608895145213,-30.6923518043743,1.1518685325288));
#5858=CARTESIAN_POINT('Ctrl Pts',(13.7020166722461,-30.7001293046305,1.10846850103127));
#5859=CARTESIAN_POINT('Ctrl Pts',(13.7431581927038,-30.7079095210034,1.06505331305085));
#5860=CARTESIAN_POINT('Ctrl Pts',(13.7828872078749,-30.7167893284822,1.0201422978762));
#5861=CARTESIAN_POINT('Ctrl Pts',(13.820963799237,-30.7267327043492,0.97396820682354));
#5862=CARTESIAN_POINT('Ctrl Pts',(13.8590741853685,-30.736684905431,0.927753134089042));
#5863=CARTESIAN_POINT('Ctrl Pts',(13.8955286265147,-30.7477024656982,0.880273333152889));
#5864=CARTESIAN_POINT('Ctrl Pts',(13.930121366925,-30.7597251338659,0.831792563200548));
#5865=CARTESIAN_POINT('Ctrl Pts',(13.9646877586768,-30.7717386445869,0.783348720164987));
#5866=CARTESIAN_POINT('Ctrl Pts',(13.9973948520632,-30.7847555422319,0.73390612619343));
#5867=CARTESIAN_POINT('Ctrl Pts',(14.0280797616702,-30.7986938115477,0.683748572310606));
#5868=CARTESIAN_POINT('Ctrl Pts',(14.0587471951691,-30.8126241425412,0.633619584874411));
#5869=CARTESIAN_POINT('Ctrl Pts',(14.0873944899397,-30.8274745364751,0.582777184222982));
#5870=CARTESIAN_POINT('Ctrl Pts',(14.1139066028877,-30.84314462319,0.531514551850337));
#5871=CARTESIAN_POINT('Ctrl Pts',(14.1197732637638,-30.8466121357506,0.52017103953455));
#5872=CARTESIAN_POINT('Ctrl Pts',(14.1255355657245,-30.8501197225158,0.508806964006327));
#5873=CARTESIAN_POINT('Ctrl Pts',(14.1311925920689,-30.8536661946033,0.497425511654571));
#5874=CARTESIAN_POINT('Ctrl Pts',(14.1567597802163,-30.8696946366858,0.445986519513703));
#5875=CARTESIAN_POINT('Ctrl Pts',(14.1806788242274,-30.8871229657987,0.39369664540894));
#5876=CARTESIAN_POINT('Ctrl Pts',(14.2027770927318,-30.9058868003686,0.340828125588002));
#5877=CARTESIAN_POINT('Ctrl Pts',(14.2248830785583,-30.9246571877848,0.287941142628218));
#5878=CARTESIAN_POINT('Ctrl Pts',(14.2451665594135,-30.9447638797351,0.234475768277207));
#5879=CARTESIAN_POINT('Ctrl Pts',(14.263491348928,-30.9661109637157,0.180724039815161));
#5880=CARTESIAN_POINT('Ctrl Pts',(14.2818324025568,-30.9874769942394,0.126924604160708));
#5881=CARTESIAN_POINT('Ctrl Pts',(14.2982109611228,-31.0100853707185,0.0728390372992588));
#5882=CARTESIAN_POINT('Ctrl Pts',(14.3125330760228,-31.0338112899811,0.018769220635499));
#5883=CARTESIAN_POINT('Ctrl Pts',(14.3268442820297,-31.0575191376449,-0.0352594120376883));
#5884=CARTESIAN_POINT('Ctrl Pts',(14.3391020279638,-31.0823424715467,-0.0892715721449215));
#5885=CARTESIAN_POINT('Ctrl Pts',(14.349258645209,-31.1081327559841,-0.142968160449075));
#5886=CARTESIAN_POINT('Ctrl Pts',(14.3594094779122,-31.1339083519698,-0.196634166704025));
#5887=CARTESIAN_POINT('Ctrl Pts',(14.367461600142,-31.1606493743139,-0.249984259986138));
#5888=CARTESIAN_POINT('Ctrl Pts',(14.373414373612,-31.1881894012107,-0.302732839444724));
#5889=CARTESIAN_POINT('Ctrl Pts',(14.3747316169147,-31.194283521232,-0.3144051655241));
#5890=CARTESIAN_POINT('Ctrl Pts',(14.3759462441235,-31.2004167092395,-0.326048111329434));
#5891=CARTESIAN_POINT('Ctrl Pts',(14.3770585529418,-31.2065870752141,-0.337658719487507));
#5892=CARTESIAN_POINT('Ctrl Pts',(14.3820856832934,-31.2344743251941,-0.390133391728236));
#5893=CARTESIAN_POINT('Ctrl Pts',(14.3853273896913,-31.2638407207439,-0.442451690706376));
#5894=CARTESIAN_POINT('Ctrl Pts',(14.3867233958332,-31.2945570120615,-0.494317440110226));
#5895=CARTESIAN_POINT('Ctrl Pts',(14.3881198894988,-31.3252840303516,-0.546201302458348));
#5896=CARTESIAN_POINT('Ctrl Pts',(14.3876692117264,-31.3573615943671,-0.59763156288618));
#5897=CARTESIAN_POINT('Ctrl Pts',(14.3853509125449,-31.3906269711632,-0.64831473971449));
#5898=CARTESIAN_POINT('Ctrl Pts',(14.3830305557636,-31.4239218725492,-0.699042900251102));
#5899=CARTESIAN_POINT('Ctrl Pts',(14.3788392239111,-31.4584062807987,-0.749021923205321));
#5900=CARTESIAN_POINT('Ctrl Pts',(14.3727980277331,-31.4938889631939,-0.797971596267801));
#5901=CARTESIAN_POINT('Ctrl Pts',(14.3667614330238,-31.5293446190785,-0.84688398525904));
#5902=CARTESIAN_POINT('Ctrl Pts',(14.3588779192251,-31.5657965147087,-0.894767940776057));
#5903=CARTESIAN_POINT('Ctrl Pts',(14.3492093765965,-31.6030328605358,-0.941368295641471));
#5904=CARTESIAN_POINT('Ctrl Pts',(14.3395463405345,-31.640247998987,-0.987942110006656));
#5905=CARTESIAN_POINT('Ctrl Pts',(14.3281005770856,-31.6782461308766,-1.03323325564961));
#5906=CARTESIAN_POINT('Ctrl Pts',(14.3149716746741,-31.7168029684803,-1.07702027911411));
#5907=CARTESIAN_POINT('Ctrl Pts',(14.3120664811774,-31.7253349135243,-1.08670957162503));
#5908=CARTESIAN_POINT('Ctrl Pts',(14.3090790082963,-31.7338941851498,-1.09632535949905));
#5909=CARTESIAN_POINT('Ctrl Pts',(14.3060105618214,-31.7424783113183,-1.10586550012264));
#5910=CARTESIAN_POINT('Ctrl Pts',(14.2921425782612,-31.7812746604017,-1.14898260006689));
#5911=CARTESIAN_POINT('Ctrl Pts',(14.276743966429,-31.8214030486997,-1.19096704316451));
#5912=CARTESIAN_POINT('Ctrl Pts',(14.2598646740236,-31.8626705885533,-1.23155737439071));
#5913=CARTESIAN_POINT('Ctrl Pts',(14.2429794869057,-31.9039525401653,-1.27216188087552));
#5914=CARTESIAN_POINT('Ctrl Pts',(14.2246126805971,-31.9463739858142,-1.31137063355188));
#5915=CARTESIAN_POINT('Ctrl Pts',(14.204848622758,-31.9897116760678,-1.34894683398738));
#5916=CARTESIAN_POINT('Ctrl Pts',(14.1850670233862,-32.0330878305638,-1.38655638507153));
#5917=CARTESIAN_POINT('Ctrl Pts',(14.1638859123477,-32.0773812923998,-1.42252990566966));
#5918=CARTESIAN_POINT('Ctrl Pts',(14.1414219230224,-32.1223456788394,-1.4566643520522));
#5919=CARTESIAN_POINT('Ctrl Pts',(14.1189750441073,-32.1672758167275,-1.49077279885072));
#5920=CARTESIAN_POINT('Ctrl Pts',(14.0952475818026,-32.2128752202925,-1.52304454512923));
#5921=CARTESIAN_POINT('Ctrl Pts',(14.0703836278415,-32.2588846409427,-1.55331889475902));
#5922=CARTESIAN_POINT('Ctrl Pts',(14.0455338347545,-32.3048678576505,-1.58357600210875));
#5923=CARTESIAN_POINT('Ctrl Pts',(14.0195492678734,-32.3512599716156,-1.61183773325817));
#5924=CARTESIAN_POINT('Ctrl Pts',(13.9925957131064,-32.3977984759783,-1.63799064371848));
#5925=CARTESIAN_POINT('Ctrl Pts',(13.9866313689773,-32.408096622463,-1.64377781944764));
#5926=CARTESIAN_POINT('Ctrl Pts',(13.980619648127,-32.4184019444672,-1.64946192467185));
#5927=CARTESIAN_POINT('Ctrl Pts',(13.9745624584517,-32.4287116223265,-1.65504205590818));
#5928=CARTESIAN_POINT('Ctrl Pts',(13.9471867139074,-32.4753066808503,-1.6802617131151));
#5929=CARTESIAN_POINT('Ctrl Pts',(13.9188767468619,-32.5228894435563,-1.70359676647094));
#5930=CARTESIAN_POINT('Ctrl Pts',(13.8897687667337,-32.5712172195584,-1.72487226661204));
#5931=CARTESIAN_POINT('Ctrl Pts',(13.8606506212992,-32.6195618729473,-1.74615519674216));
#5932=CARTESIAN_POINT('Ctrl Pts',(13.83073422553,-32.6686514771803,-1.76537666733525));
#5933=CARTESIAN_POINT('Ctrl Pts',(13.8001770855324,-32.7182205563234,-1.78240346403942));
#5934=CARTESIAN_POINT('Ctrl Pts',(13.7695928246328,-32.7678336303605,-1.79944537282816));
#5935=CARTESIAN_POINT('Ctrl Pts',(13.7383670797744,-32.8179263642364,-1.81428839412959));
#5936=CARTESIAN_POINT('Ctrl Pts',(13.7066735508278,-32.868219427861,-1.82684686809474));
#5937=CARTESIAN_POINT('Ctrl Pts',(13.6750041622632,-32.9184741841778,-1.83939577649969));
#5938=CARTESIAN_POINT('Ctrl Pts',(13.642868150994,-32.9689282657509,-1.84966349840251));
#5939=CARTESIAN_POINT('Ctrl Pts',(13.6104481718153,-33.0193001595944,-1.85761563656222));
#5940=CARTESIAN_POINT('Ctrl Pts',(13.5780466569263,-33.0696433649174,-1.86556324570659));
#5941=CARTESIAN_POINT('Ctrl Pts',(13.5453619571861,-33.119903802392,-1.87119797990078));
#5942=CARTESIAN_POINT('Ctrl Pts',(13.5125789155374,-33.1698079625751,-1.87453687269571));
#5943=CARTESIAN_POINT('Ctrl Pts',(13.5053246092432,-33.1808508690632,-1.8752757105155));
#5944=CARTESIAN_POINT('Ctrl Pts',(13.4980654819439,-33.1918763815167,-1.87590232633986));
#5945=CARTESIAN_POINT('Ctrl Pts',(13.4908035184053,-33.2028816358906,-1.87641723476233));
#5946=CARTESIAN_POINT('Ctrl Pts',(13.457982743529,-33.2526203841424,-1.87874438682335));
#5947=CARTESIAN_POINT('Ctrl Pts',(13.4250476365344,-33.3028734726432,-1.87880825693469));
#5948=CARTESIAN_POINT('Ctrl Pts',(13.392179621086,-33.3533721060497,-1.87655505226088));
#5949=CARTESIAN_POINT('Ctrl Pts',(13.3593001272239,-33.403888374966,-1.87430106070611));
#5950=CARTESIAN_POINT('Ctrl Pts',(13.3264882189081,-33.4546497041472,-1.86972820122915));
#5951=CARTESIAN_POINT('Ctrl Pts',(13.2939283755408,-33.5053750446201,-1.86283322829481));
#5952=CARTESIAN_POINT('Ctrl Pts',(13.261339633778,-33.5561454062231,-1.85593213574705));
#5953=CARTESIAN_POINT('Ctrl Pts',(13.2290038633833,-33.6068790136412,-1.84670481534519));
#5954=CARTESIAN_POINT('Ctrl Pts',(13.1971020718565,-33.6572923177224,-1.83519995710444));
#5955=CARTESIAN_POINT('Ctrl Pts',(13.1652245793415,-33.7076672229108,-1.82370386190406));
#5956=CARTESIAN_POINT('Ctrl Pts',(13.1337808348958,-33.7577216240468,-1.8099339111831));
#5957=CARTESIAN_POINT('Ctrl Pts',(13.1029407800775,-33.8071813481355,-1.79398881938374));
#5958=CARTESIAN_POINT('Ctrl Pts',(13.0721182897278,-33.8566129032153,-1.77805280886091));
#5959=CARTESIAN_POINT('Ctrl Pts',(13.0418991711865,-33.905449836721,-1.75994451788745));
#5960=CARTESIAN_POINT('Ctrl Pts',(13.0124364095004,-33.9534370323736,-1.73980808435037));
#5961=CARTESIAN_POINT('Ctrl Pts',(13.0059168223358,-33.9640557485747,-1.73535224836903));
#5962=CARTESIAN_POINT('Ctrl Pts',(12.9994341942536,-33.9746329489963,-1.7307972658443));
#5963=CARTESIAN_POINT('Ctrl Pts',(12.9929900464286,-33.9851660372479,-1.72614496752461));
#5964=CARTESIAN_POINT('Ctrl Pts',(12.9638654269088,-34.0327708092098,-1.70511869343321));
#5965=CARTESIAN_POINT('Ctrl Pts',(12.9355074609201,-34.0803812841189,-1.68189873004098));
#5966=CARTESIAN_POINT('Ctrl Pts',(12.9080927836634,-34.1277314312526,-1.65656309537146));
#5967=CARTESIAN_POINT('Ctrl Pts',(12.8806685324485,-34.1750981143581,-1.63121861280245));
#5968=CARTESIAN_POINT('Ctrl Pts',(12.8541886802717,-34.2222036292231,-1.60375713415714));
#5969=CARTESIAN_POINT('Ctrl Pts',(12.8288131722874,-34.2687810917287,-1.57430602553505));
#5970=CARTESIAN_POINT('Ctrl Pts',(12.8034151423441,-34.3153998939271,-1.54482877766629));
#5971=CARTESIAN_POINT('Ctrl Pts',(12.7791238088676,-34.3614890435249,-1.51335869953241));
#5972=CARTESIAN_POINT('Ctrl Pts',(12.7560762807596,-34.4067903362379,-1.48006918735819));
#5973=CARTESIAN_POINT('Ctrl Pts',(12.7330463075327,-34.4520571237836,-1.44680503119733));
#5974=CARTESIAN_POINT('Ctrl Pts',(12.7112585337638,-34.4965366476502,-1.41172471547026));
#5975=CARTESIAN_POINT('Ctrl Pts',(12.6908214294875,-34.539990225443,-1.37504051469644));
#5976=CARTESIAN_POINT('Ctrl Pts',(12.6703959648427,-34.5834190549336,-1.33837720683257));
#5977=CARTESIAN_POINT('Ctrl Pts',(12.6513198029624,-34.6258225994116,-1.30011245980211));
#5978=CARTESIAN_POINT('Ctrl Pts',(12.6336694659159,-34.666989888519,-1.26048896755186));
#5979=CARTESIAN_POINT('Ctrl Pts',(12.6297637590416,-34.6760994802303,-1.2517209907333));
#5980=CARTESIAN_POINT('Ctrl Pts',(12.6259277406503,-34.6851486598341,-1.24288658001226));
#5981=CARTESIAN_POINT('Ctrl Pts',(12.6221620196843,-34.6941353576172,-1.23398851968991));
#5982=CARTESIAN_POINT('Ctrl Pts',(12.6051426723111,-34.7347511474464,-1.19377333090049));
#5983=CARTESIAN_POINT('Ctrl Pts',(12.589657569372,-34.7749294714083,-1.15186853252901));
#5984=CARTESIAN_POINT('Ctrl Pts',(12.5758295033095,-34.8144353849114,-1.10846850103161));
#5985=CARTESIAN_POINT('Ctrl Pts',(12.5619966081066,-34.8539550949644,-1.06505331305148));
#5986=CARTESIAN_POINT('Ctrl Pts',(12.5498222393785,-34.8928013351089,-1.02014229787715));
#5987=CARTESIAN_POINT('Ctrl Pts',(12.5393951597977,-34.9307483184514,-0.973968206824812));
#5988=CARTESIAN_POINT('Ctrl Pts',(12.5289588256923,-34.9687289815301,-0.927753134090402));
#5989=CARTESIAN_POINT('Ctrl Pts',(12.5202730921983,-35.0058082337771,-0.88027333315432));
#5990=CARTESIAN_POINT('Ctrl Pts',(12.5133886580476,-35.0417777598427,-0.831792563202067));
#5991=CARTESIAN_POINT('Ctrl Pts',(12.5065094676445,-35.0777198885782,-0.783348720165615));
#5992=CARTESIAN_POINT('Ctrl Pts',(12.5014288849903,-35.1125535111578,-0.733906126193128));
#5993=CARTESIAN_POINT('Ctrl Pts',(12.498157325499,-35.1460965570489,-0.683748572309347));
#5994=CARTESIAN_POINT('Ctrl Pts',(12.4948876292731,-35.1796204990247,-0.633619584872897));
#5995=CARTESIAN_POINT('Ctrl Pts',(12.4934248002908,-35.2118549810128,-0.582777184221212));
#5996=CARTESIAN_POINT('Ctrl Pts',(12.4937394369914,-35.2426501876914,-0.531514551848308));
#5997=CARTESIAN_POINT('Ctrl Pts',(12.4938090605188,-35.2494646213253,-0.520171039533193));
#5998=CARTESIAN_POINT('Ctrl Pts',(12.4939655687831,-35.2562087145898,-0.508806964005651));
#5999=CARTESIAN_POINT('Ctrl Pts',(12.4942083905325,-35.2628810791572,-0.497425511654571));
#6000=CARTESIAN_POINT('Ctrl Pts',(12.4953058344853,-35.2930371346372,-0.445986519514037));
#6001=CARTESIAN_POINT('Ctrl Pts',(12.4984396882371,-35.3224657989414,-0.393696645409609));
#6002=CARTESIAN_POINT('Ctrl Pts',(12.5036405113948,-35.3509853781306,-0.340828125589025));
#6003=CARTESIAN_POINT('Ctrl Pts',(12.5088431508228,-35.3795149171403,-0.287941142629085));
#6004=CARTESIAN_POINT('Ctrl Pts',(12.5161143164102,-35.4071342728133,-0.234475768277919));
#6005=CARTESIAN_POINT('Ctrl Pts',(12.5254390386769,-35.4336775480422,-0.180724039815708));
#6006=CARTESIAN_POINT('Ctrl Pts',(12.5347720370741,-35.460244381679,-0.126924604161013));
#6007=CARTESIAN_POINT('Ctrl Pts',(12.5461621861603,-35.4857328177141,-0.0728390372993232));
#6008=CARTESIAN_POINT('Ctrl Pts',(12.55954837752,-35.5099990926848,-0.0187692206353172));
#6009=CARTESIAN_POINT('Ctrl Pts',(12.5729243728623,-35.5342468844775,0.035259412037625));
#6010=CARTESIAN_POINT('Ctrl Pts',(12.5882931376608,-35.5572740708003,0.0892715721446082));
#6011=CARTESIAN_POINT('Ctrl Pts',(12.6055498705317,-35.5789651015697,0.142968160448519));
#6012=CARTESIAN_POINT('Ctrl Pts',(12.6227967751013,-35.6006437785531,0.196634166703384));
#6013=CARTESIAN_POINT('Ctrl Pts',(12.6419291186596,-35.6209876321305,0.249984259985418));
#6014=CARTESIAN_POINT('Ctrl Pts',(12.662803094838,-35.6399128986269,0.302732839443923));
#6015=CARTESIAN_POINT('Ctrl Pts',(12.6674221359389,-35.6441007248007,0.314405165523565));
#6016=CARTESIAN_POINT('Ctrl Pts',(12.6721263189554,-35.6482192168235,0.326048111329166));
#6017=CARTESIAN_POINT('Ctrl Pts',(12.676913858231,-35.6522676875044,0.337658719487503));
#6018=CARTESIAN_POINT('Ctrl Pts',(12.6985513599797,-35.6705649350872,0.390133391728747));
#6019=CARTESIAN_POINT('Ctrl Pts',(12.7223625513447,-35.6880555329546,0.4424516907074));
#6020=CARTESIAN_POINT('Ctrl Pts',(12.7482656368651,-35.7046226553962,0.49431744011175));
#6021=CARTESIAN_POINT('Ctrl Pts',(12.7741777684545,-35.7211955635321,0.546201302460495));
#6022=CARTESIAN_POINT('Ctrl Pts',(12.80218309267,-35.7368440471401,0.597631562888927));
#6023=CARTESIAN_POINT('Ctrl Pts',(12.8321509036332,-35.7514690295535,0.648314739717827));
#6024=CARTESIAN_POINT('Ctrl Pts',(12.8621453124406,-35.766106992328,0.699042900254311));
#6025=CARTESIAN_POINT('Ctrl Pts',(12.8941053519454,-35.7797193965928,0.749021923208405));
#6026=CARTESIAN_POINT('Ctrl Pts',(12.9278548543831,-35.7922289084309,0.797971596270746));
#6027=CARTESIAN_POINT('Ctrl Pts',(12.9615786504418,-35.8047288920026,0.846883985262079));
#6028=CARTESIAN_POINT('Ctrl Pts',(12.9970886749731,-35.8161275165969,0.89476794077918));
#6029=CARTESIAN_POINT('Ctrl Pts',(13.034170567718,-35.8263724859765,0.941368295644665));
#6030=CARTESIAN_POINT('Ctrl Pts',(13.0712313410528,-35.8366116204946,0.987942110009404));
#6031=CARTESIAN_POINT('Ctrl Pts',(13.1098615702898,-35.8456983645268,1.03323325565192));
#6032=CARTESIAN_POINT('Ctrl Pts',(13.1498172223497,-35.8536068203165,1.077020279116));
#6033=CARTESIAN_POINT('Ctrl Pts',(13.1586587002493,-35.8553568214672,1.08670957162628));
#6034=CARTESIAN_POINT('Ctrl Pts',(13.1675649833548,-35.8570492298717,1.09632535949967));
#6035=CARTESIAN_POINT('Ctrl Pts',(13.1765332779228,-35.8586839403584,1.10586550012264));
#6036=CARTESIAN_POINT('Ctrl Pts',(13.2170658935831,-35.8660720888377,1.14898260006675));
#6037=CARTESIAN_POINT('Ctrl Pts',(13.2595174031781,-35.872800693957,1.19096704316422));
#6038=CARTESIAN_POINT('Ctrl Pts',(13.3036957872455,-35.8788165678628,1.23155737439029));
#6039=CARTESIAN_POINT('Ctrl Pts',(13.3478895996175,-35.8848345426769,1.27216188087445));
#6040=CARTESIAN_POINT('Ctrl Pts',(13.3938110523682,-35.8901391446517,1.31137063355021));
#6041=CARTESIAN_POINT('Ctrl Pts',(13.4412246219879,-35.8946918136079,1.34894683398517));
#6042=CARTESIAN_POINT('Ctrl Pts',(13.4886802733859,-35.8992485232725,1.38655638506951));
#6043=CARTESIAN_POINT('Ctrl Pts',(13.5376300920768,-35.9030518739508,1.42252990566782));
#6044=CARTESIAN_POINT('Ctrl Pts',(13.5878023876618,-35.9060796817446,1.45666435205053));
#6045=CARTESIAN_POINT('Ctrl Pts',(13.6379364679262,-35.9091051833125,1.49077279884923));
#6046=CARTESIAN_POINT('Ctrl Pts',(13.6892904409634,-35.9113562999719,1.52304454512792));
#6047=CARTESIAN_POINT('Ctrl Pts',(13.7415677450407,-35.9128281945281,1.55331889475788));
#6048=CARTESIAN_POINT('Ctrl Pts',(13.7938152754001,-35.91429925079,1.58357600210724));
#6049=CARTESIAN_POINT('Ctrl Pts',(13.8469843080689,-35.9149920127471,1.61183773325636));
#6050=CARTESIAN_POINT('Ctrl Pts',(13.9007646124839,-35.914918801778,1.63799064371642));
#6051=CARTESIAN_POINT('Ctrl Pts',(13.9126652410174,-35.9149026014877,1.64377781944629));
#6052=CARTESIAN_POINT('Ctrl Pts',(13.9245957720938,-35.914848959513,1.64946192467119));
#6053=CARTESIAN_POINT('Ctrl Pts',(13.9365528098639,-35.9147581183082,1.65504205590817));
#6054=CARTESIAN_POINT('Ctrl Pts',(13.9905931865086,-35.9143475573472,1.68026171311514));
#6055=CARTESIAN_POINT('Ctrl Pts',(14.0459560513171,-35.9136217880585,1.70359676647103));
#6056=CARTESIAN_POINT('Ctrl Pts',(14.1023631231076,-35.9125774258157,1.72487226661217));
#6057=CARTESIAN_POINT('Ctrl Pts',(14.1587898937969,-35.9115326988529,1.74615519674234));
#6058=CARTESIAN_POINT('Ctrl Pts',(14.2162609360092,-35.9101691422435,1.76537666733546));
#6059=CARTESIAN_POINT('Ctrl Pts',(14.2744675877883,-35.9084904223101,1.78240346403966));
#6060=CARTESIAN_POINT('Ctrl Pts',(14.3327259007139,-35.9068102124337,1.79944537282833));
#6061=CARTESIAN_POINT('Ctrl Pts',(14.3917203532245,-35.9048142910721,1.81428839412971));
#6062=CARTESIAN_POINT('Ctrl Pts',(14.4511221884307,-35.9025134216811,1.82684686809481));
#6063=CARTESIAN_POINT('Ctrl Pts',(14.5104787783442,-35.9002143048202,1.83939577649974));
#6064=CARTESIAN_POINT('Ctrl Pts',(14.5702413003456,-35.8976107434714,1.84966349840254));
#6065=CARTESIAN_POINT('Ctrl Pts',(14.6300746296402,-35.8947201648342,1.85761563656223));
#6066=CARTESIAN_POINT('Ctrl Pts',(14.6898738818023,-35.8918312324807,1.8655632457066));
#6067=CARTESIAN_POINT('Ctrl Pts',(14.7497430473307,-35.888655670928,1.87119797990078));
#6068=CARTESIAN_POINT('Ctrl Pts',(14.8093528386281,-35.8852168041384,1.8745368726957));
#6069=CARTESIAN_POINT('Ctrl Pts',(14.8225434293255,-35.8844558438449,1.87527571051549));
#6070=CARTESIAN_POINT('Ctrl Pts',(14.8357213668496,-35.8836820114211,1.87590232633985));
#6071=CARTESIAN_POINT('Ctrl Pts',(14.8488831784817,-35.8828955937023,1.87641723476232));
#6072=CARTESIAN_POINT('Ctrl Pts',(14.9083685854582,-35.8793413430134,1.87874438682333));
#6073=CARTESIAN_POINT('Ctrl Pts',(14.9683565902156,-35.8759452479302,1.87880825693468));
#6074=CARTESIAN_POINT('Ctrl Pts',(15.0285236973261,-35.8727300282831,1.87655505226089));
#6075=CARTESIAN_POINT('Ctrl Pts',(15.0887118164435,-35.8695136857931,1.87430106070612));
#6076=CARTESIAN_POINT('Ctrl Pts',(15.1490783712027,-35.8664784042356,1.86972820122912));
#6077=CARTESIAN_POINT('Ctrl Pts',(15.209287726352,-35.8636434229726,1.8628332282947));
#6078=CARTESIAN_POINT('Ctrl Pts',(15.2695505201408,-35.8608059255302,1.85593213574694));
#6079=CARTESIAN_POINT('Ctrl Pts',(15.3296549981877,-35.8581691306264,1.84670481534507));
#6080=CARTESIAN_POINT('Ctrl Pts',(15.3892650959741,-35.8557480207786,1.83519995710432));
#6081=CARTESIAN_POINT('Ctrl Pts',(15.4488297898389,-35.8533287550459,1.82370386190375));
#6082=CARTESIAN_POINT('Ctrl Pts',(15.5079000450177,-35.8511248741338,1.80993391118252));
#6083=CARTESIAN_POINT('Ctrl Pts',(15.5661534499527,-35.8491464652513,1.79398881938283));
#6084=CARTESIAN_POINT('Ctrl Pts',(15.6243736775756,-35.8471691831405,1.77805280885979));
#6085=CARTESIAN_POINT('Ctrl Pts',(15.6817772619055,-35.8454171255565,1.7599445178861));
#6086=CARTESIAN_POINT('Ctrl Pts',(15.7380667732405,-35.8438952232971,1.73980808434875));
#6087=CARTESIAN_POINT('Ctrl Pts',(15.750522644807,-35.8435584532909,1.73535224836793));
#6088=CARTESIAN_POINT('Ctrl Pts',(15.7629240831126,-35.8432329328993,1.73079726584374));
#6089=CARTESIAN_POINT('Ctrl Pts',(15.7752680790298,-35.842918681303,1.72614496752462));
#6090=CARTESIAN_POINT('Ctrl Pts',(15.8310573306496,-35.8414984069043,1.70511869343338));
#6091=CARTESIAN_POINT('Ctrl Pts',(15.8864681944011,-35.8407449254129,1.68189873004136));
#6092=CARTESIAN_POINT('Ctrl Pts',(15.9411819633197,-35.8406781920389,1.65656309537207));
#6093=CARTESIAN_POINT('Ctrl Pts',(15.9959148397889,-35.8406114353597,1.6312186128034));
#6094=CARTESIAN_POINT('Ctrl Pts',(16.0499493384081,-35.8412319681187,1.60375713415847));
#6095=CARTESIAN_POINT('Ctrl Pts',(16.1029743581733,-35.8425448648231,1.57430602553681));
#6096=CARTESIAN_POINT('Ctrl Pts',(16.1560464401428,-35.8438589267853,1.54482877766814));
#6097=CARTESIAN_POINT('Ctrl Pts',(16.2081064812716,-35.8458665897017,1.51335869953437));
#6098=CARTESIAN_POINT('Ctrl Pts',(16.2588623156393,-35.8485574912222,1.48006918736026));
#6099=CARTESIAN_POINT('Ctrl Pts',(16.3095794902158,-35.8512463431322,1.44680503119899));
#6100=CARTESIAN_POINT('Ctrl Pts',(16.3589937747177,-35.8546173394896,1.41172471547146));
#6101=CARTESIAN_POINT('Ctrl Pts',(16.4068442291105,-35.858645076903,1.37504051469712));
#6102=CARTESIAN_POINT('Ctrl Pts',(16.4546674310271,-35.8626705203817,1.33837720683427));
#6103=CARTESIAN_POINT('Ctrl Pts',(16.5009280586945,-35.8673518518255,1.30011245980493));
#6104=CARTESIAN_POINT('Ctrl Pts',(16.5454051453886,-35.8726498561114,1.26048896755585));
#6105=CARTESIAN_POINT('Ctrl Pts',(16.5552471366674,-35.8738222105944,1.25172099073598));
#6106=CARTESIAN_POINT('Ctrl Pts',(16.5650019652848,-35.8750247110202,1.24288658001361));
#6107=CARTESIAN_POINT('Ctrl Pts',(16.5746675343456,-35.8762568498918,1.2339885196899));
#6108=CARTESIAN_POINT('Ctrl Pts',(16.6183515138188,-35.8818255576253,1.19377333090077));
#6109=CARTESIAN_POINT('Ctrl Pts',(16.6608895145205,-35.8885042270808,1.15186853252961));
#6110=CARTESIAN_POINT('Ctrl Pts',(16.7020166722449,-35.8962817273369,1.10846850103254));
#6111=CARTESIAN_POINT('Ctrl Pts',(16.7431581927026,-35.9040619437098,1.06505331305215));
#6112=CARTESIAN_POINT('Ctrl Pts',(16.7828872078737,-35.9129417511886,1.02014229787755));
#6113=CARTESIAN_POINT('Ctrl Pts',(16.8209637992359,-35.9228851270556,0.973968206824924));
#6114=CARTESIAN_POINT('Ctrl Pts',(16.8590741853672,-35.9328373281373,0.927753134090565));
#6115=CARTESIAN_POINT('Ctrl Pts',(16.8955286265134,-35.9438548884045,0.880273333154538));
#6116=CARTESIAN_POINT('Ctrl Pts',(16.9301213669236,-35.9558775565721,0.831792563202344));
#6117=CARTESIAN_POINT('Ctrl Pts',(16.9646877586765,-35.9678910672934,0.783348720165493));
#6118=CARTESIAN_POINT('Ctrl Pts',(16.9973948520637,-35.9809079649387,0.733906126192583));
#6119=CARTESIAN_POINT('Ctrl Pts',(17.0280797616715,-35.9948462342549,0.683748572308376));
#6120=CARTESIAN_POINT('Ctrl Pts',(17.0587471951712,-36.0087765652489,0.633619584870814));
#6121=CARTESIAN_POINT('Ctrl Pts',(17.0873944899424,-36.0236269591832,0.582777184217972));
#6122=CARTESIAN_POINT('Ctrl Pts',(17.113906602891,-36.0392970458986,0.531514551843913));
#6123=CARTESIAN_POINT('Ctrl Pts',(17.1197732637659,-36.0427645584586,0.520171039530256));
#6124=CARTESIAN_POINT('Ctrl Pts',(17.1255355657255,-36.0462721452231,0.508806964004177));
#6125=CARTESIAN_POINT('Ctrl Pts',(17.1311925920688,-36.0498186173099,0.497425511654565));
#6126=CARTESIAN_POINT('Ctrl Pts',(17.1567597802163,-36.0658470593925,0.445986519513662));
#6127=CARTESIAN_POINT('Ctrl Pts',(17.1806788242274,-36.0832753885054,0.393696645408846));
#6128=CARTESIAN_POINT('Ctrl Pts',(17.2027770927318,-36.1020392230754,0.340828125587867));
#6129=CARTESIAN_POINT('Ctrl Pts',(17.2248830785582,-36.1208096104915,0.287941142628222));
#6130=CARTESIAN_POINT('Ctrl Pts',(17.2451665594134,-36.1409163024417,0.234475768277352));
#6131=CARTESIAN_POINT('Ctrl Pts',(17.2634913489279,-36.1622633864223,0.180724039815448));
#6132=CARTESIAN_POINT('Ctrl Pts',(17.2818324025569,-36.1836294169462,0.126924604160518));
#6133=CARTESIAN_POINT('Ctrl Pts',(17.2982109611229,-36.2062377934255,0.0728390372985996));
#6134=CARTESIAN_POINT('Ctrl Pts',(17.312533076023,-36.2299637126883,0.0187692206343586));
#6135=CARTESIAN_POINT('Ctrl Pts',(17.32684428203,-36.2536715603521,-0.035259412038812));
#6136=CARTESIAN_POINT('Ctrl Pts',(17.339102027964,-36.2784948942539,-0.0892715721460276));
#6137=CARTESIAN_POINT('Ctrl Pts',(17.3492586452091,-36.3042851786913,-0.142968160450158));
#6138=CARTESIAN_POINT('Ctrl Pts',(17.3594094779124,-36.3300607746771,-0.19663416670548));
#6139=CARTESIAN_POINT('Ctrl Pts',(17.3674616001422,-36.3568017970215,-0.249984259987957));
#6140=CARTESIAN_POINT('Ctrl Pts',(17.3734143736122,-36.3843418239185,-0.302732839446895));
#6141=CARTESIAN_POINT('Ctrl Pts',(17.3747316169148,-36.3904359439394,-0.314405165525541));
#6142=CARTESIAN_POINT('Ctrl Pts',(17.3759462441235,-36.3965691319466,-0.326048111330149));
#6143=CARTESIAN_POINT('Ctrl Pts',(17.3770585529417,-36.4027394979208,-0.3376587194875));
#6144=CARTESIAN_POINT('Ctrl Pts',(17.3820856832934,-36.4306267479012,-0.390133391729108));
#6145=CARTESIAN_POINT('Ctrl Pts',(17.3853273896914,-36.4599931434515,-0.442451690708116));
#6146=CARTESIAN_POINT('Ctrl Pts',(17.3867233958333,-36.4907094347696,-0.49431744011282));
#6147=CARTESIAN_POINT('Ctrl Pts',(17.3881198894988,-36.5214364530601,-0.546201302461415));
#6148=CARTESIAN_POINT('Ctrl Pts',(17.3876692117263,-36.553514017076,-0.597631562889711));
#6149=CARTESIAN_POINT('Ctrl Pts',(17.3853509125446,-36.5867793938725,-0.648314739718458));
#6150=CARTESIAN_POINT('Ctrl Pts',(17.3830305557632,-36.6200742952585,-0.699042900255015));
#6151=CARTESIAN_POINT('Ctrl Pts',(17.3788392239107,-36.654558703508,-0.749021923209178));
#6152=CARTESIAN_POINT('Ctrl Pts',(17.3727980277326,-36.6900413859033,-0.797971596271591));
#6153=CARTESIAN_POINT('Ctrl Pts',(17.3667614330232,-36.7254970417877,-0.846883985262451));
#6154=CARTESIAN_POINT('Ctrl Pts',(17.3588779192245,-36.7619489374177,-0.894767940779093));
#6155=CARTESIAN_POINT('Ctrl Pts',(17.3492093765959,-36.7991852832446,-0.941368295644146));
#6156=CARTESIAN_POINT('Ctrl Pts',(17.3395463405339,-36.8364004216957,-0.987942110009194));
#6157=CARTESIAN_POINT('Ctrl Pts',(17.3281005770849,-36.8743985535853,-1.03323325565201));
#6158=CARTESIAN_POINT('Ctrl Pts',(17.3149716746734,-36.912955391189,-1.07702027911637));
#6159=CARTESIAN_POINT('Ctrl Pts',(17.3120664811769,-36.9214873362323,-1.08670957162653));
#6160=CARTESIAN_POINT('Ctrl Pts',(17.309079008296,-36.9300466078572,-1.09632535949979));
#6161=CARTESIAN_POINT('Ctrl Pts',(17.3060105618214,-36.9386307340249,-1.10586550012263));
#6162=CARTESIAN_POINT('Ctrl Pts',(17.2921425782612,-36.9774270831083,-1.14898260006685));
#6163=CARTESIAN_POINT('Ctrl Pts',(17.276743966429,-37.0175554714064,-1.19096704316446));
#6164=CARTESIAN_POINT('Ctrl Pts',(17.2598646740236,-37.0588230112599,-1.23155737439063));
#6165=CARTESIAN_POINT('Ctrl Pts',(17.2429794869056,-37.1001049628722,-1.27216188087575));
#6166=CARTESIAN_POINT('Ctrl Pts',(17.2246126805968,-37.1425264085214,-1.31137063355239));
#6167=CARTESIAN_POINT('Ctrl Pts',(17.2048486227575,-37.1858640987754,-1.34894683398816));
#6168=CARTESIAN_POINT('Ctrl Pts',(17.1850670233857,-37.2292402532715,-1.38655638507238));
#6169=CARTESIAN_POINT('Ctrl Pts',(17.1638859123471,-37.2735337151076,-1.42252990567058));
#6170=CARTESIAN_POINT('Ctrl Pts',(17.1414219230217,-37.3184981015473,-1.45666435205317));
#6171=CARTESIAN_POINT('Ctrl Pts',(17.1189750441068,-37.363428239435,-1.49077279885125));
#6172=CARTESIAN_POINT('Ctrl Pts',(17.0952475818025,-37.4090276429994,-1.52304454512938));
#6173=CARTESIAN_POINT('Ctrl Pts',(17.0703836278416,-37.4550370636491,-1.55331889475882));
#6174=CARTESIAN_POINT('Ctrl Pts',(17.0455338347552,-37.5010202803558,-1.58357600210788));
#6175=CARTESIAN_POINT('Ctrl Pts',(17.0195492678746,-37.5474123943199,-1.61183773325672));
#6176=CARTESIAN_POINT('Ctrl Pts',(16.9925957131083,-37.5939508986816,-1.63799064371655));
#6177=CARTESIAN_POINT('Ctrl Pts',(16.9866313689786,-37.6042490451674,-1.64377781944638));
#6178=CARTESIAN_POINT('Ctrl Pts',(16.9806196481277,-37.6145543671727,-1.64946192467123));
#6179=CARTESIAN_POINT('Ctrl Pts',(16.9745624584517,-37.6248640450332,-1.65504205590818));
#6180=CARTESIAN_POINT('Ctrl Pts',(16.9471867139075,-37.6714591035566,-1.68026171311492));
#6181=CARTESIAN_POINT('Ctrl Pts',(16.9188767468623,-37.7190418662623,-1.70359676647061));
#6182=CARTESIAN_POINT('Ctrl Pts',(16.8897687667342,-37.767369642264,-1.72487226661159));
#6183=CARTESIAN_POINT('Ctrl Pts',(16.8606506213001,-37.8157142956525,-1.74615519674153));
#6184=CARTESIAN_POINT('Ctrl Pts',(16.8307342255311,-37.8648038998849,-1.76537666733448));
#6185=CARTESIAN_POINT('Ctrl Pts',(16.8001770855338,-37.9143729790276,-1.78240346403856));
#6186=CARTESIAN_POINT('Ctrl Pts',(16.7695928246345,-37.9639860530644,-1.79944537282729));
#6187=CARTESIAN_POINT('Ctrl Pts',(16.7383670797762,-38.0140787869401,-1.81428839412874));
#6188=CARTESIAN_POINT('Ctrl Pts',(16.7066735508298,-38.0643718505644,-1.82684686809392));
#6189=CARTESIAN_POINT('Ctrl Pts',(16.6750041622648,-38.1146266068819,-1.83939577649913));
#6190=CARTESIAN_POINT('Ctrl Pts',(16.6428681509952,-38.1650806884555,-1.84966349840215));
#6191=CARTESIAN_POINT('Ctrl Pts',(16.6104481718161,-38.2154525822997,-1.857615636562));
#6192=CARTESIAN_POINT('Ctrl Pts',(16.5780466569275,-38.2657957876221,-1.86556324570632));
#6193=CARTESIAN_POINT('Ctrl Pts',(16.5453619571878,-38.3160562250962,-1.8711979799005));
#6194=CARTESIAN_POINT('Ctrl Pts',(16.5125789155394,-38.3659603852787,-1.87453687269548));
#6195=CARTESIAN_POINT('Ctrl Pts',(16.5053246092446,-38.3770032917678,-1.87527571051537));
#6196=CARTESIAN_POINT('Ctrl Pts',(16.4980654819446,-38.3880288042224,-1.8759023263398));
#6197=CARTESIAN_POINT('Ctrl Pts',(16.4908035184053,-38.3990340585972,-1.87641723476232));
#6198=CARTESIAN_POINT('Ctrl Pts',(16.4579827435291,-38.4487728068489,-1.87874438682333));
#6199=CARTESIAN_POINT('Ctrl Pts',(16.4250476365346,-38.4990258953495,-1.87880825693467));
#6200=CARTESIAN_POINT('Ctrl Pts',(16.3921796210864,-38.5495245287558,-1.87655505226089));
#6201=CARTESIAN_POINT('Ctrl Pts',(16.3593001272248,-38.6000407976712,-1.87430106070618));
#6202=CARTESIAN_POINT('Ctrl Pts',(16.3264882189097,-38.6508021268515,-1.86972820122937));
#6203=CARTESIAN_POINT('Ctrl Pts',(16.2939283755429,-38.7015274673234,-1.86283322829525));
#6204=CARTESIAN_POINT('Ctrl Pts',(16.2613396337801,-38.7522978289265,-1.85593213574759));
#6205=CARTESIAN_POINT('Ctrl Pts',(16.2290038633852,-38.8030314363447,-1.8467048153458));
#6206=CARTESIAN_POINT('Ctrl Pts',(16.1971020718583,-38.853444740426,-1.83519995710512));
#6207=CARTESIAN_POINT('Ctrl Pts',(16.1652245793432,-38.9038196456148,-1.82370386190477));
#6208=CARTESIAN_POINT('Ctrl Pts',(16.1337808348973,-38.9538740467511,-1.8099339111838));
#6209=CARTESIAN_POINT('Ctrl Pts',(16.1029407800788,-39.00333377084,-1.79398881938442));
#6210=CARTESIAN_POINT('Ctrl Pts',(16.072118289729,-39.0527653259201,-1.77805280886157));
#6211=CARTESIAN_POINT('Ctrl Pts',(16.0418991711874,-39.101602259426,-1.75994451788808));
#6212=CARTESIAN_POINT('Ctrl Pts',(16.0124364095012,-39.1495894550789,-1.73980808435094));
#6213=CARTESIAN_POINT('Ctrl Pts',(16.0059168223363,-39.1602081712804,-1.73535224836942));
#6214=CARTESIAN_POINT('Ctrl Pts',(15.9994341942539,-39.1707853717025,-1.7307972658445));
#6215=CARTESIAN_POINT('Ctrl Pts',(15.9929900464286,-39.1813184599546,-1.72614496752462));
#6216=CARTESIAN_POINT('Ctrl Pts',(15.963865426909,-39.2289232319161,-1.70511869343336));
#6217=CARTESIAN_POINT('Ctrl Pts',(15.9355074609204,-39.2765337068249,-1.68189873004132));
#6218=CARTESIAN_POINT('Ctrl Pts',(15.908092783664,-39.3238838539582,-1.65656309537201));
#6219=CARTESIAN_POINT('Ctrl Pts',(15.8806685324492,-39.3712505370635,-1.63121861280318));
#6220=CARTESIAN_POINT('Ctrl Pts',(15.8541886802725,-39.4183560519282,-1.60375713415806));
#6221=CARTESIAN_POINT('Ctrl Pts',(15.8288131722884,-39.4649335144336,-1.57430602553619));
#6222=CARTESIAN_POINT('Ctrl Pts',(15.8034151423452,-39.5115523166318,-1.54482877766759));
#6223=CARTESIAN_POINT('Ctrl Pts',(15.7791238088687,-39.5576414662295,-1.51335869953388));
#6224=CARTESIAN_POINT('Ctrl Pts',(15.7560762807607,-39.6029427589422,-1.48006918735986));
#6225=CARTESIAN_POINT('Ctrl Pts',(15.7330463075338,-39.6482095464881,-1.44680503119899));
#6226=CARTESIAN_POINT('Ctrl Pts',(15.7112585337647,-39.6926890703548,-1.41172471547191));
#6227=CARTESIAN_POINT('Ctrl Pts',(15.6908214294883,-39.7361426481477,-1.37504051469807));
#6228=CARTESIAN_POINT('Ctrl Pts',(15.6703959648435,-39.7795714776383,-1.33837720683433));
#6229=CARTESIAN_POINT('Ctrl Pts',(15.6513198029633,-39.8219750221162,-1.300112459804));
#6230=CARTESIAN_POINT('Ctrl Pts',(15.6336694659168,-39.8631423112235,-1.26048896755389));
#6231=CARTESIAN_POINT('Ctrl Pts',(15.6297637590422,-39.8722519029356,-1.25172099073466));
#6232=CARTESIAN_POINT('Ctrl Pts',(15.6259277406505,-39.8813010825401,-1.24288658001294));
#6233=CARTESIAN_POINT('Ctrl Pts',(15.6221620196843,-39.8902877803239,-1.23398851968989));
#6234=CARTESIAN_POINT('Ctrl Pts',(15.6051426723112,-39.9309035701529,-1.1937733309007));
#6235=CARTESIAN_POINT('Ctrl Pts',(15.5896575693722,-39.9710818941145,-1.15186853252947));
#6236=CARTESIAN_POINT('Ctrl Pts',(15.5758295033097,-40.0105878076174,-1.10846850103232));
#6237=CARTESIAN_POINT('Ctrl Pts',(15.5619966081066,-40.0501075176709,-1.06505331305163));
#6238=CARTESIAN_POINT('Ctrl Pts',(15.5498222393783,-40.088953757816,-1.0201422978767));
#6239=CARTESIAN_POINT('Ctrl Pts',(15.5393951597974,-40.1269007411589,-0.973968206823742));
#6240=CARTESIAN_POINT('Ctrl Pts',(15.528958825692,-40.1648814042379,-0.927753134088986));
#6241=CARTESIAN_POINT('Ctrl Pts',(15.520273092198,-40.201960656485,-0.880273333152562));
#6242=CARTESIAN_POINT('Ctrl Pts',(15.5133886580473,-40.2379301825509,-0.831792563199941));
#6243=CARTESIAN_POINT('Ctrl Pts',(15.5065094676442,-40.2738723112865,-0.78334872016332));
#6244=CARTESIAN_POINT('Ctrl Pts',(15.50142888499,-40.3087059338662,-0.733906126190651));
#6245=CARTESIAN_POINT('Ctrl Pts',(15.4981573254988,-40.3422489797573,-0.683748572306699));
#6246=CARTESIAN_POINT('Ctrl Pts',(15.494887629273,-40.375772921733,-0.633619584870454));
#6247=CARTESIAN_POINT('Ctrl Pts',(15.4934248002907,-40.4080074037208,-0.582777184218984));
#6248=CARTESIAN_POINT('Ctrl Pts',(15.4937394369914,-40.4388026103992,-0.531514551846304));
#6249=CARTESIAN_POINT('Ctrl Pts',(15.4938090605188,-40.4456170440328,-0.520171039531854));
#6250=CARTESIAN_POINT('Ctrl Pts',(15.4939655687831,-40.4523611372968,-0.50880696400498));
#6251=CARTESIAN_POINT('Ctrl Pts',(15.4942083905324,-40.4590335018639,-0.49742551165457));
#6252=CARTESIAN_POINT('Ctrl Pts',(15.4953058344853,-40.4891895573443,-0.445986519513396));
#6253=CARTESIAN_POINT('Ctrl Pts',(15.4984396882371,-40.5186182216488,-0.393696645408317));
#6254=CARTESIAN_POINT('Ctrl Pts',(15.5036405113949,-40.5471378008383,-0.340828125587056));
#6255=CARTESIAN_POINT('Ctrl Pts',(15.508843150823,-40.5756673398482,-0.287941142626714));
#6256=CARTESIAN_POINT('Ctrl Pts',(15.5161143164105,-40.6032866955214,-0.234475768275153));
#6257=CARTESIAN_POINT('Ctrl Pts',(15.5254390386774,-40.6298299707505,-0.180724039812537));
#6258=CARTESIAN_POINT('Ctrl Pts',(15.5347720370746,-40.6563968043871,-0.126924604158004));
#6259=CARTESIAN_POINT('Ctrl Pts',(15.5461621861609,-40.6818852404221,-0.0728390372964673));
#6260=CARTESIAN_POINT('Ctrl Pts',(15.5595483775206,-40.7061515153927,-0.018769220632637));
#6261=CARTESIAN_POINT('Ctrl Pts',(15.572924372863,-40.7303993071853,0.0352594120403899));
#6262=CARTESIAN_POINT('Ctrl Pts',(15.5882931376616,-40.7534264935081,0.0892715721474465));
#6263=CARTESIAN_POINT('Ctrl Pts',(15.6055498705326,-40.7751175242776,0.142968160451429));
#6264=CARTESIAN_POINT('Ctrl Pts',(15.6227967751024,-40.796796201261,0.196634166706726));
#6265=CARTESIAN_POINT('Ctrl Pts',(15.641929118661,-40.8171400548386,0.249984259989185));
#6266=CARTESIAN_POINT('Ctrl Pts',(15.6628030948396,-40.836065321335,0.302732839448093));
#6267=CARTESIAN_POINT('Ctrl Pts',(15.66742213594,-40.8402531475084,0.314405165526342));
#6268=CARTESIAN_POINT('Ctrl Pts',(15.6721263189559,-40.8443716395307,0.32604811133055));
#6269=CARTESIAN_POINT('Ctrl Pts',(15.676913858231,-40.8484201102111,0.337658719487509));
#6270=CARTESIAN_POINT('Ctrl Pts',(15.6985513599794,-40.8667173577936,0.39013339172803));
#6271=CARTESIAN_POINT('Ctrl Pts',(15.722362551344,-40.8842079556607,0.442451690705955));
#6272=CARTESIAN_POINT('Ctrl Pts',(15.748265636864,-40.9007750781021,0.494317440109603));
#6273=CARTESIAN_POINT('Ctrl Pts',(15.7741777684528,-40.9173479862377,0.546201302457251));
#6274=CARTESIAN_POINT('Ctrl Pts',(15.8021830926676,-40.9329964698455,0.59763156288463));
#6275=CARTESIAN_POINT('Ctrl Pts',(15.83215090363,-40.9476214522587,0.648314739712493));
#6276=CARTESIAN_POINT('Ctrl Pts',(15.8621453124374,-40.9622594150332,0.699042900249139));
#6277=CARTESIAN_POINT('Ctrl Pts',(15.894105351942,-40.9758718192981,0.749021923203392));
#6278=CARTESIAN_POINT('Ctrl Pts',(15.9278548543797,-40.9883813311363,0.797971596265911));
#6279=CARTESIAN_POINT('Ctrl Pts',(15.9615786504381,-41.000881314708,0.846883985257014));
#6280=CARTESIAN_POINT('Ctrl Pts',(15.9970886749691,-41.0122799393024,0.894767940773897));
#6281=CARTESIAN_POINT('Ctrl Pts',(16.0341705677136,-41.022524908682,0.941368295639198));
#6282=CARTESIAN_POINT('Ctrl Pts',(16.0712313410483,-41.0327640432001,0.98794211000402));
#6283=CARTESIAN_POINT('Ctrl Pts',(16.1098615702851,-41.0418507872325,1.03323325564664));
#6284=CARTESIAN_POINT('Ctrl Pts',(16.1498172223449,-41.0497592430222,1.07702027911083));
#6285=CARTESIAN_POINT('Ctrl Pts',(16.1586587002461,-41.0515092441733,1.08670957162287));
#6286=CARTESIAN_POINT('Ctrl Pts',(16.1675649833532,-41.0532016525781,1.09632535949797));
#6287=CARTESIAN_POINT('Ctrl Pts',(16.1765332779228,-41.0548363630651,1.10586550012264));
#6288=CARTESIAN_POINT('Ctrl Pts',(16.2170658935834,-41.0622245115445,1.14898260006709));
#6289=CARTESIAN_POINT('Ctrl Pts',(16.2595174031787,-41.0689531166638,1.1909670431649));
#6290=CARTESIAN_POINT('Ctrl Pts',(16.3036957872465,-41.0749689905696,1.23155737439127));
#6291=CARTESIAN_POINT('Ctrl Pts',(16.3478895996191,-41.0809869653838,1.27216188087589));
#6292=CARTESIAN_POINT('Ctrl Pts',(16.3938110523704,-41.0862915673586,1.31137063355205));
#6293=CARTESIAN_POINT('Ctrl Pts',(16.4412246219907,-41.0908442363149,1.3489468339874));
#6294=CARTESIAN_POINT('Ctrl Pts',(16.4886802733888,-41.0954009459794,1.38655638507171));
#6295=CARTESIAN_POINT('Ctrl Pts',(16.5376300920798,-41.0992042966577,1.42252990566999));
#6296=CARTESIAN_POINT('Ctrl Pts',(16.5878023876649,-41.1022321044514,1.45666435205266));
#6297=CARTESIAN_POINT('Ctrl Pts',(16.6379364679291,-41.1052576060193,1.49077279885112));
#6298=CARTESIAN_POINT('Ctrl Pts',(16.6892904409661,-41.1075087226786,1.52304454512959));
#6299=CARTESIAN_POINT('Ctrl Pts',(16.7415677450431,-41.1089806172348,1.55331889475933));
#6300=CARTESIAN_POINT('Ctrl Pts',(16.7938152754033,-41.1104516734967,1.58357600210906));
#6301=CARTESIAN_POINT('Ctrl Pts',(16.846984308073,-41.1111444354538,1.61183773325848));
#6302=CARTESIAN_POINT('Ctrl Pts',(16.9007646124888,-41.1110712244847,1.63799064371879));
#6303=CARTESIAN_POINT('Ctrl Pts',(16.9126652410207,-41.1110550241943,1.64377781944784));
#6304=CARTESIAN_POINT('Ctrl Pts',(16.9245957720954,-41.1110013822196,1.64946192467195));
#6305=CARTESIAN_POINT('Ctrl Pts',(16.9365528098639,-41.1109105410149,1.65504205590818));
#6306=CARTESIAN_POINT('Ctrl Pts',(16.9905931865084,-41.1104999800539,1.68026171311506));
#6307=CARTESIAN_POINT('Ctrl Pts',(17.0459560513166,-41.1097742107652,1.70359676647086));
#6308=CARTESIAN_POINT('Ctrl Pts',(17.1023631231069,-41.1087298485223,1.72487226661194));
#6309=CARTESIAN_POINT('Ctrl Pts',(17.1587898937959,-41.1076851215595,1.746155196742));
#6310=CARTESIAN_POINT('Ctrl Pts',(17.2162609360078,-41.1063215649501,1.76537666733503));
#6311=CARTESIAN_POINT('Ctrl Pts',(17.2744675877866,-41.1046428450168,1.78240346403918));
#6312=CARTESIAN_POINT('Ctrl Pts',(17.332725900712,-41.1029626351404,1.79944537282785));
#6313=CARTESIAN_POINT('Ctrl Pts',(17.3917203532226,-41.1009667137788,1.81428839412925));
#6314=CARTESIAN_POINT('Ctrl Pts',(17.4511221884286,-41.0986658443878,1.82684686809438));
#6315=CARTESIAN_POINT('Ctrl Pts',(17.5104787783426,-41.096366727527,1.83939577649946));
#6316=CARTESIAN_POINT('Ctrl Pts',(17.5702413003446,-41.0937631661781,1.84966349840239));
#6317=CARTESIAN_POINT('Ctrl Pts',(17.6300746296397,-41.0908725875409,1.85761563656216));
#6318=CARTESIAN_POINT('Ctrl Pts',(17.6898738818011,-41.0879836551874,1.86556324570646));
#6319=CARTESIAN_POINT('Ctrl Pts',(17.7497430473289,-41.0848080936348,1.87119797990062));
#6320=CARTESIAN_POINT('Ctrl Pts',(17.8093528386257,-41.0813692268452,1.87453687269556));
#6321=CARTESIAN_POINT('Ctrl Pts',(17.8225434293238,-41.0806082665516,1.87527571051541));
#6322=CARTESIAN_POINT('Ctrl Pts',(17.8357213668488,-41.0798344341278,1.87590232633982));
#6323=CARTESIAN_POINT('Ctrl Pts',(17.8488831784817,-41.0790480164089,1.87641723476232));
#6324=CARTESIAN_POINT('Ctrl Pts',(17.9083685854582,-41.0754937657201,1.87874438682333));
#6325=CARTESIAN_POINT('Ctrl Pts',(17.9683565902155,-41.0720976706368,1.87880825693467));
#6326=CARTESIAN_POINT('Ctrl Pts',(18.028523697326,-41.0688824509898,1.87655505226089));
#6327=CARTESIAN_POINT('Ctrl Pts',(18.0887118164424,-41.0656661084998,1.87430106070616));
#6328=CARTESIAN_POINT('Ctrl Pts',(18.1490783712004,-41.0626308269423,1.86972820122929));
#6329=CARTESIAN_POINT('Ctrl Pts',(18.2092877263486,-41.0597958456794,1.86283322829508));
#6330=CARTESIAN_POINT('Ctrl Pts',(18.2695505201376,-41.056958348237,1.85593213574738));
#6331=CARTESIAN_POINT('Ctrl Pts',(18.3296549981847,-41.0543215533332,1.84670481534557));
#6332=CARTESIAN_POINT('Ctrl Pts',(18.3892650959712,-41.0519004434854,1.83519995710487));
#6333=CARTESIAN_POINT('Ctrl Pts',(18.4488297898368,-41.0494811777526,1.82370386190423));
#6334=CARTESIAN_POINT('Ctrl Pts',(18.5079000450163,-41.0472772968405,1.80993391118287));
#6335=CARTESIAN_POINT('Ctrl Pts',(18.566153449952,-41.045298887958,1.793988819383));
#6336=CARTESIAN_POINT('Ctrl Pts',(18.6243736775742,-41.0433216058472,1.77805280886017));
#6337=CARTESIAN_POINT('Ctrl Pts',(18.6817772619035,-41.0415695482632,1.75994451788674));
#6338=CARTESIAN_POINT('Ctrl Pts',(18.7380667732378,-41.0400476460038,1.73980808434969));
#6339=CARTESIAN_POINT('Ctrl Pts',(18.7505226448052,-41.0397108759976,1.73535224836857));
#6340=CARTESIAN_POINT('Ctrl Pts',(18.7629240831117,-41.039385355606,1.73079726584407));
#6341=CARTESIAN_POINT('Ctrl Pts',(18.7752680790298,-41.0390711040097,1.72614496752461));
#6342=CARTESIAN_POINT('Ctrl Pts',(18.8310573306497,-41.0376508296109,1.70511869343333));
#6343=CARTESIAN_POINT('Ctrl Pts',(18.8864681944013,-41.0368973481195,1.68189873004126));
#6344=CARTESIAN_POINT('Ctrl Pts',(18.94118196332,-41.0368306147455,1.65656309537192));
#6345=CARTESIAN_POINT('Ctrl Pts',(18.9959148397898,-41.0367638580664,1.63121861280294));
#6346=CARTESIAN_POINT('Ctrl Pts',(19.0499493384097,-41.0373843908253,1.60375713415765));
#6347=CARTESIAN_POINT('Ctrl Pts',(19.1029743581755,-41.0386972875298,1.57430602553558));
#6348=CARTESIAN_POINT('Ctrl Pts',(19.1560464401448,-41.040011349492,1.54482877766693));
#6349=CARTESIAN_POINT('Ctrl Pts',(19.2081064812735,-41.0420190124084,1.51335869953315));
#6350=CARTESIAN_POINT('Ctrl Pts',(19.2588623156411,-41.0447099139289,1.48006918735906));
#6351=CARTESIAN_POINT('Ctrl Pts',(19.3095794902174,-41.0473987658389,1.44680503119789));
#6352=CARTESIAN_POINT('Ctrl Pts',(19.3589937747191,-41.0507697621964,1.41172471547047));
#6353=CARTESIAN_POINT('Ctrl Pts',(19.4068442291116,-41.0547974996097,1.37504051469626));
#6354=CARTESIAN_POINT('Ctrl Pts',(19.4546674310289,-41.0588229430885,1.33837720683284));
#6355=CARTESIAN_POINT('Ctrl Pts',(19.5009280586969,-41.0635042745324,1.30011245980285));
#6356=CARTESIAN_POINT('Ctrl Pts',(19.5454051453916,-41.0688022788184,1.26048896755312));
#6357=CARTESIAN_POINT('Ctrl Pts',(19.5552471366694,-41.0699746333013,1.25172099073414));
#6358=CARTESIAN_POINT('Ctrl Pts',(19.5650019652858,-41.0711771337269,1.24288658001268));
#6359=CARTESIAN_POINT('Ctrl Pts',(19.5746675343455,-41.0724092725985,1.2339885196899));
#6360=CARTESIAN_POINT('Ctrl Pts',(19.6183515138191,-41.0779779803321,1.1937733309004));
#6361=CARTESIAN_POINT('Ctrl Pts',(19.6608895145212,-41.0846566497875,1.15186853252883));
#6362=CARTESIAN_POINT('Ctrl Pts',(19.702016672246,-41.0924341500438,1.10846850103133));
#6363=CARTESIAN_POINT('Ctrl Pts',(19.7431581927032,-41.1002143664166,1.06505331305146));
#6364=CARTESIAN_POINT('Ctrl Pts',(19.7828872078737,-41.1090941738953,1.0201422978774));
#6365=CARTESIAN_POINT('Ctrl Pts',(19.8209637992355,-41.1190375497622,0.973968206825355));
#6366=CARTESIAN_POINT('Ctrl Pts',(19.8590741853671,-41.1289897508439,0.927753134090774));
#6367=CARTESIAN_POINT('Ctrl Pts',(19.8955286265134,-41.1400073111111,0.880273333154538));
#6368=CARTESIAN_POINT('Ctrl Pts',(19.9301213669238,-41.1520299792788,0.831792563202099));
#6369=CARTESIAN_POINT('Ctrl Pts',(19.964687758676,-41.1640434899999,0.783348720166139));
#6370=CARTESIAN_POINT('Ctrl Pts',(19.9973948520627,-41.177060387645,0.73390612619414));
#6371=CARTESIAN_POINT('Ctrl Pts',(20.02807976167,-41.1909986569609,0.683748572310881));
#6372=CARTESIAN_POINT('Ctrl Pts',(20.0587471951687,-41.2049289879544,0.63361958487495));
#6373=CARTESIAN_POINT('Ctrl Pts',(20.0873944899392,-41.2197793818882,0.582777184223805));
#6374=CARTESIAN_POINT('Ctrl Pts',(20.1139066028871,-41.235449468603,0.531514551851436));
#6375=CARTESIAN_POINT('Ctrl Pts',(20.1197732637633,-41.2389169811637,0.520171039535283));
#6376=CARTESIAN_POINT('Ctrl Pts',(20.1255355657243,-41.242424567929,0.508806964006691));
#6377=CARTESIAN_POINT('Ctrl Pts',(20.1311925920688,-41.2459710400166,0.497425511654565));
#6378=CARTESIAN_POINT('Ctrl Pts',(20.1567597802162,-41.2619994820991,0.445986519513783));
#6379=CARTESIAN_POINT('Ctrl Pts',(20.1806788242272,-41.279427811212,0.393696645409107));
#6380=CARTESIAN_POINT('Ctrl Pts',(20.2027770927316,-41.2981916457819,0.340828125588261));
#6381=CARTESIAN_POINT('Ctrl Pts',(20.2248830785584,-41.3169620331983,0.287941142627905));
#6382=CARTESIAN_POINT('Ctrl Pts',(20.2451665594138,-41.3370687251488,0.234475768276321));
#6383=CARTESIAN_POINT('Ctrl Pts',(20.2634913489284,-41.3584158091296,0.180724039813684));
#6384=CARTESIAN_POINT('Ctrl Pts',(20.2818324025573,-41.3797818396534,0.126924604159152));
#6385=CARTESIAN_POINT('Ctrl Pts',(20.2982109611232,-41.4023902161325,0.0728390372976226));
#6386=CARTESIAN_POINT('Ctrl Pts',(20.3125330760231,-41.4261161353952,0.0187692206337898));
#6387=CARTESIAN_POINT('Ctrl Pts',(20.3268442820301,-41.4498239830589,-0.0352594120392662));
#6388=CARTESIAN_POINT('Ctrl Pts',(20.339102027964,-41.4746473169607,-0.0892715721463639));
#6389=CARTESIAN_POINT('Ctrl Pts',(20.3492586452092,-41.5004376013981,-0.142968160450382));
#6390=CARTESIAN_POINT('Ctrl Pts',(20.3594094779124,-41.5262131973838,-0.196634166705389));
#6391=CARTESIAN_POINT('Ctrl Pts',(20.3674616001421,-41.552954219728,-0.24998425998755));
#6392=CARTESIAN_POINT('Ctrl Pts',(20.3734143736121,-41.5804942466247,-0.302732839446182));
#6393=CARTESIAN_POINT('Ctrl Pts',(20.3747316169147,-41.5865883666458,-0.314405165525066));
#6394=CARTESIAN_POINT('Ctrl Pts',(20.3759462441234,-41.5927215546531,-0.326048111329918));
#6395=CARTESIAN_POINT('Ctrl Pts',(20.3770585529417,-41.5988919206274,-0.337658719487506));
#6396=CARTESIAN_POINT('Ctrl Pts',(20.3820856832934,-41.6267791706076,-0.39013339172863));
#6397=CARTESIAN_POINT('Ctrl Pts',(20.3853273896913,-41.6561455661577,-0.442451690707166));
#6398=CARTESIAN_POINT('Ctrl Pts',(20.3867233958332,-41.6868618574755,-0.494317440111406));
#6399=CARTESIAN_POINT('Ctrl Pts',(20.3881198894988,-41.7175888757661,-0.546201302460337));
#6400=CARTESIAN_POINT('Ctrl Pts',(20.3876692117263,-41.7496664397822,-0.597631562888963));
#6401=CARTESIAN_POINT('Ctrl Pts',(20.3853509125446,-41.7829318165789,-0.648314739718037));
#6402=CARTESIAN_POINT('Ctrl Pts',(20.3830305557632,-41.816226717965,-0.699042900254785));
#6403=CARTESIAN_POINT('Ctrl Pts',(20.3788392239107,-41.8507111262147,-0.749021923209121));
#6404=CARTESIAN_POINT('Ctrl Pts',(20.3727980277325,-41.8861938086101,-0.797971596271709));
#6405=CARTESIAN_POINT('Ctrl Pts',(20.3667614330232,-41.9216494644944,-0.846883985262495));
#6406=CARTESIAN_POINT('Ctrl Pts',(20.3588779192245,-41.9581013601243,-0.894767940779068));
#6407=CARTESIAN_POINT('Ctrl Pts',(20.3492093765959,-41.9953377059512,-0.941368295644055));
#6408=CARTESIAN_POINT('Ctrl Pts',(20.3395463405339,-42.0325528444024,-0.987942110009238));
#6409=CARTESIAN_POINT('Ctrl Pts',(20.3281005770849,-42.0705509762921,-1.03323325565219));
#6410=CARTESIAN_POINT('Ctrl Pts',(20.3149716746733,-42.1091078138959,-1.07702027911667));
#6411=CARTESIAN_POINT('Ctrl Pts',(20.3120664811768,-42.1176397589392,-1.08670957162673));
#6412=CARTESIAN_POINT('Ctrl Pts',(20.3090790082959,-42.1261990305639,-1.09632535949989));
#6413=CARTESIAN_POINT('Ctrl Pts',(20.3060105618213,-42.1347831567316,-1.10586550012264));
#6414=CARTESIAN_POINT('Ctrl Pts',(20.2921425782615,-42.1735795058142,-1.148982600066));
#6415=CARTESIAN_POINT('Ctrl Pts',(20.2767439664296,-42.2137078941114,-1.19096704316276));
#6416=CARTESIAN_POINT('Ctrl Pts',(20.2598646740246,-42.254975433964,-1.23155737438818));
#6417=CARTESIAN_POINT('Ctrl Pts',(20.2429794869067,-42.296257385576,-1.27216188087308));
#6418=CARTESIAN_POINT('Ctrl Pts',(20.2246126805982,-42.3386788312249,-1.31137063354952));
#6419=CARTESIAN_POINT('Ctrl Pts',(20.2048486227591,-42.3820165214785,-1.34894683398513));
#6420=CARTESIAN_POINT('Ctrl Pts',(20.1850670233874,-42.4253926759745,-1.38655638506932));
#6421=CARTESIAN_POINT('Ctrl Pts',(20.1638859123489,-42.4696861378104,-1.42252990566751));
#6422=CARTESIAN_POINT('Ctrl Pts',(20.1414219230237,-42.5146505242499,-1.45666435205011));
#6423=CARTESIAN_POINT('Ctrl Pts',(20.1189750441085,-42.5595806621383,-1.49077279884886));
#6424=CARTESIAN_POINT('Ctrl Pts',(20.0952475818038,-42.6051800657034,-1.5230445451276));
#6425=CARTESIAN_POINT('Ctrl Pts',(20.0703836278425,-42.6511894863539,-1.5533188947576));
#6426=CARTESIAN_POINT('Ctrl Pts',(20.0455338347557,-42.6971727030616,-1.58357600210732));
#6427=CARTESIAN_POINT('Ctrl Pts',(20.0195492678746,-42.7435648170265,-1.61183773325675));
#6428=CARTESIAN_POINT('Ctrl Pts',(19.9925957131078,-42.7901033213892,-1.63799064371707));
#6429=CARTESIAN_POINT('Ctrl Pts',(19.9866313689782,-42.8004014678746,-1.64377781944672));
#6430=CARTESIAN_POINT('Ctrl Pts',(19.9806196481275,-42.8107067898797,-1.6494619246714));
#6431=CARTESIAN_POINT('Ctrl Pts',(19.9745624584516,-42.8210164677399,-1.65504205590818));
#6432=CARTESIAN_POINT('Ctrl Pts',(19.9471867139073,-42.8676115262635,-1.68026171311505));
#6433=CARTESIAN_POINT('Ctrl Pts',(19.9188767468619,-42.9151942889694,-1.70359676647086));
#6434=CARTESIAN_POINT('Ctrl Pts',(19.8897687667337,-42.9635220649715,-1.72487226661194));
#6435=CARTESIAN_POINT('Ctrl Pts',(19.8606506212993,-43.0118667183605,-1.7461551967421));
#6436=CARTESIAN_POINT('Ctrl Pts',(19.8307342255299,-43.0609563225936,-1.76537666733522));
#6437=CARTESIAN_POINT('Ctrl Pts',(19.8001770855323,-43.1105254017368,-1.78240346403943));
#6438=CARTESIAN_POINT('Ctrl Pts',(19.7695928246328,-43.1601384757738,-1.79944537282815));
#6439=CARTESIAN_POINT('Ctrl Pts',(19.7383670797743,-43.2102312096498,-1.81428839412959));
#6440=CARTESIAN_POINT('Ctrl Pts',(19.7066735508277,-43.2605242732743,-1.82684686809472));
#6441=CARTESIAN_POINT('Ctrl Pts',(19.6750041622631,-43.3107790295912,-1.83939577649969));
#6442=CARTESIAN_POINT('Ctrl Pts',(19.6428681509939,-43.3612331111643,-1.84966349840252));
#6443=CARTESIAN_POINT('Ctrl Pts',(19.6104481718151,-43.4116050050079,-1.85761563656223));
#6444=CARTESIAN_POINT('Ctrl Pts',(19.5780466569263,-43.4619482103305,-1.86556324570655));
#6445=CARTESIAN_POINT('Ctrl Pts',(19.5453619571864,-43.5122086478048,-1.87119797990071));
#6446=CARTESIAN_POINT('Ctrl Pts',(19.5125789155379,-43.5621128079876,-1.87453687269564));
#6447=CARTESIAN_POINT('Ctrl Pts',(19.5053246092435,-43.573155714476,-1.87527571051545));
#6448=CARTESIAN_POINT('Ctrl Pts',(19.498065481944,-43.5841812269298,-1.87590232633983));
#6449=CARTESIAN_POINT('Ctrl Pts',(19.4908035184053,-43.5951864813039,-1.87641723476232));
#6450=CARTESIAN_POINT('Ctrl Pts',(19.4579827435292,-43.6449252295553,-1.87874438682332));
#6451=CARTESIAN_POINT('Ctrl Pts',(19.4250476365349,-43.6951783180556,-1.87880825693467));
#6452=CARTESIAN_POINT('Ctrl Pts',(19.3921796210868,-43.7456769514617,-1.87655505226092));
#6453=CARTESIAN_POINT('Ctrl Pts',(19.3593001272252,-43.7961932203771,-1.87430106070623));
#6454=CARTESIAN_POINT('Ctrl Pts',(19.3264882189101,-43.8469545495574,-1.86972820122944));
#6455=CARTESIAN_POINT('Ctrl Pts',(19.2939283755433,-43.8976798900294,-1.86283322829534));
#6456=CARTESIAN_POINT('Ctrl Pts',(19.2613396337806,-43.9484502516322,-1.85593213574773));
#6457=CARTESIAN_POINT('Ctrl Pts',(19.2290038633859,-43.9991838590501,-1.84670481534603));
#6458=CARTESIAN_POINT('Ctrl Pts',(19.1971020718592,-44.0495971631312,-1.83519995710545));
#6459=CARTESIAN_POINT('Ctrl Pts',(19.165224579344,-44.0999720683201,-1.8237038619051));
#6460=CARTESIAN_POINT('Ctrl Pts',(19.1337808348979,-44.1500264694566,-1.80993391118412));
#6461=CARTESIAN_POINT('Ctrl Pts',(19.1029407800793,-44.1994861935458,-1.79398881938471));
#6462=CARTESIAN_POINT('Ctrl Pts',(19.0721182897293,-44.2489177486262,-1.77805280886179));
#6463=CARTESIAN_POINT('Ctrl Pts',(19.0418991711875,-44.2977546821324,-1.7599445178882));
#6464=CARTESIAN_POINT('Ctrl Pts',(19.0124364095012,-44.3457418777856,-1.73980808435093));
#6465=CARTESIAN_POINT('Ctrl Pts',(19.0059168223362,-44.3563605939871,-1.73535224836942));
#6466=CARTESIAN_POINT('Ctrl Pts',(18.9994341942538,-44.3669377944092,-1.7307972658445));
#6467=CARTESIAN_POINT('Ctrl Pts',(18.9929900464286,-44.3774708826612,-1.72614496752462));
#6468=CARTESIAN_POINT('Ctrl Pts',(18.9638689474167,-44.4250699002826,-1.70512123503431));
#6469=CARTESIAN_POINT('Ctrl Pts',(18.9355143751871,-44.4726744936063,-1.6819044064235));
#6470=CARTESIAN_POINT('Ctrl Pts',(18.9081029063368,-44.5200187400556,-1.65657248784969));
#6471=CARTESIAN_POINT('Ctrl Pts',(18.8806675607685,-44.5674042256384,-1.63121850394697));
#6472=CARTESIAN_POINT('Ctrl Pts',(18.8541774156252,-44.6145282512141,-1.60374589296114));
#6473=CARTESIAN_POINT('Ctrl Pts',(18.8287926096657,-44.6611236299078,-1.57428219817154));
#6474=CARTESIAN_POINT('Ctrl Pts',(18.8184986722539,-44.6800187876141,-1.56233420729198));
#6475=CARTESIAN_POINT('Ctrl Pts',(18.8083862688025,-44.6988270623412,-1.55005934730935));
#6476=CARTESIAN_POINT('Ctrl Pts',(18.7984650370909,-44.7175309941718,-1.53746830583367));
#6477=CARTESIAN_POINT('Origin',(18.8566790438274,-45.0585105479845,-1.8991695164178));
#6478=CARTESIAN_POINT('Ctrl Pts',(3.23546955922299,-20.8337067011995,-0.275782109461828));
#6479=CARTESIAN_POINT('Ctrl Pts',(3.24186862921633,-20.8593806772798,-0.20661167837916));
#6480=CARTESIAN_POINT('Ctrl Pts',(3.25061275091574,-20.8836022411874,-0.13722900415027));
#6481=CARTESIAN_POINT('Ctrl Pts',(3.26163446655099,-20.9062743501088,-0.0679614783569666));
#6482=CARTESIAN_POINT('Ctrl Pts',(3.27267218983593,-20.9289793874045,0.00140664976769637));
#6483=CARTESIAN_POINT('Ctrl Pts',(3.2859938790503,-20.9501303415672,0.0706586286035451));
#6484=CARTESIAN_POINT('Ctrl Pts',(3.30149075533669,-20.9696606976443,0.139474749410477));
#6485=CARTESIAN_POINT('Ctrl Pts',(3.30349716107535,-20.9721893245615,0.148384484323984));
#6486=CARTESIAN_POINT('Ctrl Pts',(3.30553997633814,-20.9746908292539,0.157286933483624));
#6487=CARTESIAN_POINT('Ctrl Pts',(3.30761891872921,-20.9771651064803,0.166181422977341));
#6488=CARTESIAN_POINT('Ctrl Pts',(3.32367525640493,-20.9962747416586,0.234876412977235));
#6489=CARTESIAN_POINT('Ctrl Pts',(3.34225287296391,-21.0143094751689,0.303705335324898));
#6490=CARTESIAN_POINT('Ctrl Pts',(3.36331943904694,-21.0311598985507,0.372344470076959));
#6491=CARTESIAN_POINT('Ctrl Pts',(3.38435814667915,-21.0479880389137,0.440892836359587));
#6492=CARTESIAN_POINT('Ctrl Pts',(3.40787918918959,-21.0636347575442,0.509251242356875));
#6493=CARTESIAN_POINT('Ctrl Pts',(3.43380253213101,-21.078010950724,0.577093346534907));
#6494=CARTESIAN_POINT('Ctrl Pts',(3.45972752251918,-21.0923880575211,0.644939762126552));
#6495=CARTESIAN_POINT('Ctrl Pts',(3.48805494275311,-21.1054942936163,0.712269124557974));
#6496=CARTESIAN_POINT('Ctrl Pts',(3.51865844890996,-21.1172636372539,0.778761359262223));
#6497=CARTESIAN_POINT('Ctrl Pts',(3.54925455115654,-21.1290301335326,0.845237507491391));
#6498=CARTESIAN_POINT('Ctrl Pts',(3.58212531838659,-21.1394602771986,0.910876280137527));
#6499=CARTESIAN_POINT('Ctrl Pts',(3.61710196385512,-21.1485133692941,0.975374241033912));
#6500=CARTESIAN_POINT('Ctrl Pts',(3.65213177087612,-21.1575802213264,1.03997023339348));
#6501=CARTESIAN_POINT('Ctrl Pts',(3.68927343113846,-21.1652658000617,1.10342135481118));
#6502=CARTESIAN_POINT('Ctrl Pts',(3.7283203630776,-21.1715556385076,1.16544861040201));
#6503=CARTESIAN_POINT('Ctrl Pts',(3.75451366980928,-21.1757749627804,1.20705748594561));
#6504=CARTESIAN_POINT('Ctrl Pts',(3.78156357052937,-21.179366767248,1.24802618569455));
#6505=CARTESIAN_POINT('Ctrl Pts',(3.80940000840298,-21.1823333185883,1.28827884419633));
#6506=CARTESIAN_POINT('Ctrl Pts',(3.85089568313003,-21.186755545672,1.3482833329773));
#6507=CARTESIAN_POINT('Ctrl Pts',(3.89472960492292,-21.1902085445568,1.4072279179729));
#6508=CARTESIAN_POINT('Ctrl Pts',(3.94074551483351,-21.1926544575637,1.46480935021334));
#6509=CARTESIAN_POINT('Ctrl Pts',(3.98670057325282,-21.1950971360925,1.52231463670269));
#6510=CARTESIAN_POINT('Ctrl Pts',(4.03483155540641,-21.1965352994454,1.57845972694472));
#6511=CARTESIAN_POINT('Ctrl Pts',(4.08493792610339,-21.1969494150408,1.63296134034075));
#6512=CARTESIAN_POINT('Ctrl Pts',(4.13504748109556,-21.1973635569535,1.68746641735274));
#6513=CARTESIAN_POINT('Ctrl Pts',(4.18713224730921,-21.1967534829521,1.74032721705632));
#6514=CARTESIAN_POINT('Ctrl Pts',(4.24095216427237,-21.195118825561,1.79128851362552));
#6515=CARTESIAN_POINT('Ctrl Pts',(4.29475906057596,-21.1934845636428,1.84223748112157));
#6516=CARTESIAN_POINT('Ctrl Pts',(4.35029972224413,-21.1908262376525,1.89128737321195));
#6517=CARTESIAN_POINT('Ctrl Pts',(4.40730213618998,-21.1871627463886,1.9382193964011));
#6518=CARTESIAN_POINT('Ctrl Pts',(4.46439118899948,-21.1834936869267,1.98522275230891));
#6519=CARTESIAN_POINT('Ctrl Pts',(4.52294581901202,-21.1788164818126,2.03010142110727));
#6520=CARTESIAN_POINT('Ctrl Pts',(4.58266933425896,-21.1731686893198,2.07267852251363));
#6521=CARTESIAN_POINT('Ctrl Pts',(4.62273282391777,-21.1693800597458,2.10123992340978));
#6522=CARTESIAN_POINT('Ctrl Pts',(4.66332182748729,-21.1651550595386,2.12876654161616));
#6523=CARTESIAN_POINT('Ctrl Pts',(4.70434308191444,-21.1605093534924,2.15521684061908));
#6524=CARTESIAN_POINT('Ctrl Pts',(4.76549331379183,-21.1535840167146,2.19464620327124));
#6525=CARTESIAN_POINT('Ctrl Pts',(4.82836829765705,-21.1460436532863,2.23203175294848));
#6526=CARTESIAN_POINT('Ctrl Pts',(4.89270780991765,-21.1379104295439,2.26715077383212));
#6527=CARTESIAN_POINT('Ctrl Pts',(4.95696223953439,-21.1297879611859,2.30222335328279));
#6528=CARTESIAN_POINT('Ctrl Pts',(5.02267680474199,-21.1210742381291,2.33503490407264));
#6529=CARTESIAN_POINT('Ctrl Pts',(5.08955858326424,-21.1118030675008,2.36540131373504));
#6530=CARTESIAN_POINT('Ctrl Pts',(5.15644461217079,-21.102531307683,2.39576965320423));
#6531=CARTESIAN_POINT('Ctrl Pts',(5.2244973822523,-21.0927021023501,2.42369216050349));
#6532=CARTESIAN_POINT('Ctrl Pts',(5.29339874516216,-21.0823601680819,2.44902900915281));
#6533=CARTESIAN_POINT('Ctrl Pts',(5.36228343875623,-21.0720207358393,2.47435972805499));
#6534=CARTESIAN_POINT('Ctrl Pts',(5.43201562568106,-21.0611689289218,2.49710580690362));
#6535=CARTESIAN_POINT('Ctrl Pts',(5.50226209398045,-21.0498589793117,2.51717642960937));
#6536=CARTESIAN_POINT('Ctrl Pts',(5.57261533098965,-21.0385318395316,2.53727755796962));
#6537=CARTESIAN_POINT('Ctrl Pts',(5.6434837004336,-21.026745293642,2.55469500339243));
#6538=CARTESIAN_POINT('Ctrl Pts',(5.71452769367997,-21.0145616201289,2.56938903350696));
#6539=CARTESIAN_POINT('Ctrl Pts',(5.76218514111884,-21.0063886169864,2.57924602402578));
#6540=CARTESIAN_POINT('Ctrl Pts',(5.80992153437209,-20.9980370694213,2.5878785763622));
#6541=CARTESIAN_POINT('Ctrl Pts',(5.85763560155421,-20.9895272661294,2.59528770975726));
#6542=CARTESIAN_POINT('Ctrl Pts',(5.92876278458999,-20.9768417339146,2.60633247743794));
#6543=CARTESIAN_POINT('Ctrl Pts',(6.00069227149917,-20.9640737507165,2.61475432517954));
#6544=CARTESIAN_POINT('Ctrl Pts',(6.07310043046255,-20.9512820916283,2.62045518191383));
#6545=CARTESIAN_POINT('Ctrl Pts',(6.14541283679449,-20.9385073482445,2.62614849982872));
#6546=CARTESIAN_POINT('Ctrl Pts',(6.21820198419475,-20.9257091132545,2.6291277811253));
#6547=CARTESIAN_POINT('Ctrl Pts',(6.29112897535549,-20.912947737482,2.62934454720093));
#6548=CARTESIAN_POINT('Ctrl Pts',(6.36406060107808,-20.900185550715,2.6295613270522));
#6549=CARTESIAN_POINT('Ctrl Pts',(6.43712937391484,-20.8874603548411,2.62701514692945));
#6550=CARTESIAN_POINT('Ctrl Pts',(6.50999015258026,-20.8748324508206,2.62170927404782));
#6551=CARTESIAN_POINT('Ctrl Pts',(6.58283330402795,-20.8622076018706,2.61640468481672));
#6552=CARTESIAN_POINT('Ctrl Pts',(6.65546784140341,-20.8496801221392,2.60834181054528));
#6553=CARTESIAN_POINT('Ctrl Pts',(6.72755350254027,-20.8373083140492,2.59757579979075));
#6554=CARTESIAN_POINT('Ctrl Pts',(6.79974872780499,-20.824917701854,2.58679342560749));
#6555=CARTESIAN_POINT('Ctrl Pts',(6.87139271924896,-20.8126833503939,2.57329990897777));
#6556=CARTESIAN_POINT('Ctrl Pts',(6.94215892568192,-20.8006600571723,2.5572005349258));
#6557=CARTESIAN_POINT('Ctrl Pts',(6.9896300292816,-20.7925946396956,2.54640081720694));
#6558=CARTESIAN_POINT('Ctrl Pts',(7.03670647086889,-20.7846241154025,2.53442952081183));
#6559=CARTESIAN_POINT('Ctrl Pts',(7.08329575335921,-20.7767637068552,2.52133001886304));
#6560=CARTESIAN_POINT('Ctrl Pts',(7.15274622402516,-20.7650462249784,2.50180263987794));
#6561=CARTESIAN_POINT('Ctrl Pts',(7.22195029957584,-20.7538517587617,2.47959273545153));
#6562=CARTESIAN_POINT('Ctrl Pts',(7.29057405515975,-20.7432450259833,2.45474630344388));
#6563=CARTESIAN_POINT('Ctrl Pts',(7.3591070626117,-20.7326523195604,2.42993272838601));
#6564=CARTESIAN_POINT('Ctrl Pts',(7.42706058357602,-20.7226459347948,2.40248965699003));
#6565=CARTESIAN_POINT('Ctrl Pts',(7.49410526368581,-20.713280712891,2.37251384629915));
#6566=CARTESIAN_POINT('Ctrl Pts',(7.56115420453236,-20.7039148958208,2.34253613062434));
#6567=CARTESIAN_POINT('Ctrl Pts',(7.62729349814889,-20.69519043664,2.31002556527974));
#6568=CARTESIAN_POINT('Ctrl Pts',(7.69220745152933,-20.687150634337,2.27512786406365));
#6569=CARTESIAN_POINT('Ctrl Pts',(7.75710570026851,-20.6791127771045,2.240238605653));
#6570=CARTESIAN_POINT('Ctrl Pts',(7.82077856718671,-20.6717593202239,2.20296372939565));
#6571=CARTESIAN_POINT('Ctrl Pts',(7.88293428494723,-20.6651205676153,2.16349342564724));
#6572=CARTESIAN_POINT('Ctrl Pts',(7.94518447415883,-20.6584717246624,2.1239631303646));
#6573=CARTESIAN_POINT('Ctrl Pts',(8.00591234872199,-20.652539796222,2.08223120813799));
#6574=CARTESIAN_POINT('Ctrl Pts',(8.064857522614,-20.6473413793201,2.03852710839638));
#6575=CARTESIAN_POINT('Ctrl Pts',(8.10439888843787,-20.6438541980828,2.00920969898384));
#6576=CARTESIAN_POINT('Ctrl Pts',(8.14313874853075,-20.6406968013597,1.97900561592648));
#6577=CARTESIAN_POINT('Ctrl Pts',(8.18100842628527,-20.6378706589539,1.94799199564959));
#6578=CARTESIAN_POINT('Ctrl Pts',(8.23746061450179,-20.6336577389483,1.90176010689425));
#6579=CARTESIAN_POINT('Ctrl Pts',(8.29269916543629,-20.6305262721282,1.85331739425806));
#6580=CARTESIAN_POINT('Ctrl Pts',(8.34643501506069,-20.6285150758632,1.80284481408902));
#6581=CARTESIAN_POINT('Ctrl Pts',(8.40009980433667,-20.6265065392064,1.75243897891719));
#6582=CARTESIAN_POINT('Ctrl Pts',(8.45226524535692,-20.6256154066465,1.7000089916859));
#6583=CARTESIAN_POINT('Ctrl Pts',(8.50266515457153,-20.6258600476996,1.64577768116514));
#6584=CARTESIAN_POINT('Ctrl Pts',(8.55306826673607,-20.6261047042999,1.59154292420618));
#6585=CARTESIAN_POINT('Ctrl Pts',(8.60170506750094,-20.6274853140785,1.53550708982212));
#6586=CARTESIAN_POINT('Ctrl Pts',(8.64833992076498,-20.6299989551482,1.47792947798962));
#6587=CARTESIAN_POINT('Ctrl Pts',(8.69496349165288,-20.6325119880925,1.42036579591624));
#6588=CARTESIAN_POINT('Ctrl Pts',(8.73958563594783,-20.6361574710468,1.361261664062));
#6589=CARTESIAN_POINT('Ctrl Pts',(8.78200902118676,-20.6409111859313,1.30090464504851));
#6590=CARTESIAN_POINT('Ctrl Pts',(8.82449688639477,-20.6456721260617,1.24045588845447));
#6591=CARTESIAN_POINT('Ctrl Pts',(8.8647789760219,-20.6515445770579,1.17875107963639));
#6592=CARTESIAN_POINT('Ctrl Pts',(8.90270117211557,-20.658483782047,1.11609838715458));
#6593=CARTESIAN_POINT('Ctrl Pts',(8.92813998804528,-20.6631387117873,1.07406995853698));
#6594=CARTESIAN_POINT('Ctrl Pts',(8.95251779902157,-20.6682732479878,1.03161537789573));
#6595=CARTESIAN_POINT('Ctrl Pts',(8.97580007665302,-20.6738691449698,0.988830267143716));
#6596=CARTESIAN_POINT('Ctrl Pts',(9.01050688159292,-20.6822109278527,0.925050661183007));
#6597=CARTESIAN_POINT('Ctrl Pts',(9.04330583807951,-20.6920349669275,0.859969813685453));
#6598=CARTESIAN_POINT('Ctrl Pts',(9.07399901152766,-20.7033274659558,0.793867798863035));
#6599=CARTESIAN_POINT('Ctrl Pts',(9.10465159628846,-20.7146050317706,0.727853197419915));
#6600=CARTESIAN_POINT('Ctrl Pts',(9.13320352671783,-20.7273471659068,0.660820696335935));
#6601=CARTESIAN_POINT('Ctrl Pts',(9.15949290620382,-20.7415120277891,0.593075062137148));
#6602=CARTESIAN_POINT('Ctrl Pts',(9.18578395639847,-20.7556777898584,0.525325122655411));
#6603=CARTESIAN_POINT('Ctrl Pts',(9.20981183404347,-20.7712663680247,0.456862603466087));
#6604=CARTESIAN_POINT('Ctrl Pts',(9.23145571231611,-20.7882085552331,0.388009033183664));
#6605=CARTESIAN_POINT('Ctrl Pts',(9.25309435428247,-20.8051466436159,0.319172120654451));
#6606=CARTESIAN_POINT('Ctrl Pts',(9.27234995304531,-20.8234375084615,0.249945031381689));
#6607=CARTESIAN_POINT('Ctrl Pts',(9.2891468470743,-20.8429866849445,0.180655744949017));
#6608=CARTESIAN_POINT('Ctrl Pts',(9.30596927096614,-20.8625655745276,0.111261144642447));
#6609=CARTESIAN_POINT('Ctrl Pts',(9.32032544605971,-20.8834063592587,0.041804843379192));
#6610=CARTESIAN_POINT('Ctrl Pts',(9.33218657768053,-20.9053919268366,-0.0273873077118918));
#6611=CARTESIAN_POINT('Ctrl Pts',(9.3401432145608,-20.9201401973571,-0.0738025098018784));
#6612=CARTESIAN_POINT('Ctrl Pts',(9.34697808876498,-20.9354031528252,-0.120098937659683));
#6613=CARTESIAN_POINT('Ctrl Pts',(9.35269438438333,-20.9511407742511,-0.166181422977341));
#6614=CARTESIAN_POINT('Ctrl Pts',(9.36121564506691,-20.9746007881591,-0.234876412977098));
#6615=CARTESIAN_POINT('Ctrl Pts',(9.3675453741578,-20.999706842796,-0.303705335324624));
#6616=CARTESIAN_POINT('Ctrl Pts',(9.3716049858295,-21.0263762358853,-0.372344470076549));
#6617=CARTESIAN_POINT('Ctrl Pts',(9.37565922906612,-21.0530103613389,-0.440892836358829));
#6618=CARTESIAN_POINT('Ctrl Pts',(9.37744916363083,-21.0812035409916,-0.509251242355766));
#6619=CARTESIAN_POINT('Ctrl Pts',(9.37693764066361,-21.1108419111196,-0.577093346533461));
#6620=CARTESIAN_POINT('Ctrl Pts',(9.37642608518874,-21.1404821647871,-0.644939762125091));
#6621=CARTESIAN_POINT('Ctrl Pts',(9.37361270847825,-21.171567548381,-0.712269124556508));
#6622=CARTESIAN_POINT('Ctrl Pts',(9.36850350597585,-21.2039556339764,-0.778761359260748));
#6623=CARTESIAN_POINT('Ctrl Pts',(9.36339553954347,-21.2363358839181,-0.845237507490097));
#6624=CARTESIAN_POINT('Ctrl Pts',(9.35599292530834,-21.2700178752143,-0.910876280136405));
#6625=CARTESIAN_POINT('Ctrl Pts',(9.34634481031159,-21.3048350847771,-0.975374241032964));
#6626=CARTESIAN_POINT('Ctrl Pts',(9.33668203099342,-21.3397052135631,-1.03997023339255));
#6627=CARTESIAN_POINT('Ctrl Pts',(9.32476710728983,-21.3757136242566,-1.10342135481028));
#6628=CARTESIAN_POINT('Ctrl Pts',(9.31069080120018,-21.4126741784787,-1.16544861040113));
#6629=CARTESIAN_POINT('Ctrl Pts',(9.3012481898413,-21.437467909654,-1.20705748594504));
#6630=CARTESIAN_POINT('Ctrl Pts',(9.29083383339552,-21.4626897130814,-1.24802618569427));
#6631=CARTESIAN_POINT('Ctrl Pts',(9.27948472328098,-21.4882800511012,-1.28827884419634));
#6632=CARTESIAN_POINT('Ctrl Pts',(9.26256664691328,-21.5264274731038,-1.34828333297726));
#6633=CARTESIAN_POINT('Ctrl Pts',(9.2436400707703,-21.5661152623663,-1.40722791797283));
#6634=CARTESIAN_POINT('Ctrl Pts',(9.22275033861447,-21.6071891658306,-1.46480935021324));
#6635=CARTESIAN_POINT('Ctrl Pts',(9.20188823106402,-21.6482087531186,-1.52231463670266));
#6636=CARTESIAN_POINT('Ctrl Pts',(9.17906822598555,-21.6906104880492,-1.57845972694475));
#6637=CARTESIAN_POINT('Ctrl Pts',(9.15437367526274,-21.7342109357619,-1.63296134034085));
#6638=CARTESIAN_POINT('Ctrl Pts',(9.12967755518386,-21.7778141543139,-1.68746641735284));
#6639=CARTESIAN_POINT('Ctrl Pts',(9.10310683249362,-21.8226158480044,-1.74032721705642));
#6640=CARTESIAN_POINT('Ctrl Pts',(9.07478121918489,-21.8684079346285,-1.79128851362561));
#6641=CARTESIAN_POINT('Ctrl Pts',(9.04646245869541,-21.9141889427672,-1.8422374811218));
#6642=CARTESIAN_POINT('Ctrl Pts',(9.01638995002209,-21.9609594037198,-1.89128737321232));
#6643=CARTESIAN_POINT('Ctrl Pts',(8.98471606654793,-22.0084931966421,-1.93821939640159));
#6644=CARTESIAN_POINT('Ctrl Pts',(8.95299404144121,-22.0560992369223,-1.98522275230941));
#6645=CARTESIAN_POINT('Ctrl Pts',(8.91966614798735,-22.1044704314653,-2.03010142110779));
#6646=CARTESIAN_POINT('Ctrl Pts',(8.88491325858982,-22.1533686166261,-2.07267852251415));
#6647=CARTESIAN_POINT('Ctrl Pts',(8.86160046430393,-22.1861703016477,-2.10123992341012));
#6648=CARTESIAN_POINT('Ctrl Pts',(8.83764700500886,-22.2192089097494,-2.12876654161632));
#6649=CARTESIAN_POINT('Ctrl Pts',(8.81311307834095,-22.2524115051551,-2.15521684061908));
#6650=CARTESIAN_POINT('Ctrl Pts',(8.77654044482297,-22.3019064910192,-2.19464620327117));
#6651=CARTESIAN_POINT('Ctrl Pts',(8.73857280660773,-22.3525876425948,-2.23203175294834));
#6652=CARTESIAN_POINT('Ctrl Pts',(8.69935947210196,-22.4042406828083,-2.26715077383193));
#6653=CARTESIAN_POINT('Ctrl Pts',(8.66019799335401,-22.4558254169831,-2.30222335328266));
#6654=CARTESIAN_POINT('Ctrl Pts',(8.61979440522145,-22.5083790383233,-2.33503490407258));
#6655=CARTESIAN_POINT('Ctrl Pts',(8.57832444667329,-22.5616647722598,-2.36540131373503));
#6656=CARTESIAN_POINT('Ctrl Pts',(8.53685185268005,-22.6149538925422,-2.39576965320422));
#6657=CARTESIAN_POINT('Ctrl Pts',(8.49431312612197,-22.6689747175642,-2.42369216050347));
#6658=CARTESIAN_POINT('Ctrl Pts',(8.45090606686655,-22.7234740810654,-2.44902900915278));
#6659=CARTESIAN_POINT('Ctrl Pts',(8.40750950908663,-22.7779602595285,-2.47435972805499));
#6660=CARTESIAN_POINT('Ctrl Pts',(8.36324547515667,-22.8329242014082,-2.49710580690364));
#6661=CARTESIAN_POINT('Ctrl Pts',(8.31832753732902,-22.8881044526766,-2.51717642960941));
#6662=CARTESIAN_POINT('Ctrl Pts',(8.27334132802268,-22.9433685732749,-2.53727755796965));
#6663=CARTESIAN_POINT('Ctrl Pts',(8.22769969513748,-22.9988491085934,-2.55469500339245));
#6664=CARTESIAN_POINT('Ctrl Pts',(8.18162632774061,-23.0542831747744,-2.56938903350697));
#6665=CARTESIAN_POINT('Ctrl Pts',(8.15071957567454,-23.0914692333648,-2.57924602402579));
#6666=CARTESIAN_POINT('Ctrl Pts',(8.11961872669561,-23.1286343888246,-2.5878785763622));
#6667=CARTESIAN_POINT('Ctrl Pts',(8.0883919872726,-23.1657010814762,-2.59528770975726));
#6668=CARTESIAN_POINT('Ctrl Pts',(8.04184240259629,-23.2209562627772,-2.60633247743792));
#6669=CARTESIAN_POINT('Ctrl Pts',(7.99482026133714,-23.2768650341225,-2.6147543251795));
#6670=CARTESIAN_POINT('Ctrl Pts',(7.94753828012866,-23.3331765096818,-2.62045518191379));
#6671=CARTESIAN_POINT('Ctrl Pts',(7.90031882466558,-23.3894135188822,-2.62614849982869));
#6672=CARTESIAN_POINT('Ctrl Pts',(7.85284065434047,-23.4460516521555,-2.62912778112528));
#6673=CARTESIAN_POINT('Ctrl Pts',(7.80532548315392,-23.5028275912359,-2.62934454720093));
#6674=CARTESIAN_POINT('Ctrl Pts',(7.75780729234462,-23.5596071384675,-2.62956132705223));
#6675=CARTESIAN_POINT('Ctrl Pts',(7.71025256303128,-23.6165239540305,-2.62701514692949));
#6676=CARTESIAN_POINT('Ctrl Pts',(7.66288608802028,-23.6733092872841,-2.62170927404788));
#6677=CARTESIAN_POINT('Ctrl Pts',(7.61553107238672,-23.7300808824546,-2.61640468481679));
#6678=CARTESIAN_POINT('Ctrl Pts',(7.56836468800612,-23.7867204971482,-2.60834181054537));
#6679=CARTESIAN_POINT('Ctrl Pts',(7.52160755734099,-23.8429626068964,-2.59757579979083));
#6680=CARTESIAN_POINT('Ctrl Pts',(7.47477935977912,-23.89929019991,-2.58679342560759));
#6681=CARTESIAN_POINT('Ctrl Pts',(7.4283621048939,-23.9552185407989,-2.57329990897789));
#6682=CARTESIAN_POINT('Ctrl Pts',(7.38256652431042,-24.0104922266885,-2.55720053492594));
#6683=CARTESIAN_POINT('Ctrl Pts',(7.35184611608344,-24.0475706996133,-2.54640081720705));
#6684=CARTESIAN_POINT('Ctrl Pts',(7.32140521877035,-24.0843548318013,-2.53442952081188));
#6685=CARTESIAN_POINT('Ctrl Pts',(7.29130326403902,-24.1207721297085,-2.52133001886304));
#6686=CARTESIAN_POINT('Ctrl Pts',(7.24643039173222,-24.1750592606718,-2.50180263987787));
#6687=CARTESIAN_POINT('Ctrl Pts',(7.20213366183125,-24.2293945150359,-2.47959273545138));
#6688=CARTESIAN_POINT('Ctrl Pts',(7.15863608400191,-24.2835210642857,-2.45474630344363));
#6689=CARTESIAN_POINT('Ctrl Pts',(7.11519602741874,-24.3375760365254,-2.42993272838569));
#6690=CARTESIAN_POINT('Ctrl Pts',(7.07255348352948,-24.3914223195744,-2.40248965698964));
#6691=CARTESIAN_POINT('Ctrl Pts',(7.0309206233938,-24.4448021047863,-2.37251384629869));
#6692=CARTESIAN_POINT('Ctrl Pts',(6.98928511746054,-24.4981852823212,-2.34253613062386));
#6693=CARTESIAN_POINT('Ctrl Pts',(6.94865986736745,-24.551101361191,-2.31002556527924));
#6694=CARTESIAN_POINT('Ctrl Pts',(6.90924021764144,-24.603298592727,-2.27512786406314));
#6695=CARTESIAN_POINT('Ctrl Pts',(6.8698301047165,-24.6554831961799,-2.24023860565251));
#6696=CARTESIAN_POINT('Ctrl Pts',(6.83162539079327,-24.7069487880225,-2.20296372939517));
#6697=CARTESIAN_POINT('Ctrl Pts',(6.79479820350458,-24.7574578422892,-2.16349342564679));
#6698=CARTESIAN_POINT('Ctrl Pts',(6.75791504199586,-24.8080436660604,-2.12396313036418));
#6699=CARTESIAN_POINT('Ctrl Pts',(6.72241390399149,-24.8576695839296,-2.08223120813761));
#6700=CARTESIAN_POINT('Ctrl Pts',(6.68843935594901,-24.9061183934996,-2.03852710839605));
#6701=CARTESIAN_POINT('Ctrl Pts',(6.66564868549808,-24.9386186301846,-2.0092096989836));
#6702=CARTESIAN_POINT('Ctrl Pts',(6.64354436967967,-24.9705896348024,-1.97900561592636));
#6703=CARTESIAN_POINT('Ctrl Pts',(6.62216201968439,-25.0019726665679,-1.94799199564959));
#6704=CARTESIAN_POINT('Ctrl Pts',(6.5902874298272,-25.0487552356599,-1.90176010689427));
#6705=CARTESIAN_POINT('Ctrl Pts',(6.5599562245426,-25.0950274906273,-1.8533173942581));
#6706=CARTESIAN_POINT('Ctrl Pts',(6.53134655267294,-25.1405585033634,-1.80284481408909));
#6707=CARTESIAN_POINT('Ctrl Pts',(6.50277471426566,-25.186029305837,-1.75243897891707));
#6708=CARTESIAN_POINT('Ctrl Pts',(6.47592025032039,-25.2307603366803,-1.70000899168558));
#6709=CARTESIAN_POINT('Ctrl Pts',(6.45093216107982,-25.2745302589353,-1.64577768116459));
#6710=CARTESIAN_POINT('Ctrl Pts',(6.42594248382858,-25.3183029627997,-1.59154292420563));
#6711=CARTESIAN_POINT('Ctrl Pts',(6.40281972658714,-25.3611139727102,-1.53550708982158));
#6712=CARTESIAN_POINT('Ctrl Pts',(6.38167917697755,-25.4027577608735,-1.47792947798907));
#6713=CARTESIAN_POINT('Ctrl Pts',(6.36054374190388,-25.4443914741496,-1.4203657959157));
#6714=CARTESIAN_POINT('Ctrl Pts',(6.34138975060389,-25.4848581261575,-1.36126166406147));
#6715=CARTESIAN_POINT('Ctrl Pts',(6.3242948958368,-25.5239747129312,-1.30090464504799));
#6716=CARTESIAN_POINT('Ctrl Pts',(6.30717405833167,-25.563150753619,-1.24045588845407));
#6717=CARTESIAN_POINT('Ctrl Pts',(6.29211870526331,-25.6009722920517,-1.17875107963611));
#6718=CARTESIAN_POINT('Ctrl Pts',(6.27916713501913,-25.6372834797305,-1.11609838715443));
#6719=CARTESIAN_POINT('Ctrl Pts',(6.27047901446228,-25.661641605438,-1.07406995853689));
#6720=CARTESIAN_POINT('Ctrl Pts',(6.26273674776036,-25.6853206771323,-1.03161537789568));
#6721=CARTESIAN_POINT('Ctrl Pts',(6.25594179788806,-25.7082816695101,-0.988830267143717));
#6722=CARTESIAN_POINT('Ctrl Pts',(6.24581259130752,-25.7425095357137,-0.925050661183071));
#6723=CARTESIAN_POINT('Ctrl Pts',(6.23792098047084,-25.7758262847861,-0.859969813685577));
#6724=CARTESIAN_POINT('Ctrl Pts',(6.23235398477746,-25.808053602229,-0.793867798863225));
#6725=CARTESIAN_POINT('Ctrl Pts',(6.22679435088548,-25.8402383022309,-0.727853197420082));
#6726=CARTESIAN_POINT('Ctrl Pts',(6.22355339753122,-25.871336066378,-0.660820696336077));
#6727=CARTESIAN_POINT('Ctrl Pts',(6.22267583801938,-25.9011857678037,-0.593075062137264));
#6728=CARTESIAN_POINT('Ctrl Pts',(6.22179822273801,-25.9310373661991,-0.525325122655538));
#6729=CARTESIAN_POINT('Ctrl Pts',(6.22328438861643,-25.9596404077219,-0.456862603466225));
#6730=CARTESIAN_POINT('Ctrl Pts',(6.2271348139982,-25.9868556497466,-0.388009033183813));
#6731=CARTESIAN_POINT('Ctrl Pts',(6.23098430784604,-26.0140643075841,-0.319172120654854));
#6732=CARTESIAN_POINT('Ctrl Pts',(6.23719686207813,-26.0398855777006,-0.249945031382356));
#6733=CARTESIAN_POINT('Ctrl Pts',(6.24572849852092,-26.0642067028758,-0.18065574494994));
#6734=CARTESIAN_POINT('Ctrl Pts',(6.25427310233184,-26.0885647941109,-0.111261144643501));
#6735=CARTESIAN_POINT('Ctrl Pts',(6.26514366379693,-26.1114179988086,-0.0418048433803723));
#6736=CARTESIAN_POINT('Ctrl Pts',(6.27825315802551,-26.1326828238988,0.0273873077105849));
#6737=CARTESIAN_POINT('Ctrl Pts',(6.2870472165181,-26.1469476088262,0.0738025098010098));
#6738=CARTESIAN_POINT('Ctrl Pts',(6.29684788658832,-26.1604982612529,0.120098937659253));
#6739=CARTESIAN_POINT('Ctrl Pts',(6.30761891872917,-26.1733175291869,0.166181422977344));
#6740=CARTESIAN_POINT('Ctrl Pts',(6.32367525640489,-26.1924271643652,0.234876412977188));
#6741=CARTESIAN_POINT('Ctrl Pts',(6.34225287296385,-26.2104618978755,0.303705335324803));
#6742=CARTESIAN_POINT('Ctrl Pts',(6.36331943904686,-26.2273123212574,0.372344470076813));
#6743=CARTESIAN_POINT('Ctrl Pts',(6.38435814667899,-26.2441404616202,0.440892836359177));
#6744=CARTESIAN_POINT('Ctrl Pts',(6.40787918918932,-26.2597871802507,0.509251242356202));
#6745=CARTESIAN_POINT('Ctrl Pts',(6.43380253213062,-26.2741633734305,0.577093346533977));
#6746=CARTESIAN_POINT('Ctrl Pts',(6.45972752251878,-26.2885404802276,0.644939762125664));
#6747=CARTESIAN_POINT('Ctrl Pts',(6.48805494275271,-26.3016467163228,0.712269124557124));
#6748=CARTESIAN_POINT('Ctrl Pts',(6.51865844890955,-26.3134160599604,0.778761359261416));
#6749=CARTESIAN_POINT('Ctrl Pts',(6.54925455115611,-26.3251825562391,0.845237507490585));
#6750=CARTESIAN_POINT('Ctrl Pts',(6.58212531838614,-26.3356126999051,0.910876280136723));
#6751=CARTESIAN_POINT('Ctrl Pts',(6.61710196385465,-26.3446657920006,0.975374241033112));
#6752=CARTESIAN_POINT('Ctrl Pts',(6.65213177087563,-26.3537326440329,1.03997023339268));
#6753=CARTESIAN_POINT('Ctrl Pts',(6.68927343113795,-26.3614182227682,1.10342135481039));
#6754=CARTESIAN_POINT('Ctrl Pts',(6.72832036307706,-26.3677080612142,1.16544861040121));
#6755=CARTESIAN_POINT('Ctrl Pts',(6.7545136698089,-26.371927385487,1.20705748594509));
#6756=CARTESIAN_POINT('Ctrl Pts',(6.78156357052916,-26.3755191899546,1.24802618569429));
#6757=CARTESIAN_POINT('Ctrl Pts',(6.80940000840295,-26.3784857412949,1.28827884419633));
#6758=CARTESIAN_POINT('Ctrl Pts',(6.85089568313002,-26.3829079683787,1.34828333297733));
#6759=CARTESIAN_POINT('Ctrl Pts',(6.89472960492293,-26.3863609672634,1.40722791797297));
#6760=CARTESIAN_POINT('Ctrl Pts',(6.94074551483355,-26.3888068802704,1.46480935021343));
#6761=CARTESIAN_POINT('Ctrl Pts',(6.98670057325275,-26.3912495587992,1.52231463670264));
#6762=CARTESIAN_POINT('Ctrl Pts',(7.03483155540622,-26.392687722152,1.57845972694453));
#6763=CARTESIAN_POINT('Ctrl Pts',(7.08493792610307,-26.3931018377474,1.63296134034044));
#6764=CARTESIAN_POINT('Ctrl Pts',(7.13504748109524,-26.3935159796601,1.68746641735244));
#6765=CARTESIAN_POINT('Ctrl Pts',(7.18713224730889,-26.3929059056587,1.74032721705603));
#6766=CARTESIAN_POINT('Ctrl Pts',(7.24095216427203,-26.3912712482677,1.79128851362524));
#6767=CARTESIAN_POINT('Ctrl Pts',(7.29475906057568,-26.3896369863495,1.84223748112135));
#6768=CARTESIAN_POINT('Ctrl Pts',(7.3502997222439,-26.3869786603592,1.89128737321179));
#6769=CARTESIAN_POINT('Ctrl Pts',(7.40730213618982,-26.3833151690952,1.93821939640099));
#6770=CARTESIAN_POINT('Ctrl Pts',(7.46439118899938,-26.3796461096334,1.98522275230886));
#6771=CARTESIAN_POINT('Ctrl Pts',(7.52294581901199,-26.3749689045192,2.03010142110728));
#6772=CARTESIAN_POINT('Ctrl Pts',(7.582669334259,-26.3693211120265,2.07267852251368));
#6773=CARTESIAN_POINT('Ctrl Pts',(7.62273282391778,-26.3655324824525,2.10123992340982));
#6774=CARTESIAN_POINT('Ctrl Pts',(7.66332182748728,-26.3613074822452,2.12876654161618));
#6775=CARTESIAN_POINT('Ctrl Pts',(7.7043430819144,-26.3566617761991,2.15521684061908));
#6776=CARTESIAN_POINT('Ctrl Pts',(7.76549331379184,-26.3497364394213,2.19464620327127));
#6777=CARTESIAN_POINT('Ctrl Pts',(7.8283682976571,-26.3421960759929,2.23203175294854));
#6778=CARTESIAN_POINT('Ctrl Pts',(7.89270780991775,-26.3340628522506,2.2671507738322));
#6779=CARTESIAN_POINT('Ctrl Pts',(7.95696223953461,-26.3259403838925,2.30222335328292));
#6780=CARTESIAN_POINT('Ctrl Pts',(8.02267680474233,-26.3172266608357,2.33503490407283));
#6781=CARTESIAN_POINT('Ctrl Pts',(8.08955858326471,-26.3079554902074,2.36540131373527));
#6782=CARTESIAN_POINT('Ctrl Pts',(8.15644461217124,-26.2986837303896,2.39576965320444));
#6783=CARTESIAN_POINT('Ctrl Pts',(8.22449738225272,-26.2888545250567,2.42369216050368));
#6784=CARTESIAN_POINT('Ctrl Pts',(8.29339874516257,-26.2785125907885,2.44902900915297));
#6785=CARTESIAN_POINT('Ctrl Pts',(8.36228343875657,-26.2681731585459,2.47435972805512));
#6786=CARTESIAN_POINT('Ctrl Pts',(8.43201562568134,-26.2573213516284,2.49710580690372));
#6787=CARTESIAN_POINT('Ctrl Pts',(8.50226209398065,-26.2460114020183,2.51717642960944));
#6788=CARTESIAN_POINT('Ctrl Pts',(8.57261533098984,-26.2346842622382,2.53727755796968));
#6789=CARTESIAN_POINT('Ctrl Pts',(8.64348370043378,-26.2228977163486,2.55469500339248));
#6790=CARTESIAN_POINT('Ctrl Pts',(8.71452769368014,-26.2107140428356,2.569389033507));
#6791=CARTESIAN_POINT('Ctrl Pts',(8.76218514111895,-26.202541039693,2.5792460240258));
#6792=CARTESIAN_POINT('Ctrl Pts',(8.80992153437213,-26.1941894921279,2.58787857636221));
#6793=CARTESIAN_POINT('Ctrl Pts',(8.85763560155417,-26.1856796888361,2.59528770975726));
#6794=CARTESIAN_POINT('Ctrl Pts',(8.92876278459006,-26.1729941566213,2.60633247743796));
#6795=CARTESIAN_POINT('Ctrl Pts',(9.00069227149935,-26.1602261734231,2.61475432517956));
#6796=CARTESIAN_POINT('Ctrl Pts',(9.07310043046284,-26.1474345143349,2.62045518191386));
#6797=CARTESIAN_POINT('Ctrl Pts',(9.14541283679517,-26.1346597709511,2.62614849982877));
#6798=CARTESIAN_POINT('Ctrl Pts',(9.21820198419582,-26.1218615359609,2.62912778112534));
#6799=CARTESIAN_POINT('Ctrl Pts',(9.29112897535694,-26.1091001601884,2.62934454720093));
#6800=CARTESIAN_POINT('Ctrl Pts',(9.36406060107956,-26.0963379734214,2.62956132705217));
#6801=CARTESIAN_POINT('Ctrl Pts',(9.43712937391635,-26.0836127775475,2.62701514692937));
#6802=CARTESIAN_POINT('Ctrl Pts',(9.5099901525818,-26.070984873527,2.6217092740477));
#6803=CARTESIAN_POINT('Ctrl Pts',(9.5828333040297,-26.0583600245769,2.61640468481655));
#6804=CARTESIAN_POINT('Ctrl Pts',(9.65546784140534,-26.0458325448455,2.60834181054505));
#6805=CARTESIAN_POINT('Ctrl Pts',(9.7275535025424,-26.0334607367555,2.59757579979043));
#6806=CARTESIAN_POINT('Ctrl Pts',(9.79974872780703,-26.0210701245603,2.58679342560712));
#6807=CARTESIAN_POINT('Ctrl Pts',(9.8713927192509,-26.0088357731002,2.57329990897737));
#6808=CARTESIAN_POINT('Ctrl Pts',(9.94215892568377,-25.9968124798787,2.55720053492538));
#6809=CARTESIAN_POINT('Ctrl Pts',(9.9896300292828,-25.988747062402,2.54640081720663));
#6810=CARTESIAN_POINT('Ctrl Pts',(10.0367064708695,-25.980776538109,2.53442952081165));
#6811=CARTESIAN_POINT('Ctrl Pts',(10.0832957533592,-25.9729161295619,2.52133001886304));
#6812=CARTESIAN_POINT('Ctrl Pts',(10.1527462240253,-25.9611986476851,2.50180263987788));
#6813=CARTESIAN_POINT('Ctrl Pts',(10.2219502995762,-25.9500041814683,2.47959273545139));
#6814=CARTESIAN_POINT('Ctrl Pts',(10.2905740551603,-25.9393974486899,2.45474630344365));
#6815=CARTESIAN_POINT('Ctrl Pts',(10.3591070626124,-25.9288047422669,2.42993272838573));
#6816=CARTESIAN_POINT('Ctrl Pts',(10.4270605835768,-25.9187983575013,2.40248965698969));
#6817=CARTESIAN_POINT('Ctrl Pts',(10.4941052636867,-25.9094331355976,2.37251384629875));
#6818=CARTESIAN_POINT('Ctrl Pts',(10.5611542045333,-25.9000673185274,2.3425361306239));
#6819=CARTESIAN_POINT('Ctrl Pts',(10.6272934981498,-25.8913428593466,2.31002556527924));
#6820=CARTESIAN_POINT('Ctrl Pts',(10.6922074515303,-25.8833030570436,2.2751278640631));
#6821=CARTESIAN_POINT('Ctrl Pts',(10.7571057002693,-25.875265199811,2.24023860565252));
#6822=CARTESIAN_POINT('Ctrl Pts',(10.8207785671873,-25.8679117429305,2.20296372939525));
#6823=CARTESIAN_POINT('Ctrl Pts',(10.8829342849477,-25.8612729903219,2.16349342564694));
#6824=CARTESIAN_POINT('Ctrl Pts',(10.9451844741592,-25.854624147369,2.12396313036433));
#6825=CARTESIAN_POINT('Ctrl Pts',(11.0059123487223,-25.8486922189286,2.08223120813775));
#6826=CARTESIAN_POINT('Ctrl Pts',(11.0648575226142,-25.8434938020267,2.03852710839618));
#6827=CARTESIAN_POINT('Ctrl Pts',(11.104398888438,-25.8400066207894,2.0092096989837));
#6828=CARTESIAN_POINT('Ctrl Pts',(11.1431387485308,-25.8368492240663,1.97900561592641));
#6829=CARTESIAN_POINT('Ctrl Pts',(11.1810084262852,-25.8340230816606,1.94799199564959));
#6830=CARTESIAN_POINT('Ctrl Pts',(11.2374606145019,-25.829810161655,1.90176010689413));
#6831=CARTESIAN_POINT('Ctrl Pts',(11.2926991654365,-25.8266786948348,1.8533173942578));
#6832=CARTESIAN_POINT('Ctrl Pts',(11.3464350150611,-25.8246674985698,1.80284481408862));
#6833=CARTESIAN_POINT('Ctrl Pts',(11.4000998043371,-25.8226589619131,1.7524389789167));
#6834=CARTESIAN_POINT('Ctrl Pts',(11.4522652453575,-25.8217678293531,1.7000089916853));
#6835=CARTESIAN_POINT('Ctrl Pts',(11.5026651545722,-25.8220124704063,1.64577768116442));
#6836=CARTESIAN_POINT('Ctrl Pts',(11.5530682667367,-25.8222571270065,1.59154292420547));
#6837=CARTESIAN_POINT('Ctrl Pts',(11.6017050675015,-25.8236377367852,1.53550708982144));
#6838=CARTESIAN_POINT('Ctrl Pts',(11.6483399207655,-25.8261513778549,1.47792947798895));
#6839=CARTESIAN_POINT('Ctrl Pts',(11.6949634916533,-25.8286644107992,1.42036579591568));
#6840=CARTESIAN_POINT('Ctrl Pts',(11.7395856359481,-25.8323098937535,1.36126166406155));
#6841=CARTESIAN_POINT('Ctrl Pts',(11.782009021187,-25.837063608638,1.30090464504817));
#6842=CARTESIAN_POINT('Ctrl Pts',(11.8244968863949,-25.8418245487684,1.24045588845423));
#6843=CARTESIAN_POINT('Ctrl Pts',(11.864778976022,-25.8476969997645,1.17875107963624));
#6844=CARTESIAN_POINT('Ctrl Pts',(11.9027011721156,-25.8546362047536,1.11609838715453));
#6845=CARTESIAN_POINT('Ctrl Pts',(11.9281399880453,-25.859291134494,1.07406995853695));
#6846=CARTESIAN_POINT('Ctrl Pts',(11.9525177990215,-25.8644256706944,1.03161537789571));
#6847=CARTESIAN_POINT('Ctrl Pts',(11.975800076653,-25.8700215676765,0.988830267143717));
#6848=CARTESIAN_POINT('Ctrl Pts',(12.0105068815926,-25.8783633505592,0.925050661183495));
#6849=CARTESIAN_POINT('Ctrl Pts',(12.043305838079,-25.888187389634,0.859969813686448));
#6850=CARTESIAN_POINT('Ctrl Pts',(12.0739990115269,-25.8994798886622,0.793867798864551));
#6851=CARTESIAN_POINT('Ctrl Pts',(12.1046515962878,-25.9107574544769,0.727853197421398));
#6852=CARTESIAN_POINT('Ctrl Pts',(12.1332035267172,-25.9234995886132,0.660820696337378));
#6853=CARTESIAN_POINT('Ctrl Pts',(12.1594929062032,-25.9376644504955,0.593075062138549));
#6854=CARTESIAN_POINT('Ctrl Pts',(12.1857839563979,-25.9518302125647,0.525325122656871));
#6855=CARTESIAN_POINT('Ctrl Pts',(12.2098118340429,-25.967418790731,0.456862603467601));
#6856=CARTESIAN_POINT('Ctrl Pts',(12.2314557123156,-25.9843609779393,0.388009033185234));
#6857=CARTESIAN_POINT('Ctrl Pts',(12.253094354282,-26.0012990663221,0.319172120656097));
#6858=CARTESIAN_POINT('Ctrl Pts',(12.2723499530448,-26.0195899311677,0.249945031383417));
#6859=CARTESIAN_POINT('Ctrl Pts',(12.2891468470738,-26.0391391076507,0.180655744950817));
#6860=CARTESIAN_POINT('Ctrl Pts',(12.3059692709657,-26.0587179972338,0.111261144644251));
#6861=CARTESIAN_POINT('Ctrl Pts',(12.3203254460593,-26.0795587819648,0.0418048433809942));
#6862=CARTESIAN_POINT('Ctrl Pts',(12.3321865776802,-26.1015443495427,-0.0273873077100924));
#6863=CARTESIAN_POINT('Ctrl Pts',(12.3401432145606,-26.1162926200634,-0.0738025098006832));
#6864=CARTESIAN_POINT('Ctrl Pts',(12.3469780887649,-26.1315555755317,-0.120098937659091));
#6865=CARTESIAN_POINT('Ctrl Pts',(12.3526943843833,-26.1472931969577,-0.166181422977345));
#6866=CARTESIAN_POINT('Ctrl Pts',(12.3612156450669,-26.1707532108657,-0.234876412977034));
#6867=CARTESIAN_POINT('Ctrl Pts',(12.3675453741578,-26.1958592655026,-0.303705335324481));
#6868=CARTESIAN_POINT('Ctrl Pts',(12.3716049858295,-26.2225286585919,-0.372344470076339));
#6869=CARTESIAN_POINT('Ctrl Pts',(12.3756592290661,-26.2491627840458,-0.440892836359306));
#6870=CARTESIAN_POINT('Ctrl Pts',(12.3774491636308,-26.2773559636987,-0.509251242356935));
#6871=CARTESIAN_POINT('Ctrl Pts',(12.3769376406636,-26.3069943338271,-0.577093346535299));
#6872=CARTESIAN_POINT('Ctrl Pts',(12.3764260851887,-26.3366345874946,-0.644939762127014));
#6873=CARTESIAN_POINT('Ctrl Pts',(12.3736127084781,-26.3677199710885,-0.712269124558506));
#6874=CARTESIAN_POINT('Ctrl Pts',(12.3685035059757,-26.4001080566841,-0.778761359262821));
#6875=CARTESIAN_POINT('Ctrl Pts',(12.3633955395432,-26.4324883066258,-0.845237507492121));
#6876=CARTESIAN_POINT('Ctrl Pts',(12.3559929253081,-26.466170297922,-0.910876280138376));
#6877=CARTESIAN_POINT('Ctrl Pts',(12.3463448103113,-26.5009875074848,-0.975374241034882));
#6878=CARTESIAN_POINT('Ctrl Pts',(12.3366820309931,-26.5358576362707,-1.03997023339422));
#6879=CARTESIAN_POINT('Ctrl Pts',(12.3247671072895,-26.5718660469641,-1.10342135481171));
#6880=CARTESIAN_POINT('Ctrl Pts',(12.3106908011999,-26.6088266011861,-1.16544861040232));
#6881=CARTESIAN_POINT('Ctrl Pts',(12.3012481898411,-26.6336203323612,-1.20705748594582));
#6882=CARTESIAN_POINT('Ctrl Pts',(12.2908338333954,-26.6588421357883,-1.24802618569465));
#6883=CARTESIAN_POINT('Ctrl Pts',(12.279484723281,-26.6844324738078,-1.28827884419634));
#6884=CARTESIAN_POINT('Ctrl Pts',(12.2625666469133,-26.7225798958103,-1.34828333297698));
#6885=CARTESIAN_POINT('Ctrl Pts',(12.2436400707704,-26.7622676850726,-1.40722791797229));
#6886=CARTESIAN_POINT('Ctrl Pts',(12.2227503386147,-26.8033415885367,-1.46480935021245));
#6887=CARTESIAN_POINT('Ctrl Pts',(12.2018882310643,-26.8443611758246,-1.52231463670186));
#6888=CARTESIAN_POINT('Ctrl Pts',(12.1790682259859,-26.8867629107552,-1.57845972694394));
#6889=CARTESIAN_POINT('Ctrl Pts',(12.1543736752631,-26.9303633584679,-1.63296134034003));
#6890=CARTESIAN_POINT('Ctrl Pts',(12.1296775551842,-26.9739665770198,-1.68746641735199));
#6891=CARTESIAN_POINT('Ctrl Pts',(12.103106832494,-27.0187682707103,-1.74032721705555));
#6892=CARTESIAN_POINT('Ctrl Pts',(12.0747812191854,-27.0645603573343,-1.79128851362472));
#6893=CARTESIAN_POINT('Ctrl Pts',(12.0464624586959,-27.110341365473,-1.84223748112084));
#6894=CARTESIAN_POINT('Ctrl Pts',(12.0163899500227,-27.1571118264255,-1.89128737321128));
#6895=CARTESIAN_POINT('Ctrl Pts',(11.9847160665486,-27.2046456193477,-1.93821939640049));
#6896=CARTESIAN_POINT('Ctrl Pts',(11.9529940414419,-27.2522516596279,-1.98522275230842));
#6897=CARTESIAN_POINT('Ctrl Pts',(11.919666147988,-27.300622854171,-2.0301014211069));
#6898=CARTESIAN_POINT('Ctrl Pts',(11.8849132585904,-27.3495210393319,-2.07267852251336));
#6899=CARTESIAN_POINT('Ctrl Pts',(11.8616004643043,-27.3823227243537,-2.10123992340961));
#6900=CARTESIAN_POINT('Ctrl Pts',(11.8376470050091,-27.4153613324557,-2.12876654161608));
#6901=CARTESIAN_POINT('Ctrl Pts',(11.8131130783409,-27.4485639278618,-2.15521684061907));
#6902=CARTESIAN_POINT('Ctrl Pts',(11.776540444823,-27.4980589137259,-2.19464620327115));
#6903=CARTESIAN_POINT('Ctrl Pts',(11.7385728066077,-27.5487400653014,-2.23203175294831));
#6904=CARTESIAN_POINT('Ctrl Pts',(11.699359472102,-27.6003931055149,-2.26715077383189));
#6905=CARTESIAN_POINT('Ctrl Pts',(11.6601979933545,-27.6519778396891,-2.30222335328218));
#6906=CARTESIAN_POINT('Ctrl Pts',(11.6197944052225,-27.7045314610286,-2.33503490407172));
#6907=CARTESIAN_POINT('Ctrl Pts',(11.5783244466749,-27.7578171949644,-2.36540131373386));
#6908=CARTESIAN_POINT('Ctrl Pts',(11.5368518526816,-27.8111063152468,-2.39576965320312));
#6909=CARTESIAN_POINT('Ctrl Pts',(11.4943131261236,-27.8651271402688,-2.42369216050245));
#6910=CARTESIAN_POINT('Ctrl Pts',(11.4509060668681,-27.91962650377,-2.44902900915183));
#6911=CARTESIAN_POINT('Ctrl Pts',(11.4075095090882,-27.9741126822331,-2.4743597280541));
#6912=CARTESIAN_POINT('Ctrl Pts',(11.3632454751583,-28.0290766241127,-2.49710580690281));
#6913=CARTESIAN_POINT('Ctrl Pts',(11.3183275373307,-28.0842568753811,-2.51717642960864));
#6914=CARTESIAN_POINT('Ctrl Pts',(11.2733413280244,-28.1395209959794,-2.53727755796891));
#6915=CARTESIAN_POINT('Ctrl Pts',(11.2276996951393,-28.1950015312977,-2.55469500339175));
#6916=CARTESIAN_POINT('Ctrl Pts',(11.1816263277426,-28.2504355974787,-2.56938903350633));
#6917=CARTESIAN_POINT('Ctrl Pts',(11.1507195756758,-28.2876216560698,-2.57924602402541));
#6918=CARTESIAN_POINT('Ctrl Pts',(11.1196187266963,-28.3247868115304,-2.58787857636204));
#6919=CARTESIAN_POINT('Ctrl Pts',(11.0883919872726,-28.3618535041829,-2.59528770975725));
#6920=CARTESIAN_POINT('Ctrl Pts',(11.0418424025962,-28.417108685484,-2.60633247743792));
#6921=CARTESIAN_POINT('Ctrl Pts',(10.994820261337,-28.4730174568294,-2.61475432517951));
#6922=CARTESIAN_POINT('Ctrl Pts',(10.9475382801284,-28.5293289323887,-2.6204551819138));
#6923=CARTESIAN_POINT('Ctrl Pts',(10.9003188246655,-28.5855659415888,-2.62614849982868));
#6924=CARTESIAN_POINT('Ctrl Pts',(10.8528406543406,-28.642204074862,-2.62912778112526));
#6925=CARTESIAN_POINT('Ctrl Pts',(10.8053254831542,-28.6989800139423,-2.62934454720093));
#6926=CARTESIAN_POINT('Ctrl Pts',(10.7578072923449,-28.7557595611739,-2.62956132705223));
#6927=CARTESIAN_POINT('Ctrl Pts',(10.7102525630315,-28.8126763767369,-2.6270151469295));
#6928=CARTESIAN_POINT('Ctrl Pts',(10.6628860880205,-28.8694617099905,-2.62170927404791));
#6929=CARTESIAN_POINT('Ctrl Pts',(10.6155310723873,-28.9262333051604,-2.61640468481687));
#6930=CARTESIAN_POINT('Ctrl Pts',(10.5683646880072,-28.9828729198536,-2.60834181054555));
#6931=CARTESIAN_POINT('Ctrl Pts',(10.5216075573424,-29.0391150296013,-2.59757579979117));
#6932=CARTESIAN_POINT('Ctrl Pts',(10.4747793597805,-29.0954426226149,-2.58679342560797));
#6933=CARTESIAN_POINT('Ctrl Pts',(10.4283621048952,-29.1513709635039,-2.57329990897831));
#6934=CARTESIAN_POINT('Ctrl Pts',(10.3825665243117,-29.2066446493936,-2.55720053492641));
#6935=CARTESIAN_POINT('Ctrl Pts',(10.3518461160843,-29.2437231223189,-2.54640081720739));
#6936=CARTESIAN_POINT('Ctrl Pts',(10.3214052187707,-29.2805072545074,-2.53442952081207));
#6937=CARTESIAN_POINT('Ctrl Pts',(10.291303264039,-29.3169245524152,-2.52133001886304));
#6938=CARTESIAN_POINT('Ctrl Pts',(10.2464303917322,-29.3712116833784,-2.50180263987789));
#6939=CARTESIAN_POINT('Ctrl Pts',(10.2021336618313,-29.4255469377425,-2.47959273545141));
#6940=CARTESIAN_POINT('Ctrl Pts',(10.158636084002,-29.4796734869922,-2.45474630344369));
#6941=CARTESIAN_POINT('Ctrl Pts',(10.1151960274185,-29.5337284592323,-2.4299327283856));
#6942=CARTESIAN_POINT('Ctrl Pts',(10.072553483529,-29.5875747422816,-2.40248965698937));
#6943=CARTESIAN_POINT('Ctrl Pts',(10.0309206233931,-29.6409545274939,-2.3725138462982));
#6944=CARTESIAN_POINT('Ctrl Pts',(9.98928511745983,-29.6943377050287,-2.34253613062334));
#6945=CARTESIAN_POINT('Ctrl Pts',(9.94865986736672,-29.7472537838986,-2.31002556527867));
#6946=CARTESIAN_POINT('Ctrl Pts',(9.90924021764072,-29.7994510154346,-2.27512786406253));
#6947=CARTESIAN_POINT('Ctrl Pts',(9.86983010471572,-29.8516356188876,-2.24023860565181));
#6948=CARTESIAN_POINT('Ctrl Pts',(9.83162539079244,-29.9031012107303,-2.20296372939438));
#6949=CARTESIAN_POINT('Ctrl Pts',(9.79479820350371,-29.953610264997,-2.1634934256459));
#6950=CARTESIAN_POINT('Ctrl Pts',(9.757915041995,-30.0041960887682,-2.12396313036324));
#6951=CARTESIAN_POINT('Ctrl Pts',(9.72241390399064,-30.0538220066374,-2.08223120813662));
#6952=CARTESIAN_POINT('Ctrl Pts',(9.68843935594817,-30.1022708162074,-2.03852710839501));
#6953=CARTESIAN_POINT('Ctrl Pts',(9.66564868549753,-30.134771052892,-2.00920969898289));
#6954=CARTESIAN_POINT('Ctrl Pts',(9.64354436967938,-30.1667420575094,-1.97900561592599));
#6955=CARTESIAN_POINT('Ctrl Pts',(9.62216201968436,-30.1981250892746,-1.94799199564958));
#6956=CARTESIAN_POINT('Ctrl Pts',(9.59028742982723,-30.2449076583664,-1.90176010689435));
#6957=CARTESIAN_POINT('Ctrl Pts',(9.55995622454268,-30.2911799133338,-1.85331739425826));
#6958=CARTESIAN_POINT('Ctrl Pts',(9.53134655267306,-30.3367109260699,-1.80284481408935));
#6959=CARTESIAN_POINT('Ctrl Pts',(9.50277471426597,-30.3821817285431,-1.75243897891767));
#6960=CARTESIAN_POINT('Ctrl Pts',(9.47592025032086,-30.4269127593862,-1.70000899168654));
#6961=CARTESIAN_POINT('Ctrl Pts',(9.45093216108043,-30.4706826816409,-1.64577768116595));
#6962=CARTESIAN_POINT('Ctrl Pts',(9.42594248382916,-30.5144553855053,-1.59154292420704));
#6963=CARTESIAN_POINT('Ctrl Pts',(9.4028197265877,-30.5572663954157,-1.53550708982303));
#6964=CARTESIAN_POINT('Ctrl Pts',(9.38167917697807,-30.598910183579,-1.47792947799057));
#6965=CARTESIAN_POINT('Ctrl Pts',(9.36054374190446,-30.640543896855,-1.42036579591748));
#6966=CARTESIAN_POINT('Ctrl Pts',(9.34138975060452,-30.6810105488628,-1.36126166406354));
#6967=CARTESIAN_POINT('Ctrl Pts',(9.32429489583745,-30.7201271356363,-1.30090464505035));
#6968=CARTESIAN_POINT('Ctrl Pts',(9.30717405833223,-30.7593031763242,-1.24045588845638));
#6969=CARTESIAN_POINT('Ctrl Pts',(9.2921187052638,-30.797124714757,-1.17875107963836));
#6970=CARTESIAN_POINT('Ctrl Pts',(9.27916713501956,-30.8334359024359,-1.11609838715662));
#6971=CARTESIAN_POINT('Ctrl Pts',(9.27047901446252,-30.8577940281439,-1.07406995853836));
#6972=CARTESIAN_POINT('Ctrl Pts',(9.26273674776045,-30.8814730998386,-1.03161537789642));
#6973=CARTESIAN_POINT('Ctrl Pts',(9.25594179788803,-30.9044340922168,-0.988830267143717));
#6974=CARTESIAN_POINT('Ctrl Pts',(9.24581259130754,-30.9386619584202,-0.925050661183348));
#6975=CARTESIAN_POINT('Ctrl Pts',(9.23792098047089,-30.9719787074924,-0.859969813686147));
#6976=CARTESIAN_POINT('Ctrl Pts',(9.23235398477751,-31.0042060249353,-0.793867798864092));
#6977=CARTESIAN_POINT('Ctrl Pts',(9.22679435088552,-31.0363907249372,-0.727853197420999));
#6978=CARTESIAN_POINT('Ctrl Pts',(9.22355339753123,-31.0674884890842,-0.660820696337054));
#6979=CARTESIAN_POINT('Ctrl Pts',(9.22267583801937,-31.09733819051,-0.593075062138292));
#6980=CARTESIAN_POINT('Ctrl Pts',(9.22179822273798,-31.1271897889054,-0.525325122656501));
#6981=CARTESIAN_POINT('Ctrl Pts',(9.22328438861637,-31.1557928304282,-0.456862603467119));
#6982=CARTESIAN_POINT('Ctrl Pts',(9.22713481399813,-31.1830080724529,-0.388009033184638));
#6983=CARTESIAN_POINT('Ctrl Pts',(9.23098430784596,-31.2102167302905,-0.319172120655617));
#6984=CARTESIAN_POINT('Ctrl Pts',(9.23719686207803,-31.236038000407,-0.249945031383046));
#6985=CARTESIAN_POINT('Ctrl Pts',(9.24572849852081,-31.2603591255822,-0.180655744950565));
#6986=CARTESIAN_POINT('Ctrl Pts',(9.25427310233174,-31.2847172168174,-0.111261144643989));
#6987=CARTESIAN_POINT('Ctrl Pts',(9.26514366379684,-31.3075704215151,-0.0418048433807318));
#6988=CARTESIAN_POINT('Ctrl Pts',(9.27825315802543,-31.3288352466054,0.0273873077103627));
#6989=CARTESIAN_POINT('Ctrl Pts',(9.28704721651805,-31.3431000315328,0.0738025098008598));
#6990=CARTESIAN_POINT('Ctrl Pts',(9.29684788658827,-31.3566506839595,0.120098937659176));
#6991=CARTESIAN_POINT('Ctrl Pts',(9.30761891872914,-31.3694699518936,0.166181422977337));
#6992=CARTESIAN_POINT('Ctrl Pts',(9.32367525640488,-31.3885795870719,0.234876412977284));
#6993=CARTESIAN_POINT('Ctrl Pts',(9.34225287296387,-31.4066143205822,0.303705335324998));
#6994=CARTESIAN_POINT('Ctrl Pts',(9.36331943904692,-31.4234647439641,0.37234447007711));
#6995=CARTESIAN_POINT('Ctrl Pts',(9.38435814667911,-31.440292884327,0.440892836359643));
#6996=CARTESIAN_POINT('Ctrl Pts',(9.40787918918951,-31.4559396029575,0.509251242356834));
#6997=CARTESIAN_POINT('Ctrl Pts',(9.4338025321309,-31.4703157961373,0.577093346534773));
#6998=CARTESIAN_POINT('Ctrl Pts',(9.45972752251909,-31.4846929029344,0.644939762126485));
#6999=CARTESIAN_POINT('Ctrl Pts',(9.48805494275305,-31.4977991390296,0.712269124557971));
#7000=CARTESIAN_POINT('Ctrl Pts',(9.51865844890992,-31.5095684826672,0.778761359262283));
#7001=CARTESIAN_POINT('Ctrl Pts',(9.54925455115649,-31.5213349789459,0.84523750749142));
#7002=CARTESIAN_POINT('Ctrl Pts',(9.58212531838652,-31.5317651226119,0.910876280137526));
#7003=CARTESIAN_POINT('Ctrl Pts',(9.61710196385504,-31.5408182147074,0.975374241033881));
#7004=CARTESIAN_POINT('Ctrl Pts',(9.6521317708761,-31.5498850667397,1.03997023339355));
#7005=CARTESIAN_POINT('Ctrl Pts',(9.6892734311385,-31.557570645475,1.10342135481135));
#7006=CARTESIAN_POINT('Ctrl Pts',(9.7283203630777,-31.563860483921,1.16544861040227));
#7007=CARTESIAN_POINT('Ctrl Pts',(9.75451366980933,-31.5680798081937,1.20705748594579));
#7008=CARTESIAN_POINT('Ctrl Pts',(9.78156357052936,-31.5716716126613,1.24802618569463));
#7009=CARTESIAN_POINT('Ctrl Pts',(9.80940000840292,-31.5746381640016,1.28827884419634));
#7010=CARTESIAN_POINT('Ctrl Pts',(9.85089568312997,-31.5790603910853,1.34828333297731));
#7011=CARTESIAN_POINT('Ctrl Pts',(9.89472960492287,-31.5825133899701,1.40722791797293));
#7012=CARTESIAN_POINT('Ctrl Pts',(9.94074551483348,-31.584959302977,1.46480935021338));
#7013=CARTESIAN_POINT('Ctrl Pts',(9.98670057325285,-31.5874019815058,1.52231463670281));
#7014=CARTESIAN_POINT('Ctrl Pts',(10.0348315554065,-31.5888401448587,1.57845972694491));
#7015=CARTESIAN_POINT('Ctrl Pts',(10.0849379261036,-31.5892542604541,1.63296134034101));
#7016=CARTESIAN_POINT('Ctrl Pts',(10.1350474810957,-31.5896684023668,1.68746641735299));
#7017=CARTESIAN_POINT('Ctrl Pts',(10.1871322473094,-31.5890583283654,1.74032721705655));
#7018=CARTESIAN_POINT('Ctrl Pts',(10.2409521642725,-31.5874236709743,1.79128851362573));
#7019=CARTESIAN_POINT('Ctrl Pts',(10.294759060576,-31.5857894090561,1.84223748112165));
#7020=CARTESIAN_POINT('Ctrl Pts',(10.350299722244,-31.5831310830658,1.89128737321192));
#7021=CARTESIAN_POINT('Ctrl Pts',(10.4073021361898,-31.5794675918019,1.93821939640097));
#7022=CARTESIAN_POINT('Ctrl Pts',(10.4643911889991,-31.5757985323401,1.98522275230865));
#7023=CARTESIAN_POINT('Ctrl Pts',(10.5229458190115,-31.5711213272259,2.03010142110689));
#7024=CARTESIAN_POINT('Ctrl Pts',(10.5826693342582,-31.5654735347332,2.07267852251315));
#7025=CARTESIAN_POINT('Ctrl Pts',(10.6227328239173,-31.5616849051592,2.10123992340947));
#7026=CARTESIAN_POINT('Ctrl Pts',(10.663321827487,-31.5574599049519,2.12876654161601));
#7027=CARTESIAN_POINT('Ctrl Pts',(10.7043430819144,-31.5528141989058,2.15521684061908));
#7028=CARTESIAN_POINT('Ctrl Pts',(10.7654933137918,-31.5458888621279,2.19464620327128));
#7029=CARTESIAN_POINT('Ctrl Pts',(10.8283682976571,-31.5383484986996,2.23203175294854));
#7030=CARTESIAN_POINT('Ctrl Pts',(10.8927078099178,-31.5302152749572,2.26715077383221));
#7031=CARTESIAN_POINT('Ctrl Pts',(10.9569622395341,-31.5220928065992,2.30222335328266));
#7032=CARTESIAN_POINT('Ctrl Pts',(11.0226768047413,-31.5133790835425,2.33503490407232));
#7033=CARTESIAN_POINT('Ctrl Pts',(11.0895585832631,-31.5041079129142,2.36540131373456));
#7034=CARTESIAN_POINT('Ctrl Pts',(11.1564446121696,-31.4948361530965,2.39576965320377));
#7035=CARTESIAN_POINT('Ctrl Pts',(11.2244973822511,-31.4850069477636,2.42369216050305));
#7036=CARTESIAN_POINT('Ctrl Pts',(11.2933987451609,-31.4746650134954,2.44902900915238));
#7037=CARTESIAN_POINT('Ctrl Pts',(11.362283438755,-31.4643255812527,2.47435972805461));
#7038=CARTESIAN_POINT('Ctrl Pts',(11.4320156256799,-31.4534737743353,2.49710580690326));
#7039=CARTESIAN_POINT('Ctrl Pts',(11.5022620939793,-31.4421638247251,2.51717642960905));
#7040=CARTESIAN_POINT('Ctrl Pts',(11.5726153309883,-31.4308366849451,2.53727755796928));
#7041=CARTESIAN_POINT('Ctrl Pts',(11.6434837004321,-31.4190501390555,2.55469500339208));
#7042=CARTESIAN_POINT('Ctrl Pts',(11.7145276936783,-31.4068664655425,2.56938903350662));
#7043=CARTESIAN_POINT('Ctrl Pts',(11.7621851411177,-31.3986934623999,2.57924602402558));
#7044=CARTESIAN_POINT('Ctrl Pts',(11.8099215343715,-31.3903419148347,2.58787857636211));
#7045=CARTESIAN_POINT('Ctrl Pts',(11.8576356015541,-31.3818321115427,2.59528770975726));
#7046=CARTESIAN_POINT('Ctrl Pts',(11.92876278459,-31.3691465793279,2.60633247743796));
#7047=CARTESIAN_POINT('Ctrl Pts',(12.0006922714993,-31.3563785961297,2.61475432517957));
#7048=CARTESIAN_POINT('Ctrl Pts',(12.0731004304628,-31.3435869370415,2.62045518191386));
#7049=CARTESIAN_POINT('Ctrl Pts',(12.1454128367948,-31.3308121936578,2.62614849982874));
#7050=CARTESIAN_POINT('Ctrl Pts',(12.218201984195,-31.3180139586677,2.62912778112531));
#7051=CARTESIAN_POINT('Ctrl Pts',(12.2911289753557,-31.3052525828952,2.62934454720093));
#7052=CARTESIAN_POINT('Ctrl Pts',(12.3640606010783,-31.2924903961283,2.6295613270522));
#7053=CARTESIAN_POINT('Ctrl Pts',(12.4371293739151,-31.2797652002543,2.62701514692943));
#7054=CARTESIAN_POINT('Ctrl Pts',(12.5099901525806,-31.2671372962338,2.62170927404779));
#7055=CARTESIAN_POINT('Ctrl Pts',(12.5828333040285,-31.2545124472838,2.61640468481667));
#7056=CARTESIAN_POINT('Ctrl Pts',(12.655467841404,-31.2419849675523,2.60834181054521));
#7057=CARTESIAN_POINT('Ctrl Pts',(12.727553502541,-31.2296131594624,2.59757579979063));
#7058=CARTESIAN_POINT('Ctrl Pts',(12.7997487278055,-31.2172225472672,2.58679342560739));
#7059=CARTESIAN_POINT('Ctrl Pts',(12.8713927192491,-31.2049881958071,2.57329990897772));
#7060=CARTESIAN_POINT('Ctrl Pts',(12.9421589256818,-31.1929649025856,2.55720053492581));
#7061=CARTESIAN_POINT('Ctrl Pts',(12.9896300292815,-31.1848994851089,2.54640081720695));
#7062=CARTESIAN_POINT('Ctrl Pts',(13.0367064708688,-31.1769289608158,2.53442952081183));
#7063=CARTESIAN_POINT('Ctrl Pts',(13.0832957533592,-31.1690685522685,2.52133001886305));
#7064=CARTESIAN_POINT('Ctrl Pts',(13.152746224025,-31.1573510703918,2.50180263987797));
#7065=CARTESIAN_POINT('Ctrl Pts',(13.2219502995756,-31.1461566041751,2.4795927354516));
#7066=CARTESIAN_POINT('Ctrl Pts',(13.2905740551594,-31.1355498713967,2.454746303444));
#7067=CARTESIAN_POINT('Ctrl Pts',(13.3591070626113,-31.1249571649737,2.42993272838613));
#7068=CARTESIAN_POINT('Ctrl Pts',(13.4270605835757,-31.1149507802081,2.40248965699016));
#7069=CARTESIAN_POINT('Ctrl Pts',(13.4941052636855,-31.1055855583044,2.37251384629929));
#7070=CARTESIAN_POINT('Ctrl Pts',(13.561154204532,-31.0962197412342,2.3425361306245));
#7071=CARTESIAN_POINT('Ctrl Pts',(13.6272934981485,-31.0874952820534,2.31002556527993));
#7072=CARTESIAN_POINT('Ctrl Pts',(13.6922074515289,-31.0794554797504,2.27512786406386));
#7073=CARTESIAN_POINT('Ctrl Pts',(13.7571057002679,-31.0714176225178,2.2402386056533));
#7074=CARTESIAN_POINT('Ctrl Pts',(13.820778567186,-31.0640641656373,2.20296372939604));
#7075=CARTESIAN_POINT('Ctrl Pts',(13.8829342849464,-31.0574254130287,2.16349342564774));
#7076=CARTESIAN_POINT('Ctrl Pts',(13.9451844741581,-31.0507765700758,2.12396313036507));
#7077=CARTESIAN_POINT('Ctrl Pts',(14.0059123487213,-31.0448446416354,2.08223120813844));
#7078=CARTESIAN_POINT('Ctrl Pts',(14.0648575226134,-31.0396462247334,2.03852710839681));
#7079=CARTESIAN_POINT('Ctrl Pts',(14.1043988884374,-31.0361590434961,2.00920969898413));
#7080=CARTESIAN_POINT('Ctrl Pts',(14.1431387485305,-31.033001646773,1.97900561592663));
#7081=CARTESIAN_POINT('Ctrl Pts',(14.1810084262852,-31.0301755043672,1.94799199564959));
#7082=CARTESIAN_POINT('Ctrl Pts',(14.2374606145018,-31.0259625843616,1.90176010689422));
#7083=CARTESIAN_POINT('Ctrl Pts',(14.2926991654363,-31.0228311175415,1.85331739425799));
#7084=CARTESIAN_POINT('Ctrl Pts',(14.3464350150607,-31.0208199212765,1.80284481408892));
#7085=CARTESIAN_POINT('Ctrl Pts',(14.4000998043365,-31.0188113846198,1.75243897891727));
#7086=CARTESIAN_POINT('Ctrl Pts',(14.4522652453566,-31.0179202520598,1.70000899168618));
#7087=CARTESIAN_POINT('Ctrl Pts',(14.502665154571,-31.0181648931129,1.64577768116561));
#7088=CARTESIAN_POINT('Ctrl Pts',(14.5530682667356,-31.0184095497132,1.59154292420659));
#7089=CARTESIAN_POINT('Ctrl Pts',(14.6017050675006,-31.0197901594918,1.53550708982247));
#7090=CARTESIAN_POINT('Ctrl Pts',(14.6483399207647,-31.0223038005615,1.47792947798989));
#7091=CARTESIAN_POINT('Ctrl Pts',(14.6949634916526,-31.0248168335058,1.42036579591648));
#7092=CARTESIAN_POINT('Ctrl Pts',(14.7395856359476,-31.02846231646,1.3612616640622));
#7093=CARTESIAN_POINT('Ctrl Pts',(14.7820090211866,-31.0332160313446,1.30090464504866));
#7094=CARTESIAN_POINT('Ctrl Pts',(14.8244968863946,-31.037976971475,1.24045588845464));
#7095=CARTESIAN_POINT('Ctrl Pts',(14.8647789760217,-31.0438494224712,1.17875107963657));
#7096=CARTESIAN_POINT('Ctrl Pts',(14.9027011721154,-31.0507886274603,1.11609838715478));
#7097=CARTESIAN_POINT('Ctrl Pts',(14.9281399880451,-31.0554435572006,1.07406995853712));
#7098=CARTESIAN_POINT('Ctrl Pts',(14.9525177990215,-31.0605780934011,1.03161537789579));
#7099=CARTESIAN_POINT('Ctrl Pts',(14.975800076653,-31.0661739903831,0.988830267143717));
#7100=CARTESIAN_POINT('Ctrl Pts',(15.0105068815928,-31.074515773266,0.925050661183067));
#7101=CARTESIAN_POINT('Ctrl Pts',(15.0433058380794,-31.0843398123408,0.85996981368557));
#7102=CARTESIAN_POINT('Ctrl Pts',(15.0739990115275,-31.0956323113691,0.793867798863216));
#7103=CARTESIAN_POINT('Ctrl Pts',(15.1046515962884,-31.1069098771839,0.727853197419949));
#7104=CARTESIAN_POINT('Ctrl Pts',(15.1332035267178,-31.1196520113202,0.660820696335817));
#7105=CARTESIAN_POINT('Ctrl Pts',(15.1594929062039,-31.1338168732025,0.593075062136874));
#7106=CARTESIAN_POINT('Ctrl Pts',(15.1857839563985,-31.1479826352717,0.525325122655191));
#7107=CARTESIAN_POINT('Ctrl Pts',(15.2098118340435,-31.1635712134381,0.456862603465919));
#7108=CARTESIAN_POINT('Ctrl Pts',(15.2314557123161,-31.1805134006464,0.388009033183554));
#7109=CARTESIAN_POINT('Ctrl Pts',(15.2530943542826,-31.1974514890293,0.319172120653958));
#7110=CARTESIAN_POINT('Ctrl Pts',(15.2723499530455,-31.2157423538751,0.249945031380815));
#7111=CARTESIAN_POINT('Ctrl Pts',(15.2891468470745,-31.2352915303582,0.180655744947757));
#7112=CARTESIAN_POINT('Ctrl Pts',(15.3059692709664,-31.2548704199413,0.111261144641073));
#7113=CARTESIAN_POINT('Ctrl Pts',(15.3203254460599,-31.2757112046725,0.0418048433777034));
#7114=CARTESIAN_POINT('Ctrl Pts',(15.3321865776807,-31.2976967722504,-0.0273873077134898));
#7115=CARTESIAN_POINT('Ctrl Pts',(15.3401432145609,-31.3124450427708,-0.0738025098029384));
#7116=CARTESIAN_POINT('Ctrl Pts',(15.346978088765,-31.3277079982387,-0.120098937660215));
#7117=CARTESIAN_POINT('Ctrl Pts',(15.3526943843833,-31.3434456196644,-0.166181422977341));
#7118=CARTESIAN_POINT('Ctrl Pts',(15.3612156450668,-31.3669056335723,-0.234876412976922));
#7119=CARTESIAN_POINT('Ctrl Pts',(15.3675453741577,-31.3920116882092,-0.303705335324268));
#7120=CARTESIAN_POINT('Ctrl Pts',(15.3716049858294,-31.4186810812984,-0.372344470076017));
#7121=CARTESIAN_POINT('Ctrl Pts',(15.3756592290661,-31.4453152067524,-0.440892836359328));
#7122=CARTESIAN_POINT('Ctrl Pts',(15.3774491636308,-31.4735083864055,-0.509251242357308));
#7123=CARTESIAN_POINT('Ctrl Pts',(15.3769376406635,-31.503146756534,-0.577093346536008));
#7124=CARTESIAN_POINT('Ctrl Pts',(15.3764260851886,-31.5327870102016,-0.644939762127695));
#7125=CARTESIAN_POINT('Ctrl Pts',(15.3736127084781,-31.5638723937955,-0.712269124559153));
#7126=CARTESIAN_POINT('Ctrl Pts',(15.3685035059756,-31.596260479391,-0.778761359263442));
#7127=CARTESIAN_POINT('Ctrl Pts',(15.3633955395432,-31.6286407293327,-0.845237507492574));
#7128=CARTESIAN_POINT('Ctrl Pts',(15.355992925308,-31.6623227206288,-0.910876280138652));
#7129=CARTESIAN_POINT('Ctrl Pts',(15.3463448103112,-31.6971399301915,-0.975374241034996));
#7130=CARTESIAN_POINT('Ctrl Pts',(15.336682030993,-31.7320100589774,-1.03997023339446));
#7131=CARTESIAN_POINT('Ctrl Pts',(15.3247671072894,-31.768018469671,-1.10342135481207));
#7132=CARTESIAN_POINT('Ctrl Pts',(15.3106908011997,-31.804979023893,-1.16544861040279));
#7133=CARTESIAN_POINT('Ctrl Pts',(15.301248189841,-31.829772755068,-1.20705748594613));
#7134=CARTESIAN_POINT('Ctrl Pts',(15.2908338333953,-31.8549945584951,-1.2480261856948));
#7135=CARTESIAN_POINT('Ctrl Pts',(15.2794847232809,-31.8805848965145,-1.28827884419633));
#7136=CARTESIAN_POINT('Ctrl Pts',(15.2625666469132,-31.9187323185172,-1.34828333297744));
#7137=CARTESIAN_POINT('Ctrl Pts',(15.2436400707701,-31.9584201077799,-1.40722791797319));
#7138=CARTESIAN_POINT('Ctrl Pts',(15.2227503386142,-31.9994940112443,-1.46480935021377));
#7139=CARTESIAN_POINT('Ctrl Pts',(15.201888231064,-32.0405135985318,-1.5223146367026));
#7140=CARTESIAN_POINT('Ctrl Pts',(15.1790682259857,-32.082915333462,-1.57845972694411));
#7141=CARTESIAN_POINT('Ctrl Pts',(15.1543736752632,-32.1265157811743,-1.63296134033967));
#7142=CARTESIAN_POINT('Ctrl Pts',(15.1296775551844,-32.1701189997261,-1.68746641735158));
#7143=CARTESIAN_POINT('Ctrl Pts',(15.1031068324942,-32.2149206934165,-1.74032721705509));
#7144=CARTESIAN_POINT('Ctrl Pts',(15.0747812191856,-32.2607127800405,-1.79128851362422));
#7145=CARTESIAN_POINT('Ctrl Pts',(15.0464624586962,-32.3064937881792,-1.84223748112036));
#7146=CARTESIAN_POINT('Ctrl Pts',(15.016389950023,-32.3532642491317,-1.89128737321084));
#7147=CARTESIAN_POINT('Ctrl Pts',(14.9847160665489,-32.4007980420539,-1.93821939640007));
#7148=CARTESIAN_POINT('Ctrl Pts',(14.9529940414421,-32.4484040823342,-1.98522275230807));
#7149=CARTESIAN_POINT('Ctrl Pts',(14.9196661479882,-32.4967752768773,-2.03010142110661));
#7150=CARTESIAN_POINT('Ctrl Pts',(14.8849132585906,-32.5456734620382,-2.07267852251313));
#7151=CARTESIAN_POINT('Ctrl Pts',(14.8616004643044,-32.5784751470602,-2.10123992340946));
#7152=CARTESIAN_POINT('Ctrl Pts',(14.8376470050091,-32.6115137551623,-2.12876654161601));
#7153=CARTESIAN_POINT('Ctrl Pts',(14.8131130783409,-32.6447163505684,-2.15521684061908));
#7154=CARTESIAN_POINT('Ctrl Pts',(14.7765404448228,-32.6942113364327,-2.1946462032713));
#7155=CARTESIAN_POINT('Ctrl Pts',(14.7385728066074,-32.7448924880085,-2.2320317529486));
#7156=CARTESIAN_POINT('Ctrl Pts',(14.6993594721015,-32.7965455282222,-2.2671507738323));
#7157=CARTESIAN_POINT('Ctrl Pts',(14.6601979933537,-32.8481302623967,-2.30222335328281));
#7158=CARTESIAN_POINT('Ctrl Pts',(14.6197944052214,-32.9006838837365,-2.33503490407254));
#7159=CARTESIAN_POINT('Ctrl Pts',(14.5783244466735,-32.9539696176727,-2.36540131373483));
#7160=CARTESIAN_POINT('Ctrl Pts',(14.5368518526803,-33.007258737955,-2.39576965320397));
#7161=CARTESIAN_POINT('Ctrl Pts',(14.4943131261224,-33.0612795629769,-2.42369216050319));
#7162=CARTESIAN_POINT('Ctrl Pts',(14.450906066867,-33.115778926478,-2.44902900915247));
#7163=CARTESIAN_POINT('Ctrl Pts',(14.4075095090871,-33.1702651049412,-2.47435972805472));
#7164=CARTESIAN_POINT('Ctrl Pts',(14.3632454751571,-33.2252290468209,-2.4971058069034));
#7165=CARTESIAN_POINT('Ctrl Pts',(14.3183275373294,-33.2804092980893,-2.5171764296092));
#7166=CARTESIAN_POINT('Ctrl Pts',(14.2733413280232,-33.3356734186875,-2.53727755796941));
#7167=CARTESIAN_POINT('Ctrl Pts',(14.2276996951381,-33.3911539540059,-2.5546950033922));
#7168=CARTESIAN_POINT('Ctrl Pts',(14.1816263277413,-33.4465880201868,-2.56938903350673));
#7169=CARTESIAN_POINT('Ctrl Pts',(14.150719575675,-33.4837740787775,-2.57924602402564));
#7170=CARTESIAN_POINT('Ctrl Pts',(14.1196187266958,-33.5209392342376,-2.58787857636214));
#7171=CARTESIAN_POINT('Ctrl Pts',(14.0883919872725,-33.5580059268895,-2.59528770975726));
#7172=CARTESIAN_POINT('Ctrl Pts',(14.0418424025961,-33.6132611081907,-2.60633247743793));
#7173=CARTESIAN_POINT('Ctrl Pts',(13.9948202613369,-33.6691698795361,-2.61475432517952));
#7174=CARTESIAN_POINT('Ctrl Pts',(13.9475382801283,-33.7254813550954,-2.62045518191382));
#7175=CARTESIAN_POINT('Ctrl Pts',(13.900318824665,-33.7817183642961,-2.62614849982874));
#7176=CARTESIAN_POINT('Ctrl Pts',(13.8528406543396,-33.8383564975698,-2.62912778112532));
#7177=CARTESIAN_POINT('Ctrl Pts',(13.8053254831527,-33.8951324366506,-2.62934454720094));
#7178=CARTESIAN_POINT('Ctrl Pts',(13.7578072923433,-33.9519119838823,-2.62956132705218));
#7179=CARTESIAN_POINT('Ctrl Pts',(13.7102525630299,-34.0088287994454,-2.6270151469294));
#7180=CARTESIAN_POINT('Ctrl Pts',(13.6628860880188,-34.065614132699,-2.62170927404773));
#7181=CARTESIAN_POINT('Ctrl Pts',(13.6155310723855,-34.1223857278693,-2.61640468481661));
#7182=CARTESIAN_POINT('Ctrl Pts',(13.5683646880051,-34.1790253425627,-2.60834181054517));
#7183=CARTESIAN_POINT('Ctrl Pts',(13.5216075573401,-34.2352674523107,-2.59757579979065));
#7184=CARTESIAN_POINT('Ctrl Pts',(13.4747793597782,-34.2915950453243,-2.58679342560735));
#7185=CARTESIAN_POINT('Ctrl Pts',(13.4283621048929,-34.3475233862133,-2.5732999089776));
#7186=CARTESIAN_POINT('Ctrl Pts',(13.3825665243094,-34.402797072103,-2.5572005349256));
#7187=CARTESIAN_POINT('Ctrl Pts',(13.3518461160827,-34.4398755450274,-2.54640081720679));
#7188=CARTESIAN_POINT('Ctrl Pts',(13.32140521877,-34.476659677215,-2.53442952081174));
#7189=CARTESIAN_POINT('Ctrl Pts',(13.291303264039,-34.5130769751218,-2.52133001886304));
#7190=CARTESIAN_POINT('Ctrl Pts',(13.2464303917327,-34.5673641060844,-2.50180263987811));
#7191=CARTESIAN_POINT('Ctrl Pts',(13.2021336618323,-34.6216993604479,-2.47959273545193));
#7192=CARTESIAN_POINT('Ctrl Pts',(13.1586360840035,-34.675825909697,-2.45474630344456));
#7193=CARTESIAN_POINT('Ctrl Pts',(13.1151960274206,-34.7298808819363,-2.42993272838686));
#7194=CARTESIAN_POINT('Ctrl Pts',(13.0725534835316,-34.783727164985,-2.40248965699108));
#7195=CARTESIAN_POINT('Ctrl Pts',(13.0309206233962,-34.8371069501965,-2.37251384630043));
#7196=CARTESIAN_POINT('Ctrl Pts',(12.9892851174628,-34.8904901277314,-2.34253613062566));
#7197=CARTESIAN_POINT('Ctrl Pts',(12.9486598673696,-34.9434062066014,-2.31002556528109));
#7198=CARTESIAN_POINT('Ctrl Pts',(12.9092402176435,-34.9956034381375,-2.27512786406503));
#7199=CARTESIAN_POINT('Ctrl Pts',(12.869830104718,-35.0477880415911,-2.24023860565402));
#7200=CARTESIAN_POINT('Ctrl Pts',(12.8316253907942,-35.0992536334345,-2.20296372939623));
#7201=CARTESIAN_POINT('Ctrl Pts',(12.794798203505,-35.1497626877019,-2.16349342564734));
#7202=CARTESIAN_POINT('Ctrl Pts',(12.7579150419963,-35.200348511473,-2.12396313036471));
#7203=CARTESIAN_POINT('Ctrl Pts',(12.7224139039918,-35.2499744293424,-2.0822312081381));
#7204=CARTESIAN_POINT('Ctrl Pts',(12.6884393559493,-35.2984232389124,-2.0385271083965));
#7205=CARTESIAN_POINT('Ctrl Pts',(12.6656486854982,-35.3309234755976,-2.00920969898392));
#7206=CARTESIAN_POINT('Ctrl Pts',(12.6435443696797,-35.3628944802155,-1.97900561592653));
#7207=CARTESIAN_POINT('Ctrl Pts',(12.6221620196843,-35.3942775119812,-1.94799199564959));
#7208=CARTESIAN_POINT('Ctrl Pts',(12.5902874298269,-35.4410600810735,-1.90176010689391));
#7209=CARTESIAN_POINT('Ctrl Pts',(12.559956224542,-35.4873323360413,-1.85331739425731));
#7210=CARTESIAN_POINT('Ctrl Pts',(12.5313465526722,-35.5328633487778,-1.80284481408786));
#7211=CARTESIAN_POINT('Ctrl Pts',(12.5027747142649,-35.5783341512515,-1.7524389789157));
#7212=CARTESIAN_POINT('Ctrl Pts',(12.4759202503196,-35.6230651820949,-1.70000899168406));
#7213=CARTESIAN_POINT('Ctrl Pts',(12.450932161079,-35.66683510435,-1.64577768116292));
#7214=CARTESIAN_POINT('Ctrl Pts',(12.4259424838277,-35.7106078082145,-1.59154292420375));
#7215=CARTESIAN_POINT('Ctrl Pts',(12.4028197265862,-35.7534188181251,-1.53550708981947));
#7216=CARTESIAN_POINT('Ctrl Pts',(12.3816791769766,-35.7950626062884,-1.47792947798673));
#7217=CARTESIAN_POINT('Ctrl Pts',(12.3605437419031,-35.8366963195644,-1.42036579591363));
#7218=CARTESIAN_POINT('Ctrl Pts',(12.3413897506033,-35.877162971572,-1.3612616640597));
#7219=CARTESIAN_POINT('Ctrl Pts',(12.3242948958363,-35.9162795583455,-1.30090464504652));
#7220=CARTESIAN_POINT('Ctrl Pts',(12.3071740583312,-35.9554555990333,-1.24045588845259));
#7221=CARTESIAN_POINT('Ctrl Pts',(12.2921187052629,-35.9932771374658,-1.17875107963462));
#7222=CARTESIAN_POINT('Ctrl Pts',(12.2791671350188,-36.0295883251447,-1.11609838715294));
#7223=CARTESIAN_POINT('Ctrl Pts',(12.270479014462,-36.0539464508519,-1.07406995853587));
#7224=CARTESIAN_POINT('Ctrl Pts',(12.2627367477602,-36.0776255225459,-1.03161537789517));
#7225=CARTESIAN_POINT('Ctrl Pts',(12.255941797888,-36.1005865149234,-0.988830267143708));
#7226=CARTESIAN_POINT('Ctrl Pts',(12.2458125913075,-36.1348143811267,-0.925050661183478));
#7227=CARTESIAN_POINT('Ctrl Pts',(12.2379209804709,-36.1681311301989,-0.859969813686402));
#7228=CARTESIAN_POINT('Ctrl Pts',(12.2323539847775,-36.2003584476417,-0.793867798864489));
#7229=CARTESIAN_POINT('Ctrl Pts',(12.2267943508855,-36.2325431476436,-0.727853197421361));
#7230=CARTESIAN_POINT('Ctrl Pts',(12.2235533975312,-36.2636409117907,-0.660820696337379));
#7231=CARTESIAN_POINT('Ctrl Pts',(12.2226758380193,-36.2934906132165,-0.593075062138574));
#7232=CARTESIAN_POINT('Ctrl Pts',(12.2217982227379,-36.3233422116119,-0.52532512265681));
#7233=CARTESIAN_POINT('Ctrl Pts',(12.2232843886163,-36.3519452531347,-0.456862603467453));
#7234=CARTESIAN_POINT('Ctrl Pts',(12.2271348139981,-36.3791604951594,-0.388009033184998));
#7235=CARTESIAN_POINT('Ctrl Pts',(12.2309843078459,-36.406369152997,-0.319172120656019));
#7236=CARTESIAN_POINT('Ctrl Pts',(12.237196862078,-36.4321904231135,-0.249945031383509));
#7237=CARTESIAN_POINT('Ctrl Pts',(12.2457284985207,-36.4565115482887,-0.18065574495107));
#7238=CARTESIAN_POINT('Ctrl Pts',(12.2542731023316,-36.4808696395237,-0.111261144644779));
#7239=CARTESIAN_POINT('Ctrl Pts',(12.2651436637966,-36.5037228442214,-0.0418048433818011));
#7240=CARTESIAN_POINT('Ctrl Pts',(12.2782531580251,-36.5249876693116,0.0273873077090091));
#7241=CARTESIAN_POINT('Ctrl Pts',(12.2870472165178,-36.5392524542392,0.0738025097999603));
#7242=CARTESIAN_POINT('Ctrl Pts',(12.2968478865881,-36.552803106666,0.120098937658729));
#7243=CARTESIAN_POINT('Ctrl Pts',(12.3076189187291,-36.5656223746002,0.16618142297734));
#7244=CARTESIAN_POINT('Ctrl Pts',(12.3236752564048,-36.5847320097785,0.23487641297725));
#7245=CARTESIAN_POINT('Ctrl Pts',(12.3422528729638,-36.6027667432888,0.303705335324935));
#7246=CARTESIAN_POINT('Ctrl Pts',(12.3633194390469,-36.6196171666707,0.372344470077012));
#7247=CARTESIAN_POINT('Ctrl Pts',(12.3843581466792,-36.6364453070337,0.440892836359892));
#7248=CARTESIAN_POINT('Ctrl Pts',(12.4078791891897,-36.6520920256643,0.50925124235744));
#7249=CARTESIAN_POINT('Ctrl Pts',(12.4338025321312,-36.6664682188442,0.577093346535715));
#7250=CARTESIAN_POINT('Ctrl Pts',(12.4597275225194,-36.6808453256412,0.644939762127416));
#7251=CARTESIAN_POINT('Ctrl Pts',(12.4880549427534,-36.6939515617364,0.712269124558878));
#7252=CARTESIAN_POINT('Ctrl Pts',(12.5186584489103,-36.705720905374,0.77876135926318));
#7253=CARTESIAN_POINT('Ctrl Pts',(12.5492545511566,-36.7174874016526,0.845237507491614));
#7254=CARTESIAN_POINT('Ctrl Pts',(12.5821253183863,-36.7279175453184,0.910876280137029));
#7255=CARTESIAN_POINT('Ctrl Pts',(12.6171019638544,-36.7369706374139,0.975374241032723));
#7256=CARTESIAN_POINT('Ctrl Pts',(12.6521317708754,-36.7460374894462,1.03997023339245));
#7257=CARTESIAN_POINT('Ctrl Pts',(12.6892734311378,-36.7537230681815,1.10342135481031));
#7258=CARTESIAN_POINT('Ctrl Pts',(12.7283203630771,-36.7600129066275,1.16544861040129));
#7259=CARTESIAN_POINT('Ctrl Pts',(12.7545136698089,-36.7642322309003,1.20705748594514));
#7260=CARTESIAN_POINT('Ctrl Pts',(12.7815635705291,-36.7678240353679,1.24802618569432));
#7261=CARTESIAN_POINT('Ctrl Pts',(12.8094000084029,-36.7707905867082,1.28827884419634));
#7262=CARTESIAN_POINT('Ctrl Pts',(12.8508956831299,-36.775212813792,1.34828333297722));
#7263=CARTESIAN_POINT('Ctrl Pts',(12.8947296049227,-36.7786658126767,1.40722791797275));
#7264=CARTESIAN_POINT('Ctrl Pts',(12.9407455148333,-36.7811117256837,1.46480935021313));
#7265=CARTESIAN_POINT('Ctrl Pts',(12.9867005732529,-36.7835544042125,1.52231463670294));
#7266=CARTESIAN_POINT('Ctrl Pts',(13.0348315554069,-36.7849925675654,1.57845972694538));
#7267=CARTESIAN_POINT('Ctrl Pts',(13.0849379261043,-36.7854066831607,1.63296134034182));
#7268=CARTESIAN_POINT('Ctrl Pts',(13.1350474810965,-36.7858208250734,1.68746641735378));
#7269=CARTESIAN_POINT('Ctrl Pts',(13.1871322473101,-36.785210751072,1.74032721705733));
#7270=CARTESIAN_POINT('Ctrl Pts',(13.2409521642733,-36.7835760936809,1.79128851362649));
#7271=CARTESIAN_POINT('Ctrl Pts',(13.2947590605769,-36.7819418317627,1.84223748112254));
#7272=CARTESIAN_POINT('Ctrl Pts',(13.3502997222452,-36.7792835057724,1.89128737321292));
#7273=CARTESIAN_POINT('Ctrl Pts',(13.4073021361911,-36.7756200145084,1.93821939640206));
#7274=CARTESIAN_POINT('Ctrl Pts',(13.4643911890004,-36.7719509550466,1.98522275230973));
#7275=CARTESIAN_POINT('Ctrl Pts',(13.5229458190128,-36.7672737499325,2.03010142110795));
#7276=CARTESIAN_POINT('Ctrl Pts',(13.5826693342596,-36.7616259574397,2.07267852251418));
#7277=CARTESIAN_POINT('Ctrl Pts',(13.6227328239182,-36.7578373278657,2.10123992341013));
#7278=CARTESIAN_POINT('Ctrl Pts',(13.6633218274875,-36.7536123276585,2.12876654161633));
#7279=CARTESIAN_POINT('Ctrl Pts',(13.7043430819143,-36.7489666216124,2.15521684061907));
#7280=CARTESIAN_POINT('Ctrl Pts',(13.7654933137917,-36.7420412848346,2.19464620327122));
#7281=CARTESIAN_POINT('Ctrl Pts',(13.8283682976569,-36.7345009214063,2.23203175294843));
#7282=CARTESIAN_POINT('Ctrl Pts',(13.8927078099174,-36.7263676976639,2.26715077383206));
#7283=CARTESIAN_POINT('Ctrl Pts',(13.9569622395338,-36.7182452293059,2.30222335328249));
#7284=CARTESIAN_POINT('Ctrl Pts',(14.0226768047409,-36.7095315062492,2.33503490407216));
#7285=CARTESIAN_POINT('Ctrl Pts',(14.0895585832627,-36.7002603356209,2.36540131373439));
#7286=CARTESIAN_POINT('Ctrl Pts',(14.1564446121692,-36.6909885758032,2.39576965320358));
#7287=CARTESIAN_POINT('Ctrl Pts',(14.2244973822506,-36.6811593704703,2.42369216050285));
#7288=CARTESIAN_POINT('Ctrl Pts',(14.2933987451604,-36.6708174362021,2.44902900915218));
#7289=CARTESIAN_POINT('Ctrl Pts',(14.3622834387544,-36.6604780039595,2.47435972805441));
#7290=CARTESIAN_POINT('Ctrl Pts',(14.4320156256792,-36.649626197042,2.49710580690308));
#7291=CARTESIAN_POINT('Ctrl Pts',(14.5022620939786,-36.6383162474319,2.51717642960887));
#7292=CARTESIAN_POINT('Ctrl Pts',(14.5726153309875,-36.6269891076519,2.53727755796908));
#7293=CARTESIAN_POINT('Ctrl Pts',(14.6434837004311,-36.6152025617624,2.55469500339187));
#7294=CARTESIAN_POINT('Ctrl Pts',(14.7145276936772,-36.6030188882494,2.5693890335064));
#7295=CARTESIAN_POINT('Ctrl Pts',(14.762185141117,-36.5948458851067,2.57924602402545));
#7296=CARTESIAN_POINT('Ctrl Pts',(14.8099215343711,-36.5864943375414,2.58787857636205));
#7297=CARTESIAN_POINT('Ctrl Pts',(14.8576356015541,-36.5779845342494,2.59528770975725));
#7298=CARTESIAN_POINT('Ctrl Pts',(14.9287627845898,-36.5652990020346,2.60633247743792));
#7299=CARTESIAN_POINT('Ctrl Pts',(15.0006922714988,-36.5525310188365,2.6147543251795));
#7300=CARTESIAN_POINT('Ctrl Pts',(15.0731004304621,-36.5397393597483,2.62045518191379));
#7301=CARTESIAN_POINT('Ctrl Pts',(15.145412836794,-36.5269646163646,2.6261484998287));
#7302=CARTESIAN_POINT('Ctrl Pts',(15.2182019841943,-36.5141663813745,2.62912778112528));
#7303=CARTESIAN_POINT('Ctrl Pts',(15.291128975355,-36.501405005602,2.62934454720092));
#7304=CARTESIAN_POINT('Ctrl Pts',(15.3640606010775,-36.488642818835,2.62956132705221));
#7305=CARTESIAN_POINT('Ctrl Pts',(15.4371293739142,-36.4759176229611,2.62701514692947));
#7306=CARTESIAN_POINT('Ctrl Pts',(15.5099901525795,-36.4632897189407,2.62170927404787));
#7307=CARTESIAN_POINT('Ctrl Pts',(15.5828333040276,-36.4506648699906,2.61640468481675));
#7308=CARTESIAN_POINT('Ctrl Pts',(15.6554678414036,-36.4381373902591,2.60834181054526));
#7309=CARTESIAN_POINT('Ctrl Pts',(15.7275535025409,-36.425765582169,2.59757579979065));
#7310=CARTESIAN_POINT('Ctrl Pts',(15.7997487278054,-36.4133749699738,2.58679342560739));
#7311=CARTESIAN_POINT('Ctrl Pts',(15.8713927192492,-36.4011406185138,2.57329990897769));
#7312=CARTESIAN_POINT('Ctrl Pts',(15.9421589256821,-36.3891173252922,2.55720053492575));
#7313=CARTESIAN_POINT('Ctrl Pts',(15.9896300292816,-36.3810519078155,2.54640081720691));
#7314=CARTESIAN_POINT('Ctrl Pts',(16.0367064708689,-36.3730813835224,2.53442952081181));
#7315=CARTESIAN_POINT('Ctrl Pts',(16.0832957533591,-36.3652209749752,2.52133001886304));
#7316=CARTESIAN_POINT('Ctrl Pts',(16.1527462240253,-36.3535034930984,2.50180263987787));
#7317=CARTESIAN_POINT('Ctrl Pts',(16.2219502995763,-36.3423090268816,2.47959273545136));
#7318=CARTESIAN_POINT('Ctrl Pts',(16.2905740551604,-36.3317022941032,2.4547463034436));
#7319=CARTESIAN_POINT('Ctrl Pts',(16.3591070626129,-36.3211095876801,2.42993272838552));
#7320=CARTESIAN_POINT('Ctrl Pts',(16.4270605835777,-36.3111032029145,2.40248965698929));
#7321=CARTESIAN_POINT('Ctrl Pts',(16.494105263688,-36.3017379810107,2.37251384629813));
#7322=CARTESIAN_POINT('Ctrl Pts',(16.5611542045347,-36.2923721639404,2.34253613062317));
#7323=CARTESIAN_POINT('Ctrl Pts',(16.6272934981514,-36.2836477047596,2.31002556527841));
#7324=CARTESIAN_POINT('Ctrl Pts',(16.692207451532,-36.2756079024566,2.27512786406214));
#7325=CARTESIAN_POINT('Ctrl Pts',(16.7571057002714,-36.267570045224,2.24023860565128));
#7326=CARTESIAN_POINT('Ctrl Pts',(16.8207785671899,-36.2602165883435,2.2029637293937));
#7327=CARTESIAN_POINT('Ctrl Pts',(16.8829342849506,-36.2535778357349,2.16349342564505));
#7328=CARTESIAN_POINT('Ctrl Pts',(16.9451844741622,-36.2469289927821,2.12396313036229));
#7329=CARTESIAN_POINT('Ctrl Pts',(17.0059123487253,-36.2409970643416,2.08223120813556));
#7330=CARTESIAN_POINT('Ctrl Pts',(17.0648575226173,-36.2357986474397,2.03852710839383));
#7331=CARTESIAN_POINT('Ctrl Pts',(17.10439888844,-36.2323114662026,2.00920969898208));
#7332=CARTESIAN_POINT('Ctrl Pts',(17.1431387485318,-36.2291540694795,1.97900561592558));
#7333=CARTESIAN_POINT('Ctrl Pts',(17.1810084262852,-36.2263279270739,1.94799199564959));
#7334=CARTESIAN_POINT('Ctrl Pts',(17.2374606145019,-36.2221150070683,1.90176010689407));
#7335=CARTESIAN_POINT('Ctrl Pts',(17.2926991654366,-36.2189835402481,1.85331739425768));
#7336=CARTESIAN_POINT('Ctrl Pts',(17.3464350150612,-36.2169723439831,1.80284481408843));
#7337=CARTESIAN_POINT('Ctrl Pts',(17.4000998043377,-36.2149638073264,1.75243897891608));
#7338=CARTESIAN_POINT('Ctrl Pts',(17.4522652453585,-36.2140726747664,1.70000899168421));
#7339=CARTESIAN_POINT('Ctrl Pts',(17.5026651545736,-36.2143173158196,1.64577768116285));
#7340=CARTESIAN_POINT('Ctrl Pts',(17.553068266738,-36.2145619724199,1.59154292420388));
#7341=CARTESIAN_POINT('Ctrl Pts',(17.6017050675028,-36.2159425821985,1.53550708981983));
#7342=CARTESIAN_POINT('Ctrl Pts',(17.6483399207667,-36.2184562232683,1.47792947798732));
#7343=CARTESIAN_POINT('Ctrl Pts',(17.6949634916545,-36.2209692562126,1.42036579591399));
#7344=CARTESIAN_POINT('Ctrl Pts',(17.7395856359494,-36.2246147391669,1.36126166405979));
#7345=CARTESIAN_POINT('Ctrl Pts',(17.7820090211882,-36.2293684540514,1.30090464504635));
#7346=CARTESIAN_POINT('Ctrl Pts',(17.824496886396,-36.2341293941818,1.24045588845241));
#7347=CARTESIAN_POINT('Ctrl Pts',(17.864778976023,-36.240001845178,1.17875107963445));
#7348=CARTESIAN_POINT('Ctrl Pts',(17.9027011721166,-36.2469410501671,1.11609838715275));
#7349=CARTESIAN_POINT('Ctrl Pts',(17.9281399880459,-36.2515959799074,1.07406995853575));
#7350=CARTESIAN_POINT('Ctrl Pts',(17.9525177990218,-36.2567305161078,1.0316153778951));
#7351=CARTESIAN_POINT('Ctrl Pts',(17.9758000766529,-36.2623264130898,0.988830267143709));
#7352=CARTESIAN_POINT('Ctrl Pts',(18.0105068815927,-36.2706681959726,0.925050661183277));
#7353=CARTESIAN_POINT('Ctrl Pts',(18.0433058380791,-36.2804922350474,0.859969813686007));
#7354=CARTESIAN_POINT('Ctrl Pts',(18.0739990115272,-36.2917847340756,0.793867798863887));
#7355=CARTESIAN_POINT('Ctrl Pts',(18.1046515962876,-36.3030622998902,0.727853197421574));
#7356=CARTESIAN_POINT('Ctrl Pts',(18.1332035267167,-36.3158044340263,0.660820696338441));
#7357=CARTESIAN_POINT('Ctrl Pts',(18.1594929062024,-36.3299692959084,0.593075062140492));
#7358=CARTESIAN_POINT('Ctrl Pts',(18.1857839563971,-36.3441350579776,0.5253251226589));
#7359=CARTESIAN_POINT('Ctrl Pts',(18.2098118340421,-36.3597236361438,0.456862603469714));
#7360=CARTESIAN_POINT('Ctrl Pts',(18.2314557123148,-36.3766658233521,0.38800903318743));
#7361=CARTESIAN_POINT('Ctrl Pts',(18.2530943542811,-36.3936039117347,0.319172120658737));
#7362=CARTESIAN_POINT('Ctrl Pts',(18.2723499530439,-36.4118947765802,0.249945031386501));
#7363=CARTESIAN_POINT('Ctrl Pts',(18.2891468470729,-36.431443953063,0.180655744954341));
#7364=CARTESIAN_POINT('Ctrl Pts',(18.3059692709647,-36.4510228426459,0.111261144648359));
#7365=CARTESIAN_POINT('Ctrl Pts',(18.3203254460583,-36.4718636273767,0.0418048433856814));
#7366=CARTESIAN_POINT('Ctrl Pts',(18.3321865776792,-36.4938491949543,-0.027387307704834));
#7367=CARTESIAN_POINT('Ctrl Pts',(18.34014321456,-36.5085974654755,-0.0738025097971843));
#7368=CARTESIAN_POINT('Ctrl Pts',(18.3469780887646,-36.5238604209444,-0.12009893765735));
#7369=CARTESIAN_POINT('Ctrl Pts',(18.3526943843832,-36.539598042371,-0.166181422977344));
#7370=CARTESIAN_POINT('Ctrl Pts',(18.3612156450669,-36.5630580562793,-0.234876412977713));
#7371=CARTESIAN_POINT('Ctrl Pts',(18.3675453741578,-36.5881641109164,-0.303705335325853));
#7372=CARTESIAN_POINT('Ctrl Pts',(18.3716049858295,-36.614833504006,-0.372344470078386));
#7373=CARTESIAN_POINT('Ctrl Pts',(18.3756592290661,-36.6414676294599,-0.440892836361369));
#7374=CARTESIAN_POINT('Ctrl Pts',(18.3774491636308,-36.6696608091128,-0.509251242359004));
#7375=CARTESIAN_POINT('Ctrl Pts',(18.3769376406635,-36.6992991792413,-0.577093346537381));
#7376=CARTESIAN_POINT('Ctrl Pts',(18.3764260851885,-36.728939432909,-0.644939762129239));
#7377=CARTESIAN_POINT('Ctrl Pts',(18.3736127084779,-36.7600248165029,-0.712269124560869));
#7378=CARTESIAN_POINT('Ctrl Pts',(18.3685035059754,-36.7924129020986,-0.778761359265312));
#7379=CARTESIAN_POINT('Ctrl Pts',(18.3633955395429,-36.8247931520403,-0.845237507494451));
#7380=CARTESIAN_POINT('Ctrl Pts',(18.3559929253077,-36.8584751433364,-0.910876280140545));
#7381=CARTESIAN_POINT('Ctrl Pts',(18.3463448103109,-36.8932923528991,-0.975374241036891));
#7382=CARTESIAN_POINT('Ctrl Pts',(18.3366820309926,-36.9281624816852,-1.03997023339647));
#7383=CARTESIAN_POINT('Ctrl Pts',(18.324767107289,-36.9641708923788,-1.10342135481419));
#7384=CARTESIAN_POINT('Ctrl Pts',(18.3106908011992,-37.001131446601,-1.16544861040502));
#7385=CARTESIAN_POINT('Ctrl Pts',(18.3012481898405,-37.0259251777756,-1.20705748594759));
#7386=CARTESIAN_POINT('Ctrl Pts',(18.2908338333951,-37.0511469812022,-1.24802618569552));
#7387=CARTESIAN_POINT('Ctrl Pts',(18.2794847232809,-37.0767373192211,-1.28827884419634));
#7388=CARTESIAN_POINT('Ctrl Pts',(18.2625666469133,-37.1148847412236,-1.34828333297701));
#7389=CARTESIAN_POINT('Ctrl Pts',(18.2436400707704,-37.154572530486,-1.40722791797235));
#7390=CARTESIAN_POINT('Ctrl Pts',(18.2227503386146,-37.1956464339501,-1.46480935021252));
#7391=CARTESIAN_POINT('Ctrl Pts',(18.2018882310642,-37.2366660212381,-1.52231463670205));
#7392=CARTESIAN_POINT('Ctrl Pts',(18.1790682259857,-37.2790677561687,-1.57845972694423));
#7393=CARTESIAN_POINT('Ctrl Pts',(18.1543736752628,-37.3226682038816,-1.63296134034042));
#7394=CARTESIAN_POINT('Ctrl Pts',(18.129677555184,-37.3662714224335,-1.68746641735244));
#7395=CARTESIAN_POINT('Ctrl Pts',(18.1031068324937,-37.411073116124,-1.74032721705606));
#7396=CARTESIAN_POINT('Ctrl Pts',(18.074781219185,-37.4568652027481,-1.79128851362529));
#7397=CARTESIAN_POINT('Ctrl Pts',(18.0464624586957,-37.5026462108866,-1.84223748112121));
#7398=CARTESIAN_POINT('Ctrl Pts',(18.0163899500225,-37.549416671839,-1.89128737321147));
#7399=CARTESIAN_POINT('Ctrl Pts',(17.9847160665486,-37.596950464761,-1.93821939640052));
#7400=CARTESIAN_POINT('Ctrl Pts',(17.952994041442,-37.644556505041,-1.98522275230822));
#7401=CARTESIAN_POINT('Ctrl Pts',(17.9196661479882,-37.6929276995838,-2.03010142110648));
#7402=CARTESIAN_POINT('Ctrl Pts',(17.8849132585909,-37.7418258847445,-2.07267852251276));
#7403=CARTESIAN_POINT('Ctrl Pts',(17.8616004643046,-37.7746275697666,-2.10123992340922));
#7404=CARTESIAN_POINT('Ctrl Pts',(17.8376470050092,-37.8076661778688,-2.12876654161589));
#7405=CARTESIAN_POINT('Ctrl Pts',(17.8131130783409,-37.8408687732751,-2.15521684061908));
#7406=CARTESIAN_POINT('Ctrl Pts',(17.7765404448226,-37.8903637591396,-2.19464620327149));
#7407=CARTESIAN_POINT('Ctrl Pts',(17.738572806607,-37.9410449107156,-2.23203175294895));
#7408=CARTESIAN_POINT('Ctrl Pts',(17.6993594721009,-37.9926979509295,-2.26715077383279));
#7409=CARTESIAN_POINT('Ctrl Pts',(17.660197993353,-38.0442826851043,-2.30222335328343));
#7410=CARTESIAN_POINT('Ctrl Pts',(17.6197944052205,-38.0968363064444,-2.33503490407327));
#7411=CARTESIAN_POINT('Ctrl Pts',(17.5783244466724,-38.1501220403808,-2.36540131373564));
#7412=CARTESIAN_POINT('Ctrl Pts',(17.536851852679,-38.2034111606634,-2.39576965320488));
#7413=CARTESIAN_POINT('Ctrl Pts',(17.4943131261208,-38.2574319856855,-2.42369216050416));
#7414=CARTESIAN_POINT('Ctrl Pts',(17.4509060668652,-38.3119313491869,-2.44902900915349));
#7415=CARTESIAN_POINT('Ctrl Pts',(17.4075095090855,-38.3664175276498,-2.47435972805555));
#7416=CARTESIAN_POINT('Ctrl Pts',(17.3632454751557,-38.4213814695292,-2.49710580690407));
#7417=CARTESIAN_POINT('Ctrl Pts',(17.3183275373282,-38.4765617207974,-2.51717642960973));
#7418=CARTESIAN_POINT('Ctrl Pts',(17.273341328022,-38.5318258413957,-2.53727755796989));
#7419=CARTESIAN_POINT('Ctrl Pts',(17.2276996951368,-38.587306376714,-2.55469500339263));
#7420=CARTESIAN_POINT('Ctrl Pts',(17.1816263277401,-38.6427404428949,-2.56938903350711));
#7421=CARTESIAN_POINT('Ctrl Pts',(17.1507195756741,-38.6799265014851,-2.57924602402586));
#7422=CARTESIAN_POINT('Ctrl Pts',(17.1196187266954,-38.7170916569447,-2.58787857636224));
#7423=CARTESIAN_POINT('Ctrl Pts',(17.0883919872725,-38.7541583495962,-2.59528770975726));
#7424=CARTESIAN_POINT('Ctrl Pts',(17.0418424025962,-38.8094135308972,-2.6063324774379));
#7425=CARTESIAN_POINT('Ctrl Pts',(16.9948202613371,-38.8653223022424,-2.61475432517947));
#7426=CARTESIAN_POINT('Ctrl Pts',(16.9475382801287,-38.9216337778016,-2.62045518191377));
#7427=CARTESIAN_POINT('Ctrl Pts',(16.9003188246654,-38.9778707870022,-2.6261484998287));
#7428=CARTESIAN_POINT('Ctrl Pts',(16.8528406543402,-39.0345089202757,-2.62912778112529));
#7429=CARTESIAN_POINT('Ctrl Pts',(16.8053254831534,-39.0912848593564,-2.62934454720093));
#7430=CARTESIAN_POINT('Ctrl Pts',(16.7578072923443,-39.1480644065877,-2.62956132705221));
#7431=CARTESIAN_POINT('Ctrl Pts',(16.7102525630312,-39.2049812221505,-2.62701514692948));
#7432=CARTESIAN_POINT('Ctrl Pts',(16.6628860880204,-39.2617665554037,-2.62170927404791));
#7433=CARTESIAN_POINT('Ctrl Pts',(16.615531072387,-39.3185381505741,-2.61640468481683));
#7434=CARTESIAN_POINT('Ctrl Pts',(16.5683646880065,-39.3751777652676,-2.60834181054544));
#7435=CARTESIAN_POINT('Ctrl Pts',(16.5216075573414,-39.4314198750157,-2.59757579979095));
#7436=CARTESIAN_POINT('Ctrl Pts',(16.4747793597799,-39.4877474680289,-2.58679342560781));
#7437=CARTESIAN_POINT('Ctrl Pts',(16.428362104895,-39.5436758089174,-2.57329990897825));
#7438=CARTESIAN_POINT('Ctrl Pts',(16.3825665243119,-39.5989494948066,-2.55720053492649));
#7439=CARTESIAN_POINT('Ctrl Pts',(16.3518461160844,-39.636027967732,-2.54640081720745));
#7440=CARTESIAN_POINT('Ctrl Pts',(16.3214052187708,-39.6728120999206,-2.5344295208121));
#7441=CARTESIAN_POINT('Ctrl Pts',(16.2913032640389,-39.7092293978285,-2.52133001886304));
#7442=CARTESIAN_POINT('Ctrl Pts',(16.2464303917323,-39.7635165287916,-2.50180263987793));
#7443=CARTESIAN_POINT('Ctrl Pts',(16.2021336618314,-39.8178517831556,-2.47959273545151));
#7444=CARTESIAN_POINT('Ctrl Pts',(16.1586360840022,-39.8719783324052,-2.45474630344385));
#7445=CARTESIAN_POINT('Ctrl Pts',(16.115196027419,-39.926033304645,-2.4299327283859));
#7446=CARTESIAN_POINT('Ctrl Pts',(16.0725534835297,-39.979879587694,-2.40248965698983));
#7447=CARTESIAN_POINT('Ctrl Pts',(16.0309206233939,-40.033259372906,-2.37251384629885));
#7448=CARTESIAN_POINT('Ctrl Pts',(15.9892851174606,-40.086642550441,-2.34253613062394));
#7449=CARTESIAN_POINT('Ctrl Pts',(15.9486598673673,-40.139558629311,-2.31002556527922));
#7450=CARTESIAN_POINT('Ctrl Pts',(15.9092402176412,-40.1917558608472,-2.27512786406301));
#7451=CARTESIAN_POINT('Ctrl Pts',(15.8698301047161,-40.2439404643002,-2.24023860565226));
#7452=CARTESIAN_POINT('Ctrl Pts',(15.8316253907928,-40.295406056143,-2.2029637293948));
#7453=CARTESIAN_POINT('Ctrl Pts',(15.794798203504,-40.3459151104098,-2.16349342564628));
#7454=CARTESIAN_POINT('Ctrl Pts',(15.7579150419953,-40.396500934181,-2.12396313036366));
#7455=CARTESIAN_POINT('Ctrl Pts',(15.722413903991,-40.4461268520502,-2.08223120813708));
#7456=CARTESIAN_POINT('Ctrl Pts',(15.6884393559485,-40.4945756616201,-2.03852710839551));
#7457=CARTESIAN_POINT('Ctrl Pts',(15.6656486854977,-40.5270758983049,-2.00920969898324));
#7458=CARTESIAN_POINT('Ctrl Pts',(15.6435443696794,-40.5590469029225,-1.97900561592617));
#7459=CARTESIAN_POINT('Ctrl Pts',(15.6221620196843,-40.5904299346879,-1.94799199564958));
#7460=CARTESIAN_POINT('Ctrl Pts',(15.5902874298272,-40.6372125037797,-1.90176010689442));
#7461=CARTESIAN_POINT('Ctrl Pts',(15.5599562245427,-40.6834847587469,-1.8533173942584));
#7462=CARTESIAN_POINT('Ctrl Pts',(15.5313465526731,-40.729015771483,-1.80284481408956));
#7463=CARTESIAN_POINT('Ctrl Pts',(15.5027747142659,-40.7744865739564,-1.75243897891762));
#7464=CARTESIAN_POINT('Ctrl Pts',(15.4759202503206,-40.8192176047997,-1.70000899168622));
#7465=CARTESIAN_POINT('Ctrl Pts',(15.4509321610801,-40.8629875270547,-1.64577768116532));
#7466=CARTESIAN_POINT('Ctrl Pts',(15.4259424838289,-40.906760230919,-1.59154292420647));
#7467=CARTESIAN_POINT('Ctrl Pts',(15.4028197265874,-40.9495712408294,-1.53550708982251));
#7468=CARTESIAN_POINT('Ctrl Pts',(15.3816791769778,-40.9912150289926,-1.47792947799012));
#7469=CARTESIAN_POINT('Ctrl Pts',(15.3605437419042,-41.0328487422688,-1.42036579591683));
#7470=CARTESIAN_POINT('Ctrl Pts',(15.3413897506042,-41.0733153942767,-1.36126166406269));
#7471=CARTESIAN_POINT('Ctrl Pts',(15.3242948958371,-41.1124319810503,-1.30090464504928));
#7472=CARTESIAN_POINT('Ctrl Pts',(15.3071740583319,-41.1516080217382,-1.24045588845528));
#7473=CARTESIAN_POINT('Ctrl Pts',(15.2921187052635,-41.1894295601709,-1.17875107963721));
#7474=CARTESIAN_POINT('Ctrl Pts',(15.2791671350192,-41.2257407478499,-1.11609838715543));
#7475=CARTESIAN_POINT('Ctrl Pts',(15.2704790144623,-41.2500988735576,-1.07406995853756));
#7476=CARTESIAN_POINT('Ctrl Pts',(15.2627367477603,-41.2737779452521,-1.03161537789602));
#7477=CARTESIAN_POINT('Ctrl Pts',(15.255941797888,-41.2967389376301,-0.988830267143717));
#7478=CARTESIAN_POINT('Ctrl Pts',(15.2458125913074,-41.3309668038336,-0.92505066118307));
#7479=CARTESIAN_POINT('Ctrl Pts',(15.2379209804708,-41.364283552906,-0.859969813685587));
#7480=CARTESIAN_POINT('Ctrl Pts',(15.2323539847774,-41.396510870349,-0.793867798863232));
#7481=CARTESIAN_POINT('Ctrl Pts',(15.2267943508853,-41.4286955703515,-0.727853197418737));
#7482=CARTESIAN_POINT('Ctrl Pts',(15.223553397531,-41.4597933344992,-0.660820696333327));
#7483=CARTESIAN_POINT('Ctrl Pts',(15.2226758380192,-41.4896430359255,-0.5930750621331));
#7484=CARTESIAN_POINT('Ctrl Pts',(15.221798222738,-41.5194946343209,-0.52532512265114));
#7485=CARTESIAN_POINT('Ctrl Pts',(15.2232843886165,-41.5480976758437,-0.4568626034616));
#7486=CARTESIAN_POINT('Ctrl Pts',(15.2271348139984,-41.5753129178684,-0.388009033178963));
#7487=CARTESIAN_POINT('Ctrl Pts',(15.2309843078464,-41.6025215757062,-0.319172120649359));
#7488=CARTESIAN_POINT('Ctrl Pts',(15.2371968620786,-41.6283428458228,-0.249945031376208));
#7489=CARTESIAN_POINT('Ctrl Pts',(15.2457284985217,-41.6526639709981,-0.180655744943154));
#7490=CARTESIAN_POINT('Ctrl Pts',(15.2542731023327,-41.6770220622331,-0.111261144636752));
#7491=CARTESIAN_POINT('Ctrl Pts',(15.265143663798,-41.6998752669307,-0.0418048433736956));
#7492=CARTESIAN_POINT('Ctrl Pts',(15.2782531580267,-41.7211400920208,0.0273873077172026));
#7493=CARTESIAN_POINT('Ctrl Pts',(15.2870472165189,-41.7354048769474,0.0738025098054051));
#7494=CARTESIAN_POINT('Ctrl Pts',(15.2968478865887,-41.7489555293734,0.120098937661456));
#7495=CARTESIAN_POINT('Ctrl Pts',(15.3076189187291,-41.7617747973069,0.166181422977352));
#7496=CARTESIAN_POINT('Ctrl Pts',(15.3236752564046,-41.780884432485,0.234876412976531));
#7497=CARTESIAN_POINT('Ctrl Pts',(15.3422528729634,-41.7989191659951,0.30370533532348));
#7498=CARTESIAN_POINT('Ctrl Pts',(15.3633194390461,-41.8157695893768,0.37234447007484));
#7499=CARTESIAN_POINT('Ctrl Pts',(15.3843581466785,-41.8325977297399,0.440892836358044));
#7500=CARTESIAN_POINT('Ctrl Pts',(15.4078791891891,-41.8482444483706,0.509251242355893));
#7501=CARTESIAN_POINT('Ctrl Pts',(15.4338025321307,-41.8626206415506,0.577093346534493));
#7502=CARTESIAN_POINT('Ctrl Pts',(15.4597275225189,-41.8769977483476,0.644939762126132));
#7503=CARTESIAN_POINT('Ctrl Pts',(15.4880549427528,-41.8901039844429,0.712269124557562));
#7504=CARTESIAN_POINT('Ctrl Pts',(15.5186584489096,-41.9018733280804,0.778761359261807));
#7505=CARTESIAN_POINT('Ctrl Pts',(15.5492545511562,-41.9136398243591,0.845237507490883));
#7506=CARTESIAN_POINT('Ctrl Pts',(15.5821253183861,-41.9240699680251,0.910876280136906));
#7507=CARTESIAN_POINT('Ctrl Pts',(15.6171019638546,-41.9331230601206,0.975374241033202));
#7508=CARTESIAN_POINT('Ctrl Pts',(15.6521317708756,-41.9421899121529,1.03997023339279));
#7509=CARTESIAN_POINT('Ctrl Pts',(15.6892734311379,-41.9498754908882,1.10342135481053));
#7510=CARTESIAN_POINT('Ctrl Pts',(15.7283203630771,-41.9561653293342,1.16544861040137));
#7511=CARTESIAN_POINT('Ctrl Pts',(15.7545136698089,-41.960384653607,1.2070574859452));
#7512=CARTESIAN_POINT('Ctrl Pts',(15.7815635705291,-41.9639764580745,1.24802618569434));
#7513=CARTESIAN_POINT('Ctrl Pts',(15.8094000084028,-41.9669430094149,1.28827884419633));
#7514=CARTESIAN_POINT('Ctrl Pts',(15.8508956831299,-41.9713652364986,1.34828333297729));
#7515=CARTESIAN_POINT('Ctrl Pts',(15.8947296049228,-41.9748182353834,1.4072279179729));
#7516=CARTESIAN_POINT('Ctrl Pts',(15.9407455148334,-41.9772641483903,1.46480935021334));
#7517=CARTESIAN_POINT('Ctrl Pts',(15.9867005732529,-41.9797068269191,1.522314636703));
#7518=CARTESIAN_POINT('Ctrl Pts',(16.0348315554068,-41.981144990272,1.57845972694531));
#7519=CARTESIAN_POINT('Ctrl Pts',(16.0849379261041,-41.9815591058674,1.63296134034162));
#7520=CARTESIAN_POINT('Ctrl Pts',(16.1350474810962,-41.9819732477801,1.68746641735353));
#7521=CARTESIAN_POINT('Ctrl Pts',(16.1871322473098,-41.9813631737787,1.74032721705703));
#7522=CARTESIAN_POINT('Ctrl Pts',(16.2409521642729,-41.9797285163876,1.79128851362614));
#7523=CARTESIAN_POINT('Ctrl Pts',(16.2947590605767,-41.9780942544694,1.84223748112241));
#7524=CARTESIAN_POINT('Ctrl Pts',(16.3502997222452,-41.9754359284791,1.89128737321299));
#7525=CARTESIAN_POINT('Ctrl Pts',(16.4073021361913,-41.9717724372151,1.93821939640231));
#7526=CARTESIAN_POINT('Ctrl Pts',(16.4643911890006,-41.9681033777532,1.98522275230988));
#7527=CARTESIAN_POINT('Ctrl Pts',(16.5229458190129,-41.9634261726391,2.03010142110802));
#7528=CARTESIAN_POINT('Ctrl Pts',(16.5826693342596,-41.9577783801464,2.07267852251417));
#7529=CARTESIAN_POINT('Ctrl Pts',(16.6227328239181,-41.9539897505724,2.10123992341013));
#7530=CARTESIAN_POINT('Ctrl Pts',(16.6633218274874,-41.9497647503652,2.12876654161633));
#7531=CARTESIAN_POINT('Ctrl Pts',(16.7043430819143,-41.945119044319,2.15521684061908));
#7532=CARTESIAN_POINT('Ctrl Pts',(16.7654933137908,-41.9381937075413,2.19464620327067));
#7533=CARTESIAN_POINT('Ctrl Pts',(16.8283682976551,-41.9306533441131,2.23203175294738));
#7534=CARTESIAN_POINT('Ctrl Pts',(16.8927078099147,-41.9225201203709,2.26715077383057));
#7535=CARTESIAN_POINT('Ctrl Pts',(16.9569622395323,-41.9143976520127,2.30222335328179));
#7536=CARTESIAN_POINT('Ctrl Pts',(17.0226768047408,-41.9056839289559,2.33503490407215));
#7537=CARTESIAN_POINT('Ctrl Pts',(17.089558583264,-41.8964127583274,2.36540131373498));
#7538=CARTESIAN_POINT('Ctrl Pts',(17.1564446121707,-41.8871409985096,2.39576965320428));
#7539=CARTESIAN_POINT('Ctrl Pts',(17.2244973822525,-41.8773117931766,2.42369216050363));
#7540=CARTESIAN_POINT('Ctrl Pts',(17.2933987451626,-41.8669698589084,2.44902900915302));
#7541=CARTESIAN_POINT('Ctrl Pts',(17.3622834387564,-41.8566304266658,2.47435972805509));
#7542=CARTESIAN_POINT('Ctrl Pts',(17.4320156256809,-41.8457786197484,2.49710580690362));
#7543=CARTESIAN_POINT('Ctrl Pts',(17.50226209398,-41.8344686701383,2.5171764296093));
#7544=CARTESIAN_POINT('Ctrl Pts',(17.5726153309896,-41.8231415303581,2.53727755796966));
#7545=CARTESIAN_POINT('Ctrl Pts',(17.643483700434,-41.8113549844685,2.55469500339256));
#7546=CARTESIAN_POINT('Ctrl Pts',(17.7145276936807,-41.7991713109554,2.56938903350715));
#7547=CARTESIAN_POINT('Ctrl Pts',(17.7621851411193,-41.7909983078129,2.57924602402589));
#7548=CARTESIAN_POINT('Ctrl Pts',(17.8099215343723,-41.7826467602478,2.58787857636225));
#7549=CARTESIAN_POINT('Ctrl Pts',(17.8576356015541,-41.774136956956,2.59528770975727));
#7550=CARTESIAN_POINT('Ctrl Pts',(17.9287627845899,-41.7614514247412,2.60633247743795));
#7551=CARTESIAN_POINT('Ctrl Pts',(18.000692271499,-41.7486834415431,2.61475432517955));
#7552=CARTESIAN_POINT('Ctrl Pts',(18.0731004304624,-41.7358917824549,2.62045518191384));
#7553=CARTESIAN_POINT('Ctrl Pts',(18.1454128367952,-41.723117039071,2.6261484998288));
#7554=CARTESIAN_POINT('Ctrl Pts',(18.2182019841964,-41.7103188040807,2.62912778112538));
#7555=CARTESIAN_POINT('Ctrl Pts',(18.291128975358,-41.6975574283081,2.62934454720094));
#7556=CARTESIAN_POINT('Ctrl Pts',(18.3640606010804,-41.6847952415412,2.62956132705215));
#7557=CARTESIAN_POINT('Ctrl Pts',(18.437129373917,-41.6720700456673,2.62701514692934));
#7558=CARTESIAN_POINT('Ctrl Pts',(18.5099901525822,-41.6594421416469,2.62170927404767));
#7559=CARTESIAN_POINT('Ctrl Pts',(18.5828333040297,-41.6468172926969,2.61640468481653));
#7560=CARTESIAN_POINT('Ctrl Pts',(18.6554678414049,-41.6342898129655,2.60834181054508));
#7561=CARTESIAN_POINT('Ctrl Pts',(18.7275535025415,-41.6219180048756,2.59757579979054));
#7562=CARTESIAN_POINT('Ctrl Pts',(18.7997487278061,-41.6095273926804,2.58679342560727));
#7563=CARTESIAN_POINT('Ctrl Pts',(18.8713927192498,-41.5972930412203,2.57329990897757));
#7564=CARTESIAN_POINT('Ctrl Pts',(18.9421589256826,-41.5852697479988,2.55720053492563));
#7565=CARTESIAN_POINT('Ctrl Pts',(18.989630029282,-41.5772043305221,2.54640081720681));
#7566=CARTESIAN_POINT('Ctrl Pts',(19.036706470869,-41.569233806229,2.53442952081175));
#7567=CARTESIAN_POINT('Ctrl Pts',(19.0832957533591,-41.5613733976818,2.52133001886304));
#7568=CARTESIAN_POINT('Ctrl Pts',(19.1527462240253,-41.549655915805,2.50180263987786));
#7569=CARTESIAN_POINT('Ctrl Pts',(19.2219502995763,-41.5384614495882,2.47959273545134));
#7570=CARTESIAN_POINT('Ctrl Pts',(19.2905740551605,-41.5278547168098,2.45474630344356));
#7571=CARTESIAN_POINT('Ctrl Pts',(19.3591070626122,-41.5172620103869,2.42993272838577));
#7572=CARTESIAN_POINT('Ctrl Pts',(19.4270605835762,-41.5072556256214,2.40248965698989));
#7573=CARTESIAN_POINT('Ctrl Pts',(19.4941052636857,-41.4978904037176,2.37251384629913));
#7574=CARTESIAN_POINT('Ctrl Pts',(19.5611542045323,-41.4885245866474,2.3425361306243));
#7575=CARTESIAN_POINT('Ctrl Pts',(19.6272934981489,-41.4798001274666,2.31002556527966));
#7576=CARTESIAN_POINT('Ctrl Pts',(19.6922074515294,-41.4717603251636,2.27512786406354));
#7577=CARTESIAN_POINT('Ctrl Pts',(19.7571057002683,-41.4637224679311,2.24023860565303));
#7578=CARTESIAN_POINT('Ctrl Pts',(19.8207785671862,-41.4563690110505,2.20296372939584));
#7579=CARTESIAN_POINT('Ctrl Pts',(19.8829342849465,-41.449730258442,2.16349342564761));
#7580=CARTESIAN_POINT('Ctrl Pts',(19.9451844741582,-41.4430814154891,2.12396313036491));
#7581=CARTESIAN_POINT('Ctrl Pts',(20.0059123487215,-41.4371494870487,2.08223120813824));
#7582=CARTESIAN_POINT('Ctrl Pts',(20.0648575226136,-41.4319510701467,2.03852710839656));
#7583=CARTESIAN_POINT('Ctrl Pts',(20.1043988884376,-41.4284638889094,2.00920969898396));
#7584=CARTESIAN_POINT('Ctrl Pts',(20.1431387485306,-41.4253064921863,1.97900561592653));
#7585=CARTESIAN_POINT('Ctrl Pts',(20.1810084262852,-41.4224803497805,1.94799199564958));
#7586=CARTESIAN_POINT('Ctrl Pts',(20.2374606145016,-41.418267429775,1.90176010689434));
#7587=CARTESIAN_POINT('Ctrl Pts',(20.2926991654359,-41.4151359629548,1.85331739425825));
#7588=CARTESIAN_POINT('Ctrl Pts',(20.3464350150602,-41.4131247666898,1.80284481408933));
#7589=CARTESIAN_POINT('Ctrl Pts',(20.4000998043366,-41.4111162300331,1.75243897891717));
#7590=CARTESIAN_POINT('Ctrl Pts',(20.4522652453572,-41.4102250974731,1.70000899168553));
#7591=CARTESIAN_POINT('Ctrl Pts',(20.5026651545721,-41.4104697385263,1.64577768116439));
#7592=CARTESIAN_POINT('Ctrl Pts',(20.5530682667365,-41.4107143951265,1.59154292420549));
#7593=CARTESIAN_POINT('Ctrl Pts',(20.6017050675013,-41.4120950049051,1.5355070898215));
#7594=CARTESIAN_POINT('Ctrl Pts',(20.6483399207653,-41.4146086459749,1.47792947798907));
#7595=CARTESIAN_POINT('Ctrl Pts',(20.6949634916534,-41.4171216789191,1.42036579591542));
#7596=CARTESIAN_POINT('Ctrl Pts',(20.7395856359485,-41.4207671618734,1.36126166406089));
#7597=CARTESIAN_POINT('Ctrl Pts',(20.7820090211876,-41.425520876758,1.30090464504709));
#7598=CARTESIAN_POINT('Ctrl Pts',(20.8244968863956,-41.4302818168884,1.24045588845307));
#7599=CARTESIAN_POINT('Ctrl Pts',(20.8647789760227,-41.4361542678846,1.17875107963501));
#7600=CARTESIAN_POINT('Ctrl Pts',(20.9027011721163,-41.4430934728737,1.11609838715323));
#7601=CARTESIAN_POINT('Ctrl Pts',(20.9281399880457,-41.4477484026141,1.07406995853608));
#7602=CARTESIAN_POINT('Ctrl Pts',(20.9525177990217,-41.4528829388144,1.03161537789526));
#7603=CARTESIAN_POINT('Ctrl Pts',(20.9758000766529,-41.4584788357964,0.988830267143709));
#7604=CARTESIAN_POINT('Ctrl Pts',(21.0105068815928,-41.4668206186793,0.925050661182975));
#7605=CARTESIAN_POINT('Ctrl Pts',(21.0433058380794,-41.4766446577542,0.85996981368539));
#7606=CARTESIAN_POINT('Ctrl Pts',(21.0739990115276,-41.4879371567824,0.793867798862945));
#7607=CARTESIAN_POINT('Ctrl Pts',(21.1046515962888,-41.4992147225973,0.72785319741889));
#7608=CARTESIAN_POINT('Ctrl Pts',(21.1332035267186,-41.5119568567338,0.660820696333936));
#7609=CARTESIAN_POINT('Ctrl Pts',(21.1594929062049,-41.5261217186163,0.593075062134168));
#7610=CARTESIAN_POINT('Ctrl Pts',(21.1857839563995,-41.5402874806857,0.525325122652251));
#7611=CARTESIAN_POINT('Ctrl Pts',(21.2098118340445,-41.5558760588521,0.456862603462757));
#7612=CARTESIAN_POINT('Ctrl Pts',(21.2314557123171,-41.5728182460605,0.388009033180158));
#7613=CARTESIAN_POINT('Ctrl Pts',(21.2530943542834,-41.5897563344434,0.319172120650899));
#7614=CARTESIAN_POINT('Ctrl Pts',(21.2723499530461,-41.6080471992891,0.249945031378103));
#7615=CARTESIAN_POINT('Ctrl Pts',(21.2891468470751,-41.6275963757721,0.180655744945393));
#7616=CARTESIAN_POINT('Ctrl Pts',(21.3059692709667,-41.6471752653552,0.111261144639139));
#7617=CARTESIAN_POINT('Ctrl Pts',(21.3203254460601,-41.6680160500862,0.0418048433762189));
#7618=CARTESIAN_POINT('Ctrl Pts',(21.3321865776809,-41.690001617664,-0.0273873077145389));
#7619=CARTESIAN_POINT('Ctrl Pts',(21.3401432145609,-41.7047498881843,-0.0738025098036383));
#7620=CARTESIAN_POINT('Ctrl Pts',(21.346978088765,-41.7200128436521,-0.120098937660575));
#7621=CARTESIAN_POINT('Ctrl Pts',(21.3526943843832,-41.7357504650777,-0.166181422977357));
#7622=CARTESIAN_POINT('Ctrl Pts',(21.3612156450668,-41.7592104789858,-0.234876412977378));
#7623=CARTESIAN_POINT('Ctrl Pts',(21.3675453741577,-41.7843165336228,-0.303705335325169));
#7624=CARTESIAN_POINT('Ctrl Pts',(21.3716049858294,-41.8109859267122,-0.372344470077365));
#7625=CARTESIAN_POINT('Ctrl Pts',(21.3756592290661,-41.837620052166,-0.440892836360022));
#7626=CARTESIAN_POINT('Ctrl Pts',(21.3774491636307,-41.8658132318188,-0.509251242357337));
#7627=CARTESIAN_POINT('Ctrl Pts',(21.3769376406635,-41.8954516019471,-0.577093346535395));
#7628=CARTESIAN_POINT('Ctrl Pts',(21.3764260851885,-41.9250918556145,-0.644939762126841));
#7629=CARTESIAN_POINT('Ctrl Pts',(21.373612708478,-41.9561772392083,-0.712269124558073));
#7630=CARTESIAN_POINT('Ctrl Pts',(21.3685035059756,-41.9885653248037,-0.77876135926213));
#7631=CARTESIAN_POINT('Ctrl Pts',(21.3633955395432,-42.0209455747454,-0.845237507491449));
#7632=CARTESIAN_POINT('Ctrl Pts',(21.3559929253081,-42.0546275660416,-0.910876280137711));
#7633=CARTESIAN_POINT('Ctrl Pts',(21.3463448103113,-42.0894447756044,-0.975374241034235));
#7634=CARTESIAN_POINT('Ctrl Pts',(21.3366820309931,-42.1243149043904,-1.03997023339384));
#7635=CARTESIAN_POINT('Ctrl Pts',(21.3247671072895,-42.160323315084,-1.1034213548116));
#7636=CARTESIAN_POINT('Ctrl Pts',(21.3106908011998,-42.1972838693061,-1.16544861040246));
#7637=CARTESIAN_POINT('Ctrl Pts',(21.301248189841,-42.2220776004812,-1.20705748594591));
#7638=CARTESIAN_POINT('Ctrl Pts',(21.2908338333953,-42.2472994039083,-1.24802618569469));
#7639=CARTESIAN_POINT('Ctrl Pts',(21.2794847232809,-42.2728897419278,-1.28827884419633));
#7640=CARTESIAN_POINT('Ctrl Pts',(21.2625666469131,-42.3110371639306,-1.34828333297748));
#7641=CARTESIAN_POINT('Ctrl Pts',(21.24364007077,-42.3507249531932,-1.40722791797326));
#7642=CARTESIAN_POINT('Ctrl Pts',(21.2227503386141,-42.3917988566577,-1.46480935021387));
#7643=CARTESIAN_POINT('Ctrl Pts',(21.2018882310633,-42.4328184439464,-1.52231463670436));
#7644=CARTESIAN_POINT('Ctrl Pts',(21.1790682259843,-42.4752201788778,-1.57845972694747));
#7645=CARTESIAN_POINT('Ctrl Pts',(21.154373675261,-42.5188206265915,-1.63296134034452));
#7646=CARTESIAN_POINT('Ctrl Pts',(21.129677555182,-42.5624238451434,-1.68746641735642));
#7647=CARTESIAN_POINT('Ctrl Pts',(21.1031068324917,-42.607225538834,-1.74032721705991));
#7648=CARTESIAN_POINT('Ctrl Pts',(21.0747812191829,-42.6530176254581,-1.79128851362901));
#7649=CARTESIAN_POINT('Ctrl Pts',(21.0464624586933,-42.6987986335969,-1.84223748112507));
#7650=CARTESIAN_POINT('Ctrl Pts',(21.01638995002,-42.7455690945495,-1.89128737321547));
#7651=CARTESIAN_POINT('Ctrl Pts',(20.9847160665458,-42.7931028874718,-1.9382193964046));
#7652=CARTESIAN_POINT('Ctrl Pts',(20.9529940414388,-42.8407089277522,-1.98522275231258));
#7653=CARTESIAN_POINT('Ctrl Pts',(20.9196661479847,-42.8890801222955,-2.03010142111108));
#7654=CARTESIAN_POINT('Ctrl Pts',(20.8849132585869,-42.9379783074566,-2.07267852251754));
#7655=CARTESIAN_POINT('Ctrl Pts',(20.8616004643019,-42.9707799924769,-2.1012399234123));
#7656=CARTESIAN_POINT('Ctrl Pts',(20.8376470050078,-43.0038186005773,-2.12876654161737));
#7657=CARTESIAN_POINT('Ctrl Pts',(20.8131130783408,-43.0370211959817,-2.15521684061907));
#7658=CARTESIAN_POINT('Ctrl Pts',(20.7765404448229,-43.0865161818458,-2.19464620327108));
#7659=CARTESIAN_POINT('Ctrl Pts',(20.7385728066078,-43.1371973334212,-2.23203175294819));
#7660=CARTESIAN_POINT('Ctrl Pts',(20.6993594721021,-43.1888503736346,-2.26715077383171));
#7661=CARTESIAN_POINT('Ctrl Pts',(20.6601979933538,-43.2404351078099,-2.30222335328278));
#7662=CARTESIAN_POINT('Ctrl Pts',(20.6197944052208,-43.2929887291506,-2.335034904073));
#7663=CARTESIAN_POINT('Ctrl Pts',(20.5783244466722,-43.3462744630876,-2.36540131373571));
#7664=CARTESIAN_POINT('Ctrl Pts',(20.5368518526788,-43.3995635833702,-2.39576965320497));
#7665=CARTESIAN_POINT('Ctrl Pts',(20.4943131261206,-43.4535844083924,-2.42369216050428));
#7666=CARTESIAN_POINT('Ctrl Pts',(20.450906066865,-43.5080837718938,-2.44902900915362));
#7667=CARTESIAN_POINT('Ctrl Pts',(20.4075095090847,-43.5625699503573,-2.47435972805595));
#7668=CARTESIAN_POINT('Ctrl Pts',(20.3632454751545,-43.6175338922374,-2.49710580690468));
#7669=CARTESIAN_POINT('Ctrl Pts',(20.3183275373265,-43.6727141435061,-2.51717642961049));
#7670=CARTESIAN_POINT('Ctrl Pts',(20.2733413280198,-43.7279782641049,-2.53727755797076));
#7671=CARTESIAN_POINT('Ctrl Pts',(20.2276996951343,-43.7834587994236,-2.55469500339356));
#7672=CARTESIAN_POINT('Ctrl Pts',(20.1816263277371,-43.8388928656051,-2.56938903350804));
#7673=CARTESIAN_POINT('Ctrl Pts',(20.1507195756722,-43.8760789241941,-2.57924602402641));
#7674=CARTESIAN_POINT('Ctrl Pts',(20.1196187266944,-43.9132440796525,-2.58787857636247));
#7675=CARTESIAN_POINT('Ctrl Pts',(20.0883919872725,-43.9503107723028,-2.59528770975726));
#7676=CARTESIAN_POINT('Ctrl Pts',(20.0418424025962,-44.0055659536039,-2.60633247743792));
#7677=CARTESIAN_POINT('Ctrl Pts',(19.994820261337,-44.0614747249492,-2.6147543251795));
#7678=CARTESIAN_POINT('Ctrl Pts',(19.9475382801285,-44.1177862005085,-2.62045518191379));
#7679=CARTESIAN_POINT('Ctrl Pts',(19.9003188246649,-44.1740232097094,-2.62614849982876));
#7680=CARTESIAN_POINT('Ctrl Pts',(19.8528406543392,-44.2306613429835,-2.62912778112535));
#7681=CARTESIAN_POINT('Ctrl Pts',(19.8053254831521,-44.2874372820646,-2.62934454720094));
#7682=CARTESIAN_POINT('Ctrl Pts',(19.7578072923429,-44.3442168292961,-2.62956132705216));
#7683=CARTESIAN_POINT('Ctrl Pts',(19.7102525630296,-44.401133644859,-2.62701514692937));
#7684=CARTESIAN_POINT('Ctrl Pts',(19.6628860880186,-44.4579189781125,-2.62170927404771));
#7685=CARTESIAN_POINT('Ctrl Pts',(19.6155310723851,-44.514690573283,-2.61640468481656));
#7686=CARTESIAN_POINT('Ctrl Pts',(19.5683646880045,-44.5713301879767,-2.60834181054507));
#7687=CARTESIAN_POINT('Ctrl Pts',(19.5216075573393,-44.6275722977249,-2.59757579979048));
#7688=CARTESIAN_POINT('Ctrl Pts',(19.4747793597774,-44.6838998907385,-2.58679342560716));
#7689=CARTESIAN_POINT('Ctrl Pts',(19.4283621048922,-44.7398282316274,-2.57329990897739));
#7690=CARTESIAN_POINT('Ctrl Pts',(19.3825665243087,-44.7951019175171,-2.55720053492538));
#7691=CARTESIAN_POINT('Ctrl Pts',(19.3518461160823,-44.8321803904412,-2.54640081720663));
#7692=CARTESIAN_POINT('Ctrl Pts',(19.3214052187697,-44.8689645226285,-2.53442952081165));
#7693=CARTESIAN_POINT('Ctrl Pts',(19.2913032640389,-44.9053818205351,-2.52133001886304));
#7694=CARTESIAN_POINT('Ctrl Pts',(19.246430467523,-44.9596688598067,-2.5018026728599));
#7695=CARTESIAN_POINT('Ctrl Pts',(19.202133795719,-45.0140040172023,-2.47959281974212));
#7696=CARTESIAN_POINT('Ctrl Pts',(19.1586362574803,-45.068130464348,-2.45474645544533));
#7697=CARTESIAN_POINT('Ctrl Pts',(19.1134700774478,-45.1243332968597,-2.42894694107226));
#7698=CARTESIAN_POINT('Ctrl Pts',(19.0691661346203,-45.1803104983177,-2.40030445526987));
#7699=CARTESIAN_POINT('Ctrl Pts',(19.0259625921186,-45.2357723552297,-2.36892887071559));
#7700=CARTESIAN_POINT('Ctrl Pts',(18.9827590496168,-45.2912342121417,-2.3375532861613));
#7701=CARTESIAN_POINT('Ctrl Pts',(18.9406564439223,-45.3461800674173,-2.30344486801562));
#7702=CARTESIAN_POINT('Ctrl Pts',(18.8998729273403,-45.4003277207435,-2.26677050498056));
#7703=CARTESIAN_POINT('Origin',(5.49999999999995,-19.5262794416289,2.16840434497101E-16));
#7704=CARTESIAN_POINT('',(7.09807621135328,-16.29422863406,-1.50553605247105E-16));
#7705=CARTESIAN_POINT('Origin',(4.49999999999996,-17.79422863406,2.16840434497101E-16));
#7706=CARTESIAN_POINT('',(8.09807621135327,-18.0262794416289,-1.50553605247105E-16));
#7707=CARTESIAN_POINT('',(8.09807621135327,-18.0262794416289,-1.50553605247105E-16));
#7708=CARTESIAN_POINT('Origin',(5.49999999999995,-19.5262794416289,2.16840434497101E-16));
#7709=CARTESIAN_POINT('Origin',(0.,-10.,3.));
#7710=CARTESIAN_POINT('',(1.5,-10.,3.));
#7711=CARTESIAN_POINT('Origin',(0.,-10.,3.));
#7712=CARTESIAN_POINT('',(1.5,-10.,-3.));
#7713=CARTESIAN_POINT('',(1.5,-10.,3.));
#7714=CARTESIAN_POINT('Origin',(0.,-10.,-3.));
#7715=CARTESIAN_POINT('Origin',(0.,-10.,3.));
#7716=CARTESIAN_POINT('',(2.5,-10.,-3.));
#7717=CARTESIAN_POINT('Origin',(0.,-10.,-3.));
#7718=CARTESIAN_POINT('',(2.5,-10.,3.));
#7719=CARTESIAN_POINT('',(2.5,-10.,3.));
#7720=CARTESIAN_POINT('Origin',(0.,-10.,3.));
#7721=CARTESIAN_POINT('',(2.40822301019062,-10.6711646096066,1.));
#7722=CARTESIAN_POINT('',(-0.622865903054925,-12.4211646096066,1.));
#7723=CARTESIAN_POINT('Origin',(0.,-10.,1.));
#7724=CARTESIAN_POINT('',(2.40822301019062,-10.6711646096066,-1.));
#7725=CARTESIAN_POINT('',(2.40822301019062,-10.6711646096066,3.));
#7726=CARTESIAN_POINT('',(-0.622865903054925,-12.4211646096066,-1.));
#7727=CARTESIAN_POINT('Origin',(0.,-10.,-1.));
#7728=CARTESIAN_POINT('',(-0.622865903054925,-12.4211646096066,3.));
#7729=CARTESIAN_POINT('Origin',(-0.76554445662278,-12.1740381056767,1.));
#7730=CARTESIAN_POINT('',(2.98445554337718,-18.66922863406,1.));
#7731=CARTESIAN_POINT('',(2.98445554337718,-18.66922863406,-1.));
#7732=CARTESIAN_POINT('',(2.98445554337718,-18.66922863406,1.));
#7733=CARTESIAN_POINT('',(-0.76554445662278,-12.1740381056767,1.));
#7734=CARTESIAN_POINT('',(-0.76554445662278,-12.1740381056767,-1.));
#7735=CARTESIAN_POINT('Origin',(2.26554445662277,-10.4240381056767,1.));
#7736=CARTESIAN_POINT('',(6.01554445662273,-16.91922863406,1.));
#7737=CARTESIAN_POINT('',(2.26554445662277,-10.4240381056767,1.));
#7738=CARTESIAN_POINT('',(6.01554445662273,-16.91922863406,-1.));
#7739=CARTESIAN_POINT('',(6.01554445662273,-16.91922863406,1.));
#7740=CARTESIAN_POINT('',(2.26554445662277,-10.4240381056767,-1.));
#7741=CARTESIAN_POINT('Origin',(0.,0.,1.));
#7742=CARTESIAN_POINT('',(8.83012701892212,-15.29422863406,1.));
#7743=CARTESIAN_POINT('Origin',(0.,0.,-1.));
#7744=CARTESIAN_POINT('',(8.83012701892212,-15.29422863406,-1.));
#7745=CARTESIAN_POINT('Origin',(0.,-10.,3.));
#7746=CARTESIAN_POINT('Origin',(0.,-10.,-3.));
#7747=CARTESIAN_POINT('Origin',(4.49999999999996,-17.79422863406,2.16840434497101E-16));
#7748=CARTESIAN_POINT('Origin',(5.49999999999995,-19.5262794416289,2.16840434497101E-16));
#7749=CARTESIAN_POINT('Ctrl Pts',(3.23546955922298,-20.8337067011995,-0.275782109461831));
#7750=CARTESIAN_POINT('Ctrl Pts',(3.19478646287985,-20.8571950978247,-0.160590892492083));
#7751=CARTESIAN_POINT('Ctrl Pts',(3.16609800813309,-20.8737583848954,-0.0273286702176377));
#7752=CARTESIAN_POINT('Ctrl Pts',(3.13988678358144,-20.888891442446,0.302695031901609));
#7753=CARTESIAN_POINT('Ctrl Pts',(3.15185977323478,-20.8819788336467,0.505045958749506));
#7754=CARTESIAN_POINT('Ctrl Pts',(3.24434506152257,-20.8285824275577,0.905660854503917));
#7755=CARTESIAN_POINT('Ctrl Pts',(3.31916946032855,-20.7853825407651,1.09246911691544));
#7756=CARTESIAN_POINT('Ctrl Pts',(3.51311377456417,-20.6734087387334,1.40491660680051));
#7757=CARTESIAN_POINT('Ctrl Pts',(3.62398989329116,-20.6093943817396,1.52876642599518));
#7758=CARTESIAN_POINT('Ctrl Pts',(3.81928683300962,-20.4966396410213,1.66967867861614));
#7759=CARTESIAN_POINT('Ctrl Pts',(3.89646793982015,-20.4520791082279,1.70509112652145));
#7760=CARTESIAN_POINT('Ctrl Pts',(4.01069549422891,-20.3861297989411,1.72863250364951));
#7761=CARTESIAN_POINT('Ctrl Pts',(4.05275149332675,-20.3618487565409,1.72894065285834));
#7762=CARTESIAN_POINT('Ctrl Pts',(4.11567773776654,-20.3255182723745,1.71361810977144));
#7763=CARTESIAN_POINT('Ctrl Pts',(4.14030222240021,-20.3113013195102,1.70246840376101));
#7764=CARTESIAN_POINT('Ctrl Pts',(4.18011703938166,-20.2883142242082,1.67084097729165));
#7765=CARTESIAN_POINT('Ctrl Pts',(4.19525068130979,-20.2795768119921,1.65305151274377));
#7766=CARTESIAN_POINT('Ctrl Pts',(4.22086530937756,-20.264788199582,1.60918078140847));
#7767=CARTESIAN_POINT('Ctrl Pts',(4.2301173432281,-20.2594465353219,1.58365589452017));
#7768=CARTESIAN_POINT('Ctrl Pts',(4.24553996400391,-20.2505422810654,1.51733112234353));
#7769=CARTESIAN_POINT('Ctrl Pts',(4.24810838618388,-20.2490594018618,1.47473909891144));
#7770=CARTESIAN_POINT('Ctrl Pts',(4.24563774453512,-20.2504858274828,1.34638123818485));
#7771=CARTESIAN_POINT('Ctrl Pts',(4.22827734454219,-20.2605088590919,1.24517362806592));
#7772=CARTESIAN_POINT('Ctrl Pts',(4.20325688541709,-20.2749544279031,1.13384235805383));
#7773=CARTESIAN_POINT('Origin',(18.6221620196843,-45.0864402030305,-1.2339885196899));
#7774=CARTESIAN_POINT('Ctrl Pts',(18.6886546214932,-45.2109506803708,-1.32333454806873));
#7775=CARTESIAN_POINT('Ctrl Pts',(18.6534200942688,-45.1984263741837,-1.33050220974328));
#7776=CARTESIAN_POINT('Ctrl Pts',(18.6179251635874,-45.1908739234988,-1.34288752657174));
#7777=CARTESIAN_POINT('Ctrl Pts',(18.5470215891454,-45.185850564164,-1.37789046380575));
#7778=CARTESIAN_POINT('Ctrl Pts',(18.5124223059912,-45.1893923862984,-1.40108283157508));
#7779=CARTESIAN_POINT('Ctrl Pts',(18.4521552156851,-45.2081885454495,-1.45435746423492));
#7780=CARTESIAN_POINT('Ctrl Pts',(18.426979600515,-45.2232129895809,-1.48392674358772));
#7781=CARTESIAN_POINT('Ctrl Pts',(18.389723568323,-45.2625315455739,-1.54510765557877));
#7782=CARTESIAN_POINT('Ctrl Pts',(18.3777553489124,-45.2862666614671,-1.57608573045647));
#7783=CARTESIAN_POINT('Ctrl Pts',(18.3679521931281,-45.3419359617658,-1.63840496576467));
#7784=CARTESIAN_POINT('Ctrl Pts',(18.3717657514849,-45.3715611958691,-1.66645854752162));
#7785=CARTESIAN_POINT('Ctrl Pts',(18.3912949388311,-45.4302955552117,-1.71530376490681));
#7786=CARTESIAN_POINT('Ctrl Pts',(18.4084911637847,-45.4596223662212,-1.73547949720297));
#7787=CARTESIAN_POINT('Ctrl Pts',(18.4492950593841,-45.5109364170729,-1.76471771766154));
#7788=CARTESIAN_POINT('Ctrl Pts',(18.4757817897306,-45.5370275164247,-1.77633599562865));
#7789=CARTESIAN_POINT('Ctrl Pts',(18.5261801552888,-45.5734326754053,-1.78494045784658));
#7790=CARTESIAN_POINT('Ctrl Pts',(18.5444289208832,-45.584745828607,-1.78615024656862));
#7791=CARTESIAN_POINT('Ctrl Pts',(18.5825570867818,-45.6048265898968,-1.78505107379611));
#7792=CARTESIAN_POINT('Ctrl Pts',(18.6022265451803,-45.6134733978683,-1.78273773091633));
#7793=CARTESIAN_POINT('Ctrl Pts',(18.6221620188092,-45.6205950572474,-1.77871850142445));
#7794=CARTESIAN_POINT('Ctrl Pts',(18.8143835621595,-45.3725581651887,-2.29264601963605));
#7795=CARTESIAN_POINT('Ctrl Pts',(18.799421862846,-45.366692611081,-2.29601323464502));
#7796=CARTESIAN_POINT('Ctrl Pts',(18.7845100498018,-45.360314232665,-2.29875605009942));
#7797=CARTESIAN_POINT('Ctrl Pts',(18.7622518217144,-45.3499802606706,-2.30191697923756));
#7798=CARTESIAN_POINT('Ctrl Pts',(18.7548376244511,-45.3464005096126,-2.30281208768347));
#7799=CARTESIAN_POINT('Ctrl Pts',(18.7400559460073,-45.3389851193664,-2.30427767151426));
#7800=CARTESIAN_POINT('Ctrl Pts',(18.7326634287054,-45.3351353187089,-2.3048487962336));
#7801=CARTESIAN_POINT('Ctrl Pts',(18.7107560010767,-45.3232997976908,-2.30605306308975));
#7802=CARTESIAN_POINT('Ctrl Pts',(18.69647386335,-45.3150169340706,-2.30618966865469));
#7803=CARTESIAN_POINT('Ctrl Pts',(18.668502415621,-45.297660633993,-2.30516256178937));
#7804=CARTESIAN_POINT('Ctrl Pts',(18.6548195137261,-45.2885911850942,-2.3039990903213));
#7805=CARTESIAN_POINT('Ctrl Pts',(18.6280626028503,-45.269665384442,-2.3003672370976));
#7806=CARTESIAN_POINT('Ctrl Pts',(18.6150036070141,-45.2598211706463,-2.29790262175487));
#7807=CARTESIAN_POINT('Ctrl Pts',(18.5958424864585,-45.244407875027,-2.29318270097683));
#7808=CARTESIAN_POINT('Ctrl Pts',(18.5895683887268,-45.2391944776938,-2.29144761696805));
#7809=CARTESIAN_POINT('Ctrl Pts',(18.5773056208511,-45.2286717796098,-2.28767708876727));
#7810=CARTESIAN_POINT('Ctrl Pts',(18.571302721882,-45.2233510576313,-2.28563816739681));
#7811=CARTESIAN_POINT('Ctrl Pts',(18.5536922471648,-45.2072288630195,-2.27907242657322));
#7812=CARTESIAN_POINT('Ctrl Pts',(18.5424689819436,-45.1962571521417,-2.27409434987581));
#7813=CARTESIAN_POINT('Ctrl Pts',(18.5210534195265,-45.1738767847226,-2.26294902313096));
#7814=CARTESIAN_POINT('Ctrl Pts',(18.5108563517502,-45.1624608434638,-2.2567766707594));
#7815=CARTESIAN_POINT('Ctrl Pts',(18.4915255994775,-45.1392076266336,-2.24323675136636));
#7816=CARTESIAN_POINT('Ctrl Pts',(18.4823425082748,-45.1272886562345,-2.23580916151862));
#7817=CARTESIAN_POINT('Ctrl Pts',(18.4654779188592,-45.1035758058956,-2.22008460131979));
#7818=CARTESIAN_POINT('Ctrl Pts',(18.4577062314804,-45.0916806335816,-2.21173267647811));
#7819=CARTESIAN_POINT('Ctrl Pts',(18.4435024450096,-45.0678731904181,-2.19410226893954));
#7820=CARTESIAN_POINT('Ctrl Pts',(18.4370613768115,-45.0559500756431,-2.18481745164526));
#7821=CARTESIAN_POINT('Ctrl Pts',(18.4283974556018,-45.0380432871124,-2.17018589369896));
#7822=CARTESIAN_POINT('Ctrl Pts',(18.4256747602959,-45.0320672479267,-2.1651880723044));
#7823=CARTESIAN_POINT('Ctrl Pts',(18.4205692543985,-45.0201143102805,-2.15495946376726));
#7824=CARTESIAN_POINT('Ctrl Pts',(18.4181811783317,-45.0141230761169,-2.14971582230565));
#7825=CARTESIAN_POINT('Ctrl Pts',(18.411557743034,-44.996204520912,-2.13367800718911));
#7826=CARTESIAN_POINT('Ctrl Pts',(18.4079107853335,-44.9844773686462,-2.12271082270486));
#7827=CARTESIAN_POINT('Ctrl Pts',(18.4020639448891,-44.9613631523321,-2.10017046144782));
#7828=CARTESIAN_POINT('Ctrl Pts',(18.3998694271457,-44.9499903424353,-2.08860999048261));
#7829=CARTESIAN_POINT('Ctrl Pts',(18.3969224236575,-44.927612616283,-2.06491243172319));
#7830=CARTESIAN_POINT('Ctrl Pts',(18.3961709968481,-44.9166059372197,-2.05277259205872));
#7831=CARTESIAN_POINT('Ctrl Pts',(18.3961415719036,-44.9003846022915,-2.03412910558187));
#7832=CARTESIAN_POINT('Ctrl Pts',(18.3963173860228,-44.8950134660865,-2.02782648667107));
#7833=CARTESIAN_POINT('Ctrl Pts',(18.3970392739734,-44.8844199010087,-2.01513320991302));
#7834=CARTESIAN_POINT('Ctrl Pts',(18.3975826848578,-44.879219163033,-2.00876936719308));
#7835=CARTESIAN_POINT('Ctrl Pts',(18.3997509614153,-44.8639020731823,-1.98962815132851));
#7836=CARTESIAN_POINT('Ctrl Pts',(18.4019103092124,-44.8540407117655,-1.97676890218923));
#7837=CARTESIAN_POINT('Ctrl Pts',(18.407622325662,-44.835045996909,-1.95090394599962));
#7838=CARTESIAN_POINT('Ctrl Pts',(18.4111751980384,-44.825905164125,-1.93788950367134));
#7839=CARTESIAN_POINT('Ctrl Pts',(18.4196773870788,-44.8083449742005,-1.91169905664016));
#7840=CARTESIAN_POINT('Ctrl Pts',(18.4246337291704,-44.7999153918194,-1.89850633451621));
#7841=CARTESIAN_POINT('Ctrl Pts',(18.4359627695104,-44.7838395187261,-1.87201135519203));
#7842=CARTESIAN_POINT('Ctrl Pts',(18.4422430814637,-44.7763186261024,-1.85891858586588));
#7843=CARTESIAN_POINT('Ctrl Pts',(18.4560163442605,-44.7622376811399,-1.83296819839048));
#7844=CARTESIAN_POINT('Ctrl Pts',(18.4635048906187,-44.7556841943707,-1.82012124842252));
#7845=CARTESIAN_POINT('Ctrl Pts',(18.4796749688842,-44.7435444443489,-1.79468113425342));
#7846=CARTESIAN_POINT('Ctrl Pts',(18.4883628415307,-44.737956512423,-1.78208152867849));
#7847=CARTESIAN_POINT('Ctrl Pts',(18.5069294527721,-44.7277745729134,-1.75716664715693));
#7848=CARTESIAN_POINT('Ctrl Pts',(18.5168839026318,-44.7231591454028,-1.74477273547151));
#7849=CARTESIAN_POINT('Ctrl Pts',(18.5375829891438,-44.7151329976084,-1.72079652319878));
#7850=CARTESIAN_POINT('Ctrl Pts',(18.5483955659724,-44.7116778811927,-1.70911489538877));
#7851=CARTESIAN_POINT('Ctrl Pts',(18.5708927433727,-44.7058864158376,-1.68640778762084));
#7852=CARTESIAN_POINT('Ctrl Pts',(18.5825836040364,-44.703545953535,-1.67537312136182));
#7853=CARTESIAN_POINT('Ctrl Pts',(18.6068588448963,-44.6999847326678,-1.65394839029514));
#7854=CARTESIAN_POINT('Ctrl Pts',(18.619445513792,-44.6987636790236,-1.64355633794861));
#7855=CARTESIAN_POINT('Ctrl Pts',(18.645538711709,-44.6974830389479,-1.6234501769643));
#7856=CARTESIAN_POINT('Ctrl Pts',(18.6588325169338,-44.6974335055609,-1.61389957814289));
#7857=CARTESIAN_POINT('Ctrl Pts',(18.6859142215439,-44.6984777777184,-1.59576518307013));
#7858=CARTESIAN_POINT('Ctrl Pts',(18.6997000237853,-44.6995718128947,-1.58718313777874));
#7859=CARTESIAN_POINT('Ctrl Pts',(18.7277631107646,-44.7028992757828,-1.57098989163726));
#7860=CARTESIAN_POINT('Ctrl Pts',(18.7420482463831,-44.705135147643,-1.56337590956548));
#7861=CARTESIAN_POINT('Ctrl Pts',(18.7710946722565,-44.7107644468085,-1.54915862669876));
#7862=CARTESIAN_POINT('Ctrl Pts',(18.7859459094799,-44.7141859522031,-1.54252376800531));
#7863=CARTESIAN_POINT('Ctrl Pts',(18.8156397942149,-44.7221041428292,-1.53052427124137));
#7864=CARTESIAN_POINT('Ctrl Pts',(18.8305728440077,-44.7266157346991,-1.52511234349085));
#7865=CARTESIAN_POINT('Ctrl Pts',(18.860539209484,-44.7367266946174,-1.5155044665792));
#7866=CARTESIAN_POINT('Ctrl Pts',(18.8756508883745,-44.7423612795317,-1.51129385304441));
#7867=CARTESIAN_POINT('Ctrl Pts',(18.9054576403702,-44.7545267829697,-1.50424311881235));
#7868=CARTESIAN_POINT('Ctrl Pts',(18.9202547119906,-44.7610889823919,-1.50136656793277));
#7869=CARTESIAN_POINT('Ctrl Pts',(18.9495825981467,-44.7751396990536,-1.49691920365679));
#7870=CARTESIAN_POINT('Ctrl Pts',(18.9641293094195,-44.7826350228748,-1.49534501613366));
#7871=CARTESIAN_POINT('Ctrl Pts',(18.9857447788442,-44.7945759268798,-1.49397586706081));
#7872=CARTESIAN_POINT('Ctrl Pts',(18.9929278602255,-44.7986804211822,-1.49368555779672));
#7873=CARTESIAN_POINT('Ctrl Pts',(19.0072126126538,-44.8071190824507,-1.49344249033367));
#7874=CARTESIAN_POINT('Ctrl Pts',(19.0143424710875,-44.8114714840967,-1.49349117220706));
#7875=CARTESIAN_POINT('Ctrl Pts',(19.0354329844958,-44.8247714038735,-1.49415091340346));
#7876=CARTESIAN_POINT('Ctrl Pts',(19.0491062136184,-44.8339600939764,-1.49526534883766));
#7877=CARTESIAN_POINT('Ctrl Pts',(19.0757504934149,-44.8529989681212,-1.49881561860667));
#7878=CARTESIAN_POINT('Ctrl Pts',(19.0887128011736,-44.8628432034342,-1.50125064598544));
#7879=CARTESIAN_POINT('Ctrl Pts',(19.1139155845031,-44.8831828996875,-1.50744605367826));
#7880=CARTESIAN_POINT('Ctrl Pts',(19.1261415989452,-44.8936651252513,-1.51120097784455));
#7881=CARTESIAN_POINT('Ctrl Pts',(19.1439645943469,-44.9099328769387,-1.51787676636393));
#7882=CARTESIAN_POINT('Ctrl Pts',(19.1497815019618,-44.9154129298509,-1.5202634684245));
#7883=CARTESIAN_POINT('Ctrl Pts',(19.1611066834579,-44.9264248357533,-1.52532718281113));
#7884=CARTESIAN_POINT('Ctrl Pts',(19.1666295883308,-44.9319700105026,-1.52800963496645));
#7885=CARTESIAN_POINT('Ctrl Pts',(19.182766450003,-44.9487031839457,-1.53649330236943));
#7886=CARTESIAN_POINT('Ctrl Pts',(19.1929633751574,-44.9600013145975,-1.54273516166076));
#7887=CARTESIAN_POINT('Ctrl Pts',(19.2122406126713,-44.9828745059678,-1.55637255063521));
#7888=CARTESIAN_POINT('Ctrl Pts',(19.2213264422722,-44.9944588868497,-1.56377534127668));
#7889=CARTESIAN_POINT('Ctrl Pts',(19.2383462415657,-45.0178815598089,-1.5797264080401));
#7890=CARTESIAN_POINT('Ctrl Pts',(19.2463304771073,-45.0298136028999,-1.58835146880908));
#7891=CARTESIAN_POINT('Ctrl Pts',(19.2607714831931,-45.0534013484058,-1.60637132681278));
#7892=CARTESIAN_POINT('Ctrl Pts',(19.2673038350586,-45.0651515570016,-1.61582546123857));
#7893=CARTESIAN_POINT('Ctrl Pts',(19.2789889194292,-45.0885216379426,-1.63556445143045));
#7894=CARTESIAN_POINT('Ctrl Pts',(19.2841483413751,-45.1001499111597,-1.64585461771952));
#7895=CARTESIAN_POINT('Ctrl Pts',(19.2930976235061,-45.1232965562804,-1.66727425622956));
#7896=CARTESIAN_POINT('Ctrl Pts',(19.2968886296023,-45.1348186371361,-1.67840737565011));
#7897=CARTESIAN_POINT('Ctrl Pts',(19.3030533575681,-45.1577395162296,-1.70152165051547));
#7898=CARTESIAN_POINT('Ctrl Pts',(19.3053753002664,-45.1689424569227,-1.71330457990983));
#7899=CARTESIAN_POINT('Ctrl Pts',(19.3085649502556,-45.1908773666279,-1.73731958680616));
#7900=CARTESIAN_POINT('Ctrl Pts',(19.3094315307921,-45.2016060723277,-1.74954856369043));
#7901=CARTESIAN_POINT('Ctrl Pts',(19.3097256320476,-45.2225959572621,-1.77444163318775));
#7902=CARTESIAN_POINT('Ctrl Pts',(19.3091504322929,-45.2328640131764,-1.78711583153893));
#7903=CARTESIAN_POINT('Ctrl Pts',(19.3065477416738,-45.2529009468769,-1.81286399012433));
#7904=CARTESIAN_POINT('Ctrl Pts',(19.3044916971078,-45.2627436719468,-1.82604582345194));
#7905=CARTESIAN_POINT('Ctrl Pts',(19.2989881366047,-45.2815256556052,-1.8522784706461));
#7906=CARTESIAN_POINT('Ctrl Pts',(19.2955400517893,-45.290535759037,-1.86541441902233));
#7907=CARTESIAN_POINT('Ctrl Pts',(19.2872838742066,-45.3077809202632,-1.89168343393709));
#7908=CARTESIAN_POINT('Ctrl Pts',(19.2824758531213,-45.3160216986954,-1.90482330786193));
#7909=CARTESIAN_POINT('Ctrl Pts',(19.2714947564013,-45.3317383217991,-1.93111314012225));
#7910=CARTESIAN_POINT('Ctrl Pts',(19.2653276103518,-45.3392082270028,-1.94425196045163));
#7911=CARTESIAN_POINT('Ctrl Pts',(19.2515609423283,-45.3533830770125,-1.97058421507986));
#7912=CARTESIAN_POINT('Ctrl Pts',(19.244064213872,-45.3599773095852,-1.98357519226534));
#7913=CARTESIAN_POINT('Ctrl Pts',(19.2279384887284,-45.3721611568294,-2.00912118369974));
#7914=CARTESIAN_POINT('Ctrl Pts',(19.2192997653202,-45.37776054843,-2.02169452303134));
#7915=CARTESIAN_POINT('Ctrl Pts',(19.2008823814414,-45.3879779405028,-2.04643994358655));
#7916=CARTESIAN_POINT('Ctrl Pts',(19.1910930202263,-45.3925988298126,-2.05862275579914));
#7917=CARTESIAN_POINT('Ctrl Pts',(19.1703915953673,-45.4008287111318,-2.08254175691223));
#7918=CARTESIAN_POINT('Ctrl Pts',(19.1593769020686,-45.4044612308546,-2.09437589174056));
#7919=CARTESIAN_POINT('Ctrl Pts',(19.1365984286433,-45.4105559999369,-2.11715811641161));
#7920=CARTESIAN_POINT('Ctrl Pts',(19.1247946980441,-45.4130446424486,-2.12816493034605));
#7921=CARTESIAN_POINT('Ctrl Pts',(19.1003849579208,-45.4169112106896,-2.14940462118797));
#7922=CARTESIAN_POINT('Ctrl Pts',(19.0877771726989,-45.4182909661987,-2.15964088112869));
#7923=CARTESIAN_POINT('Ctrl Pts',(19.0617491248472,-45.4199293752183,-2.17933956376603));
#7924=CARTESIAN_POINT('Ctrl Pts',(19.0483317526372,-45.4201882850831,-2.1888003047611));
#7925=CARTESIAN_POINT('Ctrl Pts',(19.0206432686844,-45.4195375776723,-2.20692604496228));
#7926=CARTESIAN_POINT('Ctrl Pts',(19.0065974658149,-45.418632682757,-2.21544292771705));
#7927=CARTESIAN_POINT('Ctrl Pts',(18.9781346138199,-45.415695036091,-2.23140600796168));
#7928=CARTESIAN_POINT('Ctrl Pts',(18.9637143613756,-45.4136621054362,-2.23885416694541));
#7929=CARTESIAN_POINT('Ctrl Pts',(18.9344985968864,-45.4084658423515,-2.25268578324637));
#7930=CARTESIAN_POINT('Ctrl Pts',(18.9196997691129,-45.4053010066314,-2.25906973315595));
#7931=CARTESIAN_POINT('Ctrl Pts',(18.8972234079784,-45.399684523811,-2.26782447509019));
#7932=CARTESIAN_POINT('Ctrl Pts',(18.8896670993892,-45.3976611130282,-2.27061057640927));
#7933=CARTESIAN_POINT('Ctrl Pts',(18.8745247920546,-45.3933350465311,-2.27587916719238));
#7934=CARTESIAN_POINT('Ctrl Pts',(18.86697271241,-45.3910428501848,-2.27835075020622));
#7935=CARTESIAN_POINT('Ctrl Pts',(18.8443734352162,-45.3837824914105,-2.28528292905637));
#7936=CARTESIAN_POINT('Ctrl Pts',(18.8293452614729,-45.3784237192965,-2.28927880462709));
#7937=CARTESIAN_POINT('Ctrl Pts',(18.8143835621595,-45.3725581651887,-2.29264601963605));
#7938=CARTESIAN_POINT('Ctrl Pts',(18.6221620196843,-45.62059505756,-1.77871850124803));
#7939=CARTESIAN_POINT('Ctrl Pts',(18.6129193730699,-45.6172932558704,-1.78058192917525));
#7940=CARTESIAN_POINT('Ctrl Pts',(18.6037208544611,-45.6136589591554,-1.78208130646566));
#7941=CARTESIAN_POINT('Ctrl Pts',(18.5900102210826,-45.6077105512134,-1.78377425389336));
#7942=CARTESIAN_POINT('Ctrl Pts',(18.5854465361298,-45.6056405946596,-1.78424599704345));
#7943=CARTESIAN_POINT('Ctrl Pts',(18.576354527559,-45.6013345885701,-1.78500009038837));
#7944=CARTESIAN_POINT('Ctrl Pts',(18.5718108421278,-45.5990902159595,-1.78528264628693));
#7945=CARTESIAN_POINT('Ctrl Pts',(18.5583557915536,-45.592164749705,-1.78583455232009));
#7946=CARTESIAN_POINT('Ctrl Pts',(18.549597268328,-45.5872853986604,-1.78581522368785));
#7947=CARTESIAN_POINT('Ctrl Pts',(18.5324696592232,-45.5770009406535,-1.78502001129054));
#7948=CARTESIAN_POINT('Ctrl Pts',(18.5241044984817,-45.5715981948212,-1.7842443140869));
#7949=CARTESIAN_POINT('Ctrl Pts',(18.5077731763177,-45.560269424572,-1.78193347961354));
#7950=CARTESIAN_POINT('Ctrl Pts',(18.4998161446777,-45.554350730268,-1.78040065085215));
#7951=CARTESIAN_POINT('Ctrl Pts',(18.4881626129628,-45.5450449208074,-1.77750557246982));
#7952=CARTESIAN_POINT('Ctrl Pts',(18.4843505062967,-45.54189107573,-1.77644663525675));
#7953=CARTESIAN_POINT('Ctrl Pts',(18.4769071413954,-45.5355132808845,-1.77415492247898));
#7954=CARTESIAN_POINT('Ctrl Pts',(18.4732672288629,-45.5322824364064,-1.77292001334332));
#7955=CARTESIAN_POINT('Ctrl Pts',(18.4626004022307,-45.5224752605349,-1.7689552464585));
#7956=CARTESIAN_POINT('Ctrl Pts',(18.4558179103171,-45.5157781683263,-1.76596391369291));
#7957=CARTESIAN_POINT('Ctrl Pts',(18.4429084062604,-45.5020723540079,-1.75929249956289));
#7958=CARTESIAN_POINT('Ctrl Pts',(18.4367785698554,-45.4950591040281,-1.75560939899404));
#7959=CARTESIAN_POINT('Ctrl Pts',(18.4251947575442,-45.4807293651287,-1.74755147248085));
#7960=CARTESIAN_POINT('Ctrl Pts',(18.4197116844311,-45.4733619559223,-1.74314118482812));
#7961=CARTESIAN_POINT('Ctrl Pts',(18.4096841967476,-45.4586601759361,-1.73382309642942));
#7962=CARTESIAN_POINT('Ctrl Pts',(18.4050855722086,-45.4512635702888,-1.72888250720206));
#7963=CARTESIAN_POINT('Ctrl Pts',(18.3967294933308,-45.4364159601022,-1.71846981786302));
#7964=CARTESIAN_POINT('Ctrl Pts',(18.3929666633764,-45.4289582747971,-1.71299394688883));
#7965=CARTESIAN_POINT('Ctrl Pts',(18.387949845685,-45.4177241224448,-1.7043764995696));
#7966=CARTESIAN_POINT('Ctrl Pts',(18.3863815973451,-45.4139692966578,-1.70143483928496));
#7967=CARTESIAN_POINT('Ctrl Pts',(18.3834588294126,-45.4064475115089,-1.69541819155667));
#7968=CARTESIAN_POINT('Ctrl Pts',(18.3821013440093,-45.4026715013318,-1.69233565252243));
#7969=CARTESIAN_POINT('Ctrl Pts',(18.3783678140288,-45.3913602280059,-1.68291331926215));
#7970=CARTESIAN_POINT('Ctrl Pts',(18.3763571442371,-45.3839334687444,-1.67647740418325));
#7971=CARTESIAN_POINT('Ctrl Pts',(18.373239274455,-45.3692470015761,-1.66326464104222));
#7972=CARTESIAN_POINT('Ctrl Pts',(18.3721351020341,-45.361996292618,-1.65649525672691));
#7973=CARTESIAN_POINT('Ctrl Pts',(18.3708276406403,-45.3476781657535,-1.64263357999033));
#7974=CARTESIAN_POINT('Ctrl Pts',(18.3706250612,-45.3406095748083,-1.635539689768));
#7975=CARTESIAN_POINT('Ctrl Pts',(18.3710077529534,-45.3301503262564,-1.62465679749559));
#7976=CARTESIAN_POINT('Ctrl Pts',(18.3712517326172,-45.3266799167243,-1.62097960829253));
#7977=CARTESIAN_POINT('Ctrl Pts',(18.3719701704098,-45.3198204005466,-1.61357771003206));
#7978=CARTESIAN_POINT('Ctrl Pts',(18.3724424090973,-45.3164453844991,-1.60986862656259));
#7979=CARTESIAN_POINT('Ctrl Pts',(18.3741925883538,-45.3064826315517,-1.59871817096884));
#7980=CARTESIAN_POINT('Ctrl Pts',(18.3758024868939,-45.300037895571,-1.59123476923353));
#7981=CARTESIAN_POINT('Ctrl Pts',(18.3798873333543,-45.287560207475,-1.57619835335595));
#7982=CARTESIAN_POINT('Ctrl Pts',(18.3823625923558,-45.2815224282728,-1.56864024051346));
#7983=CARTESIAN_POINT('Ctrl Pts',(18.3881814606797,-45.2698526364099,-1.55344639789905));
#7984=CARTESIAN_POINT('Ctrl Pts',(18.3915297734654,-45.2642137421464,-1.54580098849944));
#7985=CARTESIAN_POINT('Ctrl Pts',(18.3991069351451,-45.2533791834234,-1.53046386154549));
#7986=CARTESIAN_POINT('Ctrl Pts',(18.4032741386649,-45.2482681928533,-1.52289338059093));
#7987=CARTESIAN_POINT('Ctrl Pts',(18.4123563475389,-45.2386112685697,-1.50790546647126));
#7988=CARTESIAN_POINT('Ctrl Pts',(18.4172683983267,-45.2340697519755,-1.50049420992322));
#7989=CARTESIAN_POINT('Ctrl Pts',(18.4278282750222,-45.2255558775991,-1.48583573393937));
#7990=CARTESIAN_POINT('Ctrl Pts',(18.4334801703118,-45.2215821677685,-1.47858483274337));
#7991=CARTESIAN_POINT('Ctrl Pts',(18.4455181297567,-45.2142206641317,-1.46426506544444));
#7992=CARTESIAN_POINT('Ctrl Pts',(18.4519528219293,-45.2108157610502,-1.45715123177322));
#7993=CARTESIAN_POINT('Ctrl Pts',(18.4652968721977,-45.2047449038404,-1.44340852007555));
#7994=CARTESIAN_POINT('Ctrl Pts',(18.4722504447086,-45.2020474267363,-1.43672247316454));
#7995=CARTESIAN_POINT('Ctrl Pts',(18.4866860257431,-45.1973329645429,-1.42374529115857));
#7996=CARTESIAN_POINT('Ctrl Pts',(18.4941721105413,-45.1953130577611,-1.41744886968267));
#7997=CARTESIAN_POINT('Ctrl Pts',(18.5096858061187,-45.1919542156582,-1.40524401960937));
#7998=CARTESIAN_POINT('Ctrl Pts',(18.5177148817011,-45.1906149853657,-1.39933446124003));
#7999=CARTESIAN_POINT('Ctrl Pts',(18.5343294229057,-45.1886445172451,-1.38792248147468));
#8000=CARTESIAN_POINT('Ctrl Pts',(18.542779440216,-45.188029106266,-1.38251285316967));
#8001=CARTESIAN_POINT('Ctrl Pts',(18.5599645231716,-45.1875150185148,-1.37226320603098));
#8002=CARTESIAN_POINT('Ctrl Pts',(18.5686982527055,-45.1876165784289,-1.36742418470241));
#8003=CARTESIAN_POINT('Ctrl Pts',(18.5864477638643,-45.1885360827692,-1.35831709053276));
#8004=CARTESIAN_POINT('Ctrl Pts',(18.5954684722606,-45.1893552624518,-1.35404748924571));
#8005=CARTESIAN_POINT('Ctrl Pts',(18.6137800334896,-45.1917248752601,-1.34610113724339));
#8006=CARTESIAN_POINT('Ctrl Pts',(18.6231272825575,-45.1932895780203,-1.34240702291553));
#8007=CARTESIAN_POINT('Ctrl Pts',(18.6417841046389,-45.1971209486494,-1.33575597841215));
#8008=CARTESIAN_POINT('Ctrl Pts',(18.6511507406784,-45.1993932961657,-1.33277254722322));
#8009=CARTESIAN_POINT('Ctrl Pts',(18.6699132468501,-45.204646120538,-1.32751128947911));
#8010=CARTESIAN_POINT('Ctrl Pts',(18.6793578875184,-45.207646105241,-1.32522575676464));
#8011=CARTESIAN_POINT('Ctrl Pts',(18.6979513544394,-45.214255255135,-1.32144333958208));
#8012=CARTESIAN_POINT('Ctrl Pts',(18.7071641468385,-45.2178802413143,-1.31992638960479));
#8013=CARTESIAN_POINT('Ctrl Pts',(18.7253869486455,-45.225754682879,-1.31764408095801));
#8014=CARTESIAN_POINT('Ctrl Pts',(18.7344068621661,-45.2300078746987,-1.316876927761));
#8015=CARTESIAN_POINT('Ctrl Pts',(18.7477801983432,-45.2368600692891,-1.31629654325037));
#8016=CARTESIAN_POINT('Ctrl Pts',(18.752219283311,-45.2392274939513,-1.31619867106209));
#8017=CARTESIAN_POINT('Ctrl Pts',(18.7610367701067,-45.2441187387261,-1.31619676023362));
#8018=CARTESIAN_POINT('Ctrl Pts',(18.7654325107433,-45.2466532619187,-1.3162938241929));
#8019=CARTESIAN_POINT('Ctrl Pts',(18.7784191500246,-45.2544329831877,-1.31687816890436));
#8020=CARTESIAN_POINT('Ctrl Pts',(18.7868169502624,-45.2598527540315,-1.31765275683562));
#8021=CARTESIAN_POINT('Ctrl Pts',(18.8031371766128,-45.2711680622823,-1.31995614213438));
#8022=CARTESIAN_POINT('Ctrl Pts',(18.8110542369534,-45.2770600838242,-1.3214843906258));
#8023=CARTESIAN_POINT('Ctrl Pts',(18.8264003541456,-45.2893146918086,-1.32529693961078));
#8024=CARTESIAN_POINT('Ctrl Pts',(18.8338206659933,-45.2956692062439,-1.32757795725868));
#8025=CARTESIAN_POINT('Ctrl Pts',(18.8445991939612,-45.3055898547247,-1.33159522925254));
#8026=CARTESIAN_POINT('Ctrl Pts',(18.8481102922723,-45.308941341363,-1.3330260675456));
#8027=CARTESIAN_POINT('Ctrl Pts',(18.8549328043703,-45.3156945009062,-1.33605192943852));
#8028=CARTESIAN_POINT('Ctrl Pts',(18.8582530677542,-45.3191042958294,-1.33765022769154));
#8029=CARTESIAN_POINT('Ctrl Pts',(18.867933585062,-45.3294204870494,-1.34269225948157));
#8030=CARTESIAN_POINT('Ctrl Pts',(18.8740225584048,-45.336421260905,-1.34638576214841));
#8031=CARTESIAN_POINT('Ctrl Pts',(18.8854757967299,-45.3506622005078,-1.35442702575445));
#8032=CARTESIAN_POINT('Ctrl Pts',(18.8908432353629,-45.3579082824918,-1.35877902402508));
#8033=CARTESIAN_POINT('Ctrl Pts',(18.9008330792294,-45.3726243827529,-1.36813301959756));
#8034=CARTESIAN_POINT('Ctrl Pts',(18.9054840795676,-45.380154146016,-1.37317976216689));
#8035=CARTESIAN_POINT('Ctrl Pts',(18.9138227526446,-45.3951016039498,-1.38370412631569));
#8036=CARTESIAN_POINT('Ctrl Pts',(18.9175551433971,-45.4025783442055,-1.38921665563984));
#8037=CARTESIAN_POINT('Ctrl Pts',(18.9241472981129,-45.4175069410417,-1.40071017489184));
#8038=CARTESIAN_POINT('Ctrl Pts',(18.9270110154327,-45.4249640522584,-1.40669428620247));
#8039=CARTESIAN_POINT('Ctrl Pts',(18.9318734081378,-45.4398636906155,-1.41913718051563));
#8040=CARTESIAN_POINT('Ctrl Pts',(18.9338726776514,-45.4473086206934,-1.42559807779935));
#8041=CARTESIAN_POINT('Ctrl Pts',(18.9369783416384,-45.4621742438128,-1.4390004513004));
#8042=CARTESIAN_POINT('Ctrl Pts',(18.9380587854086,-45.4694678481601,-1.44582700875946));
#8043=CARTESIAN_POINT('Ctrl Pts',(18.9393173410065,-45.4838003767252,-1.45973104908589));
#8044=CARTESIAN_POINT('Ctrl Pts',(18.9394948496878,-45.4908371992824,-1.46680673001694));
#8045=CARTESIAN_POINT('Ctrl Pts',(18.9389586363646,-45.504655487356,-1.4812020445518));
#8046=CARTESIAN_POINT('Ctrl Pts',(18.9382429617193,-45.5114415845077,-1.48852750652597));
#8047=CARTESIAN_POINT('Ctrl Pts',(18.935914549752,-45.5247359862846,-1.5034028039268));
#8048=CARTESIAN_POINT('Ctrl Pts',(18.9342813020382,-45.5312939444273,-1.51101488314489));
#8049=CARTESIAN_POINT('Ctrl Pts',(18.9301711295785,-45.543861814362,-1.52615759875804));
#8050=CARTESIAN_POINT('Ctrl Pts',(18.9276914024776,-45.5499184342165,-1.53373745384419));
#8051=CARTESIAN_POINT('Ctrl Pts',(18.9219044584414,-45.5615659591846,-1.5488905221349));
#8052=CARTESIAN_POINT('Ctrl Pts',(18.9185970863043,-45.5671606360396,-1.55646766958521));
#8053=CARTESIAN_POINT('Ctrl Pts',(18.9111518540018,-45.5778903308794,-1.5716231951062));
#8054=CARTESIAN_POINT('Ctrl Pts',(18.9070179238834,-45.5830212371186,-1.57919515593537));
#8055=CARTESIAN_POINT('Ctrl Pts',(18.8978775137544,-45.5928252580521,-1.59436601615716));
#8056=CARTESIAN_POINT('Ctrl Pts',(18.8929394538017,-45.5974219543871,-1.60184826399308));
#8057=CARTESIAN_POINT('Ctrl Pts',(18.8823875119263,-45.6059897116602,-1.61655719916668));
#8058=CARTESIAN_POINT('Ctrl Pts',(18.8767671790069,-45.6099675442075,-1.62379444292518));
#8059=CARTESIAN_POINT('Ctrl Pts',(18.8648446796018,-45.6173136869872,-1.63803320411293));
#8060=CARTESIAN_POINT('Ctrl Pts',(18.8585356910874,-45.620684256901,-1.645040886683));
#8061=CARTESIAN_POINT('Ctrl Pts',(18.8452471260023,-45.6267961002234,-1.65879399575824));
#8062=CARTESIAN_POINT('Ctrl Pts',(18.8382022586574,-45.629556299998,-1.66559567268411));
#8063=CARTESIAN_POINT('Ctrl Pts',(18.8236812226873,-45.6343318803847,-1.67868354354709));
#8064=CARTESIAN_POINT('Ctrl Pts',(18.816179049323,-45.6363659793353,-1.68500354300762));
#8065=CARTESIAN_POINT('Ctrl Pts',(18.8007069179842,-45.6397318406192,-1.69719202919393));
#8066=CARTESIAN_POINT('Ctrl Pts',(18.7927357842832,-45.6410648637206,-1.70306246701553));
#8067=CARTESIAN_POINT('Ctrl Pts',(18.7763184849427,-45.6430238072,-1.7143510708677));
#8068=CARTESIAN_POINT('Ctrl Pts',(18.7678741313109,-45.643649793127,-1.7197682782934));
#8069=CARTESIAN_POINT('Ctrl Pts',(18.750484658679,-45.6441668837513,-1.73013665595371));
#8070=CARTESIAN_POINT('Ctrl Pts',(18.7416810490484,-45.6440534227969,-1.7350030871688));
#8071=CARTESIAN_POINT('Ctrl Pts',(18.7238738472453,-45.6431037361945,-1.74411204981961));
#8072=CARTESIAN_POINT('Ctrl Pts',(18.7148682493225,-45.6422674984819,-1.74835570404536));
#8073=CARTESIAN_POINT('Ctrl Pts',(18.6966533086483,-45.6398726569234,-1.75622164832084));
#8074=CARTESIAN_POINT('Ctrl Pts',(18.6874419268025,-45.6383131841139,-1.75984420616735));
#8075=CARTESIAN_POINT('Ctrl Pts',(18.6734737700129,-45.6354195819173,-1.76479817562067));
#8076=CARTESIAN_POINT('Ctrl Pts',(18.6687815047508,-45.6343591081953,-1.76637215337371));
#8077=CARTESIAN_POINT('Ctrl Pts',(18.6593857582353,-45.6320583062489,-1.76934304099513));
#8078=CARTESIAN_POINT('Ctrl Pts',(18.6547033024031,-45.6308236309591,-1.77073381700843));
#8079=CARTESIAN_POINT('Ctrl Pts',(18.6407016991349,-45.6268695302727,-1.77462522039306));
#8080=CARTESIAN_POINT('Ctrl Pts',(18.6314046662986,-45.6238968592495,-1.77685507332082));
#8081=CARTESIAN_POINT('Ctrl Pts',(18.6221620196843,-45.62059505756,-1.77871850124803));
#8082=CARTESIAN_POINT('Ctrl Pts',(18.8143835720322,-45.3725581690592,-2.29264601741413));
#8083=CARTESIAN_POINT('Ctrl Pts',(18.8004239876014,-45.3670854822463,-2.29578770105548));
#8084=CARTESIAN_POINT('Ctrl Pts',(18.7868223091714,-45.3612925527447,-2.29831830851143));
#8085=CARTESIAN_POINT('Ctrl Pts',(18.7734632629,-45.3551737210001,-2.30031107484356));
#8086=CARTESIAN_POINT('Ctrl Pts',(18.7721970853537,-45.3545937748568,-2.30049995030169));
#8087=CARTESIAN_POINT('Ctrl Pts',(18.7709330877609,-45.3540108759632,-2.30068396486783));
#8088=CARTESIAN_POINT('Ctrl Pts',(18.7696711723614,-45.3534250039398,-2.30086316260009));
#8089=CARTESIAN_POINT('Ctrl Pts',(18.7622047899902,-45.3499585714448,-2.30192342289145));
#8090=CARTESIAN_POINT('Ctrl Pts',(18.7547981841974,-45.346380911665,-2.30281570621072));
#8091=CARTESIAN_POINT('Ctrl Pts',(18.747446675797,-45.3426929858494,-2.30354453863187));
#8092=CARTESIAN_POINT('Ctrl Pts',(18.7400309651229,-45.3389728525998,-2.30427973610029));
#8093=CARTESIAN_POINT('Ctrl Pts',(18.7326462625095,-45.3351263544063,-2.30484927334382));
#8094=CARTESIAN_POINT('Ctrl Pts',(18.7253607974182,-45.3311904062177,-2.30524970736628));
#8095=CARTESIAN_POINT('Ctrl Pts',(18.7123145848033,-45.3241422334153,-2.3059667717307));
#8096=CARTESIAN_POINT('Ctrl Pts',(18.6995547694162,-45.3167993788134,-2.3061540494447));
#8097=CARTESIAN_POINT('Ctrl Pts',(18.6869391162223,-45.3090816154315,-2.30581663077418));
#8098=CARTESIAN_POINT('Ctrl Pts',(18.6854534455579,-45.3081727402051,-2.30577689497828));
#8099=CARTESIAN_POINT('Ctrl Pts',(18.6839697956892,-45.3072586368875,-2.30572983528853));
#8100=CARTESIAN_POINT('Ctrl Pts',(18.6824879511072,-45.3063391513267,-2.30567542238217));
#8101=CARTESIAN_POINT('Ctrl Pts',(18.6722737305609,-45.3000012206008,-2.3053003591449));
#8102=CARTESIAN_POINT('Ctrl Pts',(18.6621479860631,-45.2934106165849,-2.30457758487901));
#8103=CARTESIAN_POINT('Ctrl Pts',(18.6520560907276,-45.286510756581,-2.30347965695592));
#8104=CARTESIAN_POINT('Ctrl Pts',(18.6484920955429,-45.2840740420678,-2.30309191910282));
#8105=CARTESIAN_POINT('Ctrl Pts',(18.6449539352567,-45.2816133646422,-2.30265953234694));
#8106=CARTESIAN_POINT('Ctrl Pts',(18.6414409530944,-45.2791285251635,-2.30218272861357));
#8107=CARTESIAN_POINT('Ctrl Pts',(18.628011060722,-45.2696291524881,-2.30035994030265));
#8108=CARTESIAN_POINT('Ctrl Pts',(18.6149637231189,-45.2597892538428,-2.29789258754658));
#8109=CARTESIAN_POINT('Ctrl Pts',(18.6022294924165,-45.2495457329913,-2.29475584752329));
#8110=CARTESIAN_POINT('Ctrl Pts',(18.5958359434542,-45.2444027091494,-2.29318096629256));
#8111=CARTESIAN_POINT('Ctrl Pts',(18.589563243215,-45.2391901429808,-2.29144593577685));
#8112=CARTESIAN_POINT('Ctrl Pts',(18.5834369872997,-45.2339331804978,-2.28956226538368));
#8113=CARTESIAN_POINT('Ctrl Pts',(18.5773027399217,-45.2286693605116,-2.28767613781572));
#8114=CARTESIAN_POINT('Ctrl Pts',(18.5713010530664,-45.2233495740206,-2.28563749245308));
#8115=CARTESIAN_POINT('Ctrl Pts',(18.5654325544997,-45.2179770224707,-2.28344953823052));
#8116=CARTESIAN_POINT('Ctrl Pts',(18.553698651473,-45.2072347519946,-2.27907478336218));
#8117=CARTESIAN_POINT('Ctrl Pts',(18.542482749313,-45.1962715684224,-2.27410148247452));
#8118=CARTESIAN_POINT('Ctrl Pts',(18.5317611930651,-45.185066998578,-2.26852163941299));
#8119=CARTESIAN_POINT('Ctrl Pts',(18.5265356102954,-45.1796059996551,-2.26580207789727));
#8120=CARTESIAN_POINT('Ctrl Pts',(18.5214264579813,-45.1740858650027,-2.26293705907253));
#8121=CARTESIAN_POINT('Ctrl Pts',(18.5164344168917,-45.1685050515947,-2.2599242470794));
#8122=CARTESIAN_POINT('Ctrl Pts',(18.5112098007234,-45.1626642326909,-2.25677107065937));
#8123=CARTESIAN_POINT('Ctrl Pts',(18.5061284176769,-45.1567736219033,-2.25346498673654));
#8124=CARTESIAN_POINT('Ctrl Pts',(18.5011909625963,-45.1508342975478,-2.25000661864255));
#8125=CARTESIAN_POINT('Ctrl Pts',(18.491508410506,-45.1391870386839,-2.24322461684791));
#8126=CARTESIAN_POINT('Ctrl Pts',(18.4823299625097,-45.1272711143548,-2.23579736542041));
#8127=CARTESIAN_POINT('Ctrl Pts',(18.4739101995274,-45.1154323141895,-2.22794676536405));
#8128=CARTESIAN_POINT('Ctrl Pts',(18.4654702471985,-45.103565126332,-2.2200773407296));
#8129=CARTESIAN_POINT('Ctrl Pts',(18.4577018487684,-45.091673400839,-2.21172713083511));
#8130=CARTESIAN_POINT('Ctrl Pts',(18.4506043254293,-45.0797770058834,-2.20291734912335));
#8131=CARTESIAN_POINT('Ctrl Pts',(18.4435022248184,-45.0678729388103,-2.19410188588521));
#8132=CARTESIAN_POINT('Ctrl Pts',(18.4370628910371,-45.0559533293678,-2.18481990262873));
#8133=CARTESIAN_POINT('Ctrl Pts',(18.4312854178286,-45.0440123208978,-2.17506295044399));
#8134=CARTESIAN_POINT('Ctrl Pts',(18.4283984600337,-45.0380454931449,-2.17018747839114));
#8135=CARTESIAN_POINT('Ctrl Pts',(18.4256758338712,-45.0320698970282,-2.1651901129344));
#8136=CARTESIAN_POINT('Ctrl Pts',(18.4231219961346,-45.0260908918466,-2.16007363253705));
#8137=CARTESIAN_POINT('Ctrl Pts',(18.4205706988703,-45.0201178343793,-2.15496224184333));
#8138=CARTESIAN_POINT('Ctrl Pts',(18.418182587299,-45.0141270383902,-2.14971911935779));
#8139=CARTESIAN_POINT('Ctrl Pts',(18.4159733552971,-45.0081503497711,-2.14436973787106));
#8140=CARTESIAN_POINT('Ctrl Pts',(18.4115653077667,-44.9962251524691,-2.13369619709656));
#8141=CARTESIAN_POINT('Ctrl Pts',(18.4079166371414,-44.9845006989954,-2.12273326060535));
#8142=CARTESIAN_POINT('Ctrl Pts',(18.4049873524301,-44.9729204300536,-2.11144045659183));
#8143=CARTESIAN_POINT('Ctrl Pts',(18.4020714181278,-44.9613929389545,-2.1001991202805));
#8144=CARTESIAN_POINT('Ctrl Pts',(18.3998736076026,-44.9500224126483,-2.08864349710599));
#8145=CARTESIAN_POINT('Ctrl Pts',(18.3983959092214,-44.9388017294662,-2.07676095428626));
#8146=CARTESIAN_POINT('Ctrl Pts',(18.3969534133881,-44.9278483516032,-2.06516148397203));
#8147=CARTESIAN_POINT('Ctrl Pts',(18.3961981046829,-44.9170360420461,-2.05324784150275));
#8148=CARTESIAN_POINT('Ctrl Pts',(18.3961530998036,-44.9063694860149,-2.04100636176672));
#8149=CARTESIAN_POINT('Ctrl Pts',(18.3961522869288,-44.9061768274623,-2.04078525705771));
#8150=CARTESIAN_POINT('Ctrl Pts',(18.3961517065425,-44.9059843646424,-2.04056421547236));
#8151=CARTESIAN_POINT('Ctrl Pts',(18.3961513577277,-44.9057920947054,-2.040343234352));
#8152=CARTESIAN_POINT('Ctrl Pts',(18.3961413899904,-44.9002977855887,-2.03402847395322));
#8153=CARTESIAN_POINT('Ctrl Pts',(18.3963218076041,-44.8949486379762,-2.02774797606833));
#8154=CARTESIAN_POINT('Ctrl Pts',(18.3966783095951,-44.8897170364107,-2.02147951930314));
#8155=CARTESIAN_POINT('Ctrl Pts',(18.3970409778534,-44.8843949459994,-2.01510263963699));
#8156=CARTESIAN_POINT('Ctrl Pts',(18.3975832129578,-44.879215584956,-2.00876434096866));
#8157=CARTESIAN_POINT('Ctrl Pts',(18.3983054323315,-44.8741136640234,-2.00238878355093));
#8158=CARTESIAN_POINT('Ctrl Pts',(18.3992264158328,-44.867607628357,-1.99425859013933));
#8159=CARTESIAN_POINT('Ctrl Pts',(18.4004372205309,-44.861214582528,-1.98605493790166));
#8160=CARTESIAN_POINT('Ctrl Pts',(18.4019814199691,-44.8548256801295,-1.97762112291159));
#8161=CARTESIAN_POINT('Ctrl Pts',(18.4024376090313,-44.8529382636973,-1.97512959619772));
#8162=CARTESIAN_POINT('Ctrl Pts',(18.4029231971869,-44.8510513677406,-1.97261795136468));
#8163=CARTESIAN_POINT('Ctrl Pts',(18.403440078478,-44.8491626004708,-1.97008207935643));
#8164=CARTESIAN_POINT('Ctrl Pts',(18.4038588959962,-44.8476321739806,-1.96802731815887));
#8165=CARTESIAN_POINT('Ctrl Pts',(18.4043018647573,-44.8460878557025,-1.96593952534612));
#8166=CARTESIAN_POINT('Ctrl Pts',(18.4047663150324,-44.8445433944683,-1.96383639013916));
#8167=CARTESIAN_POINT('Ctrl Pts',(18.4059382132851,-44.8406464187982,-1.9585297715262));
#8168=CARTESIAN_POINT('Ctrl Pts',(18.4072504491973,-44.836749090789,-1.95312358986634));
#8169=CARTESIAN_POINT('Ctrl Pts',(18.4086264109651,-44.8330535376181,-1.94790428743763));
#8170=CARTESIAN_POINT('Ctrl Pts',(18.409982715073,-44.8294107809196,-1.94275955050535));
#8171=CARTESIAN_POINT('Ctrl Pts',(18.4114002396028,-44.825963730331,-1.93779647790292));
#8172=CARTESIAN_POINT('Ctrl Pts',(18.4127613885304,-44.8228831621709,-1.93329453562058));
#8173=CARTESIAN_POINT('Ctrl Pts',(18.4136001434265,-44.8209848822878,-1.9305203894159));
#8174=CARTESIAN_POINT('Ctrl Pts',(18.414487376004,-44.8190644191933,-1.92768639394373));
#8175=CARTESIAN_POINT('Ctrl Pts',(18.4154262847733,-44.8171251875568,-1.92479418624063));
#8176=CARTESIAN_POINT('Ctrl Pts',(18.4181694429729,-44.8114594409591,-1.916344181793));
#8177=CARTESIAN_POINT('Ctrl Pts',(18.4213570016482,-44.8056288168499,-1.90738961609199));
#8178=CARTESIAN_POINT('Ctrl Pts',(18.425067403476,-44.7997293148395,-1.89798447547152));
#8179=CARTESIAN_POINT('Ctrl Pts',(18.4267071356894,-44.7971221569254,-1.89382807604023));
#8180=CARTESIAN_POINT('Ctrl Pts',(18.4284458771357,-44.7945059656841,-1.88959094729095));
#8181=CARTESIAN_POINT('Ctrl Pts',(18.4302982493404,-44.7918774552728,-1.88525884485412));
#8182=CARTESIAN_POINT('Ctrl Pts',(18.4312589896668,-44.7905141677304,-1.88301198242625));
#8183=CARTESIAN_POINT('Ctrl Pts',(18.4322476807013,-44.7891512009799,-1.88074559978552));
#8184=CARTESIAN_POINT('Ctrl Pts',(18.4332663774496,-44.7877881173523,-1.87845772299634));
#8185=CARTESIAN_POINT('Ctrl Pts',(18.43459451111,-44.7860109866696,-1.87547488617116));
#8186=CARTESIAN_POINT('Ctrl Pts',(18.4360905916004,-44.7840843386202,-1.87220096972747));
#8187=CARTESIAN_POINT('Ctrl Pts',(18.437552740056,-44.7822772399823,-1.86908824391098));
#8188=CARTESIAN_POINT('Ctrl Pts',(18.4391864896795,-44.780258056015,-1.86561020130088));
#8189=CARTESIAN_POINT('Ctrl Pts',(18.4407777072385,-44.7783878950342,-1.86233324968192));
#8190=CARTESIAN_POINT('Ctrl Pts',(18.4419912296012,-44.7769984935751,-1.85987648243287));
#8191=CARTESIAN_POINT('Ctrl Pts',(18.4421307944011,-44.7768387012692,-1.85959393450455));
#8192=CARTESIAN_POINT('Ctrl Pts',(18.4422653209045,-44.7766852340587,-1.85932222665245));
#8193=CARTESIAN_POINT('Ctrl Pts',(18.4423942727962,-44.7765385757179,-1.85906229563845));
#8194=CARTESIAN_POINT('Ctrl Pts',(18.4442993095736,-44.7743719573813,-1.85522227332556));
#8195=CARTESIAN_POINT('Ctrl Pts',(18.4464978127059,-44.7719689214077,-1.85090212076217));
#8196=CARTESIAN_POINT('Ctrl Pts',(18.4491297065906,-44.7692782255981,-1.84594334195215));
#8197=CARTESIAN_POINT('Ctrl Pts',(18.4515807522943,-44.7667724184899,-1.84132530109245));
#8198=CARTESIAN_POINT('Ctrl Pts',(18.4544067332379,-44.7640174757803,-1.83615446044127));
#8199=CARTESIAN_POINT('Ctrl Pts',(18.4577529093881,-44.7609994330517,-1.83031111945421));
#8200=CARTESIAN_POINT('Ctrl Pts',(18.4593149008355,-44.7595906139345,-1.82758345413227));
#8201=CARTESIAN_POINT('Ctrl Pts',(18.4609907570087,-44.7581248818874,-1.82470935927919));
#8202=CARTESIAN_POINT('Ctrl Pts',(18.4627983272808,-44.7566033146199,-1.8216773121477));
#8203=CARTESIAN_POINT('Ctrl Pts',(18.465907725695,-44.7539859011107,-1.81646155777946));
#8204=CARTESIAN_POINT('Ctrl Pts',(18.468851062055,-44.7516706279046,-1.81171012416722));
#8205=CARTESIAN_POINT('Ctrl Pts',(18.4715899190303,-44.7496144243376,-1.80740112264175));
#8206=CARTESIAN_POINT('Ctrl Pts',(18.4755934405833,-44.7466087707485,-1.80110244380068));
#8207=CARTESIAN_POINT('Ctrl Pts',(18.4791597997392,-44.7441550963149,-1.79574749180543));
#8208=CARTESIAN_POINT('Ctrl Pts',(18.4822053765618,-44.7421501763609,-1.79127796352151));
#8209=CARTESIAN_POINT('Ctrl Pts',(18.4836683130458,-44.7411871172364,-1.78913103491851));
#8210=CARTESIAN_POINT('Ctrl Pts',(18.4850117290154,-44.7403280695135,-1.78718848257471));
#8211=CARTESIAN_POINT('Ctrl Pts',(18.486229714533,-44.7395641131514,-1.78544433398189));
#8212=CARTESIAN_POINT('Ctrl Pts',(18.4873872880559,-44.7388380489704,-1.78378669503485));
#8213=CARTESIAN_POINT('Ctrl Pts',(18.4891933860945,-44.7377225025067,-1.78121987593171));
#8214=CARTESIAN_POINT('Ctrl Pts',(18.4912772121235,-44.736491572082,-1.77832245138861));
#8215=CARTESIAN_POINT('Ctrl Pts',(18.4932650638731,-44.7353173343269,-1.7755584728382));
#8216=CARTESIAN_POINT('Ctrl Pts',(18.4955070564238,-44.7340392999125,-1.77249400980688));
#8217=CARTESIAN_POINT('Ctrl Pts',(18.4976460311451,-44.73286651034,-1.7696234929949));
#8218=CARTESIAN_POINT('Ctrl Pts',(18.498580264236,-44.7323542748206,-1.76836974662419));
#8219=CARTESIAN_POINT('Ctrl Pts',(18.4994950361885,-44.7318614215613,-1.76715206750054));
#8220=CARTESIAN_POINT('Ctrl Pts',(18.5003576343236,-44.7314034029234,-1.76601151907465));
#8221=CARTESIAN_POINT('Ctrl Pts',(18.5052655100644,-44.7287974402272,-1.75952220531098));
#8222=CARTESIAN_POINT('Ctrl Pts',(18.5101114448029,-44.7264480717817,-1.75337123329988));
#8223=CARTESIAN_POINT('Ctrl Pts',(18.5148610415796,-44.7243168044746,-1.74753823326662));
#8224=CARTESIAN_POINT('Ctrl Pts',(18.5190637936833,-44.7224309205608,-1.74237681550574));
#8225=CARTESIAN_POINT('Ctrl Pts',(18.5231989650652,-44.7207126167444,-1.73745616497633));
#8226=CARTESIAN_POINT('Ctrl Pts',(18.5272331822637,-44.7191479490509,-1.73278354382904));
#8227=CARTESIAN_POINT('Ctrl Pts',(18.5323172306827,-44.7171761052155,-1.72689495851323));
#8228=CARTESIAN_POINT('Ctrl Pts',(18.5372581723168,-44.7154369208339,-1.72137500930987));
#8229=CARTESIAN_POINT('Ctrl Pts',(18.542026435158,-44.7138915816973,-1.71619922278658));
#8230=CARTESIAN_POINT('Ctrl Pts',(18.5452525177388,-44.7128460454431,-1.71269742028524));
#8231=CARTESIAN_POINT('Ctrl Pts',(18.5490365918176,-44.7116862681572,-1.70866569029123));
#8232=CARTESIAN_POINT('Ctrl Pts',(18.5531138200782,-44.7105402951052,-1.70443999061808));
#8233=CARTESIAN_POINT('Ctrl Pts',(18.5552257322364,-44.7099467069452,-1.70225117362124));
#8234=CARTESIAN_POINT('Ctrl Pts',(18.5574158606756,-44.7093563068657,-1.70001003806637));
#8235=CARTESIAN_POINT('Ctrl Pts',(18.5596440490768,-44.708782795066,-1.69776098915752));
#8236=CARTESIAN_POINT('Ctrl Pts',(18.5637477023021,-44.7077265587329,-1.69361891714801));
#8237=CARTESIAN_POINT('Ctrl Pts',(18.5679830742223,-44.706729306282,-1.68945007474751));
#8238=CARTESIAN_POINT('Ctrl Pts',(18.5720778157018,-44.7058476668227,-1.68551414114025));
#8239=CARTESIAN_POINT('Ctrl Pts',(18.5728458353102,-44.7056823043949,-1.68477590792015));
#8240=CARTESIAN_POINT('Ctrl Pts',(18.5736088231611,-44.7055209032599,-1.68404580744789));
#8241=CARTESIAN_POINT('Ctrl Pts',(18.5743648681294,-44.7053636940034,-1.68332547089644));
#8242=CARTESIAN_POINT('Ctrl Pts',(18.58122353312,-44.7039375280099,-1.67679074439966));
#8243=CARTESIAN_POINT('Ctrl Pts',(18.5880173171863,-44.7027501655137,-1.67057651486332));
#8244=CARTESIAN_POINT('Ctrl Pts',(18.5947210176705,-44.7017664392736,-1.66466019129503));
#8245=CARTESIAN_POINT('Ctrl Pts',(18.5989653103428,-44.7011436157925,-1.66091440807775));
#8246=CARTESIAN_POINT('Ctrl Pts',(18.6031738180247,-44.7006024502006,-1.65728783989602));
#8247=CARTESIAN_POINT('Ctrl Pts',(18.6073407582855,-44.700135176751,-1.65377565492483));
#8248=CARTESIAN_POINT('Ctrl Pts',(18.6125018364014,-44.6995564224076,-1.64942554192594));
#8249=CARTESIAN_POINT('Ctrl Pts',(18.6181386121197,-44.6990337803828,-1.64479966015728));
#8250=CARTESIAN_POINT('Ctrl Pts',(18.6240306101813,-44.6986245769102,-1.64012155899839));
#8251=CARTESIAN_POINT('Ctrl Pts',(18.6268033999718,-44.6984320046794,-1.63792003228428));
#8252=CARTESIAN_POINT('Ctrl Pts',(18.6296323111388,-44.6982640568705,-1.63570665739715));
#8253=CARTESIAN_POINT('Ctrl Pts',(18.6324920213832,-44.6981237807725,-1.63350305160767));
#8254=CARTESIAN_POINT('Ctrl Pts',(18.6362109497917,-44.6979413578269,-1.63063735841798));
#8255=CARTESIAN_POINT('Ctrl Pts',(18.6399646635497,-44.6978067642329,-1.62780173184111));
#8256=CARTESIAN_POINT('Ctrl Pts',(18.6436937629378,-44.697720531018,-1.62503928727001));
#8257=CARTESIAN_POINT('Ctrl Pts',(18.6519075484317,-44.6975305920927,-1.61895467412767));
#8258=CARTESIAN_POINT('Ctrl Pts',(18.6599702366363,-44.697569880747,-1.61324230583385));
#8259=CARTESIAN_POINT('Ctrl Pts',(18.6680416881922,-44.6978090218053,-1.60775448089976));
#8260=CARTESIAN_POINT('Ctrl Pts',(18.6694848509728,-44.6978517798486,-1.60677326647549));
#8261=CARTESIAN_POINT('Ctrl Pts',(18.6709283344754,-44.697901024391,-1.60579931342513));
#8262=CARTESIAN_POINT('Ctrl Pts',(18.6723731047756,-44.6979567121928,-1.60483188349929));
#8263=CARTESIAN_POINT('Ctrl Pts',(18.6805679321806,-44.6982725768841,-1.59934456051963));
#8264=CARTESIAN_POINT('Ctrl Pts',(18.6888021087005,-44.6987928324897,-1.59406520294023));
#8265=CARTESIAN_POINT('Ctrl Pts',(18.6972615123352,-44.6995351544724,-1.5888818875588));
#8266=CARTESIAN_POINT('Ctrl Pts',(18.7026429287197,-44.7000073796851,-1.58558454184454));
#8267=CARTESIAN_POINT('Ctrl Pts',(18.7081158005212,-44.7005701960318,-1.58232667770584));
#8268=CARTESIAN_POINT('Ctrl Pts',(18.7137314098992,-44.7012361070428,-1.57908626479971));
#8269=CARTESIAN_POINT('Ctrl Pts',(18.7159232409764,-44.7014960190755,-1.57782149774905));
#8270=CARTESIAN_POINT('Ctrl Pts',(18.7181370386302,-44.7017717646743,-1.57655937941308));
#8271=CARTESIAN_POINT('Ctrl Pts',(18.7203759135888,-44.7020643954889,-1.57529891730949));
#8272=CARTESIAN_POINT('Ctrl Pts',(18.7326429648932,-44.7036677531046,-1.56839270165288));
#8273=CARTESIAN_POINT('Ctrl Pts',(18.7447343611095,-44.7056570974029,-1.56206039186384));
#8274=CARTESIAN_POINT('Ctrl Pts',(18.7565711408401,-44.7079508087299,-1.55626683595386));
#8275=CARTESIAN_POINT('Ctrl Pts',(18.7579890031085,-44.7082255597026,-1.55557285798758));
#8276=CARTESIAN_POINT('Ctrl Pts',(18.7594040701221,-44.7085049379473,-1.55488629909964));
#8277=CARTESIAN_POINT('Ctrl Pts',(18.7608158989421,-44.7087887219445,-1.55420722350708));
#8278=CARTESIAN_POINT('Ctrl Pts',(18.7674150186135,-44.7101151749334,-1.55103311271009));
#8279=CARTESIAN_POINT('Ctrl Pts',(18.7739379815234,-44.7115363266361,-1.54802478285648));
#8280=CARTESIAN_POINT('Ctrl Pts',(18.7803771570996,-44.713039660849,-1.54517187036228));
#8281=CARTESIAN_POINT('Ctrl Pts',(18.7819869509937,-44.7134154944022,-1.54445864223873));
#8282=CARTESIAN_POINT('Ctrl Pts',(18.7834188829847,-44.7137558360497,-1.54383126623162));
#8283=CARTESIAN_POINT('Ctrl Pts',(18.7847866301017,-44.7140849945395,-1.54323678801712));
#8284=CARTESIAN_POINT('Ctrl Pts',(18.7858124404394,-44.7143318634069,-1.54279092935624));
#8285=CARTESIAN_POINT('Ctrl Pts',(18.7868021784292,-44.7145725376574,-1.54236366527359));
#8286=CARTESIAN_POINT('Ctrl Pts',(18.7878041612743,-44.7148185849535,-1.54193392585844));
#8287=CARTESIAN_POINT('Ctrl Pts',(18.789307135542,-44.7151876558978,-1.54128931673572));
#8288=CARTESIAN_POINT('Ctrl Pts',(18.7908372641589,-44.7155695477042,-1.54063843407745));
#8289=CARTESIAN_POINT('Ctrl Pts',(18.7925588171132,-44.7160071547615,-1.53991486409862));
#8290=CARTESIAN_POINT('Ctrl Pts',(18.7934195935903,-44.7162259582902,-1.53955307910921));
#8291=CARTESIAN_POINT('Ctrl Pts',(18.7943283140833,-44.7164585734448,-1.53917329091374));
#8292=CARTESIAN_POINT('Ctrl Pts',(18.7953057447759,-44.7167106512364,-1.53876797724112));
#8293=CARTESIAN_POINT('Ctrl Pts',(18.7962831753214,-44.71696272899,-1.53836266362956));
#8294=CARTESIAN_POINT('Ctrl Pts',(18.7973293149979,-44.7172342636307,-1.53793181150032));
#8295=CARTESIAN_POINT('Ctrl Pts',(18.7984650862778,-44.7175312467786,-1.53746858862735));
#8296=CARTESIAN_POINT('Ctrl Pts',(3.62216201968442,-19.8058202438613,-1.94799199564959));
#8297=CARTESIAN_POINT('Ctrl Pts',(3.34425572651223,-20.2137053466864,-1.54490813204841));
#8298=CARTESIAN_POINT('Ctrl Pts',(3.25594179788809,-20.5121292468035,-0.988830267143717));
#8299=CARTESIAN_POINT('Ctrl Pts',(3.16762786926396,-20.8105531469205,-0.432752402239027));
#8300=CARTESIAN_POINT('Ctrl Pts',(3.3076189187292,-20.9771651064803,0.166181422977342));
#8301=CARTESIAN_POINT('Ctrl Pts',(3.44760996819445,-21.1437770660401,0.765115248193711));
#8302=CARTESIAN_POINT('Ctrl Pts',(3.80940000840298,-21.1823333185883,1.28827884419634));
#8303=CARTESIAN_POINT('Ctrl Pts',(4.17119004861151,-21.2208895711365,1.81144244019896));
#8304=CARTESIAN_POINT('Ctrl Pts',(4.70434308191443,-21.1605093534924,2.15521684061908));
#8305=CARTESIAN_POINT('Ctrl Pts',(5.23749611521735,-21.1001291358485,2.49899124103919));
#8306=CARTESIAN_POINT('Ctrl Pts',(5.8576356015542,-20.9895272661294,2.59528770975726));
#8307=CARTESIAN_POINT('Ctrl Pts',(6.47777508789106,-20.8789253964104,2.69158417847533));
#8308=CARTESIAN_POINT('Ctrl Pts',(7.08329575335921,-20.7767637068552,2.52133001886304));
#8309=CARTESIAN_POINT('Ctrl Pts',(7.68881641882736,-20.6746020173,2.35107585925076));
#8310=CARTESIAN_POINT('Ctrl Pts',(8.18100842628526,-20.6378706589539,1.94799199564959));
#8311=CARTESIAN_POINT('Ctrl Pts',(8.67320043374317,-20.6011393006078,1.54490813204841));
#8312=CARTESIAN_POINT('Ctrl Pts',(8.97580007665302,-20.6738691449698,0.988830267143717));
#8313=CARTESIAN_POINT('Ctrl Pts',(9.27839971956287,-20.7465989893318,0.432752402239027));
#8314=CARTESIAN_POINT('Ctrl Pts',(9.35269438438334,-20.9511407742511,-0.166181422977342));
#8315=CARTESIAN_POINT('Ctrl Pts',(9.4269890492038,-21.1556825591703,-0.765115248193711));
#8316=CARTESIAN_POINT('Ctrl Pts',(9.27948472328098,-21.4882800511012,-1.28827884419634));
#8317=CARTESIAN_POINT('Ctrl Pts',(9.13198039735816,-21.8208775430321,-1.81144244019896));
#8318=CARTESIAN_POINT('Ctrl Pts',(8.81311307834095,-22.2524115051551,-2.15521684061908));
#8319=CARTESIAN_POINT('Ctrl Pts',(8.49424575932375,-22.6839454672782,-2.49899124103919));
#8320=CARTESIAN_POINT('Ctrl Pts',(8.0883919872726,-23.1657010814762,-2.59528770975726));
#8321=CARTESIAN_POINT('Ctrl Pts',(7.68253821522146,-23.6474566956743,-2.69158417847533));
#8322=CARTESIAN_POINT('Ctrl Pts',(7.29130326403902,-24.1207721297085,-2.52133001886305));
#8323=CARTESIAN_POINT('Ctrl Pts',(6.90006831285659,-24.5940875637428,-2.35107585925076));
#8324=CARTESIAN_POINT('Ctrl Pts',(6.62216201968439,-25.0019726665679,-1.94799199564959));
#8325=CARTESIAN_POINT('Ctrl Pts',(6.34425572651219,-25.4098577693931,-1.54490813204841));
#8326=CARTESIAN_POINT('Ctrl Pts',(6.25594179788806,-25.7082816695101,-0.988830267143717));
#8327=CARTESIAN_POINT('Ctrl Pts',(6.16762786926392,-26.0067055696272,-0.432752402239027));
#8328=CARTESIAN_POINT('Ctrl Pts',(6.30761891872917,-26.1733175291869,0.166181422977342));
#8329=CARTESIAN_POINT('Ctrl Pts',(6.44760996819441,-26.3399294887468,0.765115248193711));
#8330=CARTESIAN_POINT('Ctrl Pts',(6.80940000840295,-26.3784857412949,1.28827884419634));
#8331=CARTESIAN_POINT('Ctrl Pts',(7.17119004861148,-26.4170419938431,1.81144244019896));
#8332=CARTESIAN_POINT('Ctrl Pts',(7.7043430819144,-26.3566617761991,2.15521684061908));
#8333=CARTESIAN_POINT('Ctrl Pts',(8.23749611521731,-26.2962815585551,2.49899124103919));
#8334=CARTESIAN_POINT('Ctrl Pts',(8.85763560155417,-26.1856796888361,2.59528770975726));
#8335=CARTESIAN_POINT('Ctrl Pts',(9.47777508789103,-26.0750778191171,2.69158417847533));
#8336=CARTESIAN_POINT('Ctrl Pts',(10.0832957533592,-25.9729161295619,2.52133001886304));
#8337=CARTESIAN_POINT('Ctrl Pts',(10.6888164188273,-25.8707544400067,2.35107585925076));
#8338=CARTESIAN_POINT('Ctrl Pts',(11.1810084262852,-25.8340230816606,1.94799199564959));
#8339=CARTESIAN_POINT('Ctrl Pts',(11.6732004337431,-25.7972917233145,1.54490813204841));
#8340=CARTESIAN_POINT('Ctrl Pts',(11.975800076653,-25.8700215676765,0.988830267143717));
#8341=CARTESIAN_POINT('Ctrl Pts',(12.2783997195628,-25.9427514120385,0.432752402239027));
#8342=CARTESIAN_POINT('Ctrl Pts',(12.3526943843833,-26.1472931969577,-0.166181422977342));
#8343=CARTESIAN_POINT('Ctrl Pts',(12.4269890492038,-26.351834981877,-0.765115248193711));
#8344=CARTESIAN_POINT('Ctrl Pts',(12.279484723281,-26.6844324738078,-1.28827884419634));
#8345=CARTESIAN_POINT('Ctrl Pts',(12.1319803973581,-27.0170299657387,-1.81144244019896));
#8346=CARTESIAN_POINT('Ctrl Pts',(11.8131130783409,-27.4485639278618,-2.15521684061908));
#8347=CARTESIAN_POINT('Ctrl Pts',(11.4942457593237,-27.8800978899848,-2.49899124103919));
#8348=CARTESIAN_POINT('Ctrl Pts',(11.0883919872726,-28.3618535041829,-2.59528770975726));
#8349=CARTESIAN_POINT('Ctrl Pts',(10.6825382152214,-28.8436091183809,-2.69158417847533));
#8350=CARTESIAN_POINT('Ctrl Pts',(10.291303264039,-29.3169245524152,-2.52133001886305));
#8351=CARTESIAN_POINT('Ctrl Pts',(9.90006831285655,-29.7902399864494,-2.35107585925076));
#8352=CARTESIAN_POINT('Ctrl Pts',(9.62216201968436,-30.1981250892746,-1.94799199564959));
#8353=CARTESIAN_POINT('Ctrl Pts',(9.34425572651217,-30.6060101920997,-1.54490813204841));
#8354=CARTESIAN_POINT('Ctrl Pts',(9.25594179788803,-30.9044340922168,-0.988830267143717));
#8355=CARTESIAN_POINT('Ctrl Pts',(9.16762786926389,-31.2028579923338,-0.432752402239027));
#8356=CARTESIAN_POINT('Ctrl Pts',(9.30761891872914,-31.3694699518936,0.166181422977342));
#8357=CARTESIAN_POINT('Ctrl Pts',(9.44760996819438,-31.5360819114534,0.765115248193711));
#8358=CARTESIAN_POINT('Ctrl Pts',(9.80940000840292,-31.5746381640016,1.28827884419634));
#8359=CARTESIAN_POINT('Ctrl Pts',(10.1711900486115,-31.6131944165497,1.81144244019896));
#8360=CARTESIAN_POINT('Ctrl Pts',(10.7043430819144,-31.5528141989058,2.15521684061908));
#8361=CARTESIAN_POINT('Ctrl Pts',(11.2374961152173,-31.4924339812617,2.49899124103919));
#8362=CARTESIAN_POINT('Ctrl Pts',(11.8576356015541,-31.3818321115427,2.59528770975726));
#8363=CARTESIAN_POINT('Ctrl Pts',(12.477775087891,-31.2712302418237,2.69158417847533));
#8364=CARTESIAN_POINT('Ctrl Pts',(13.0832957533591,-31.1690685522685,2.52133001886304));
#8365=CARTESIAN_POINT('Ctrl Pts',(13.6888164188273,-31.0669068627133,2.35107585925076));
#8366=CARTESIAN_POINT('Ctrl Pts',(14.1810084262852,-31.0301755043672,1.94799199564959));
#8367=CARTESIAN_POINT('Ctrl Pts',(14.6732004337431,-30.9934441460211,1.54490813204841));
#8368=CARTESIAN_POINT('Ctrl Pts',(14.975800076653,-31.0661739903831,0.988830267143717));
#8369=CARTESIAN_POINT('Ctrl Pts',(15.2783997195628,-31.1389038347451,0.432752402239027));
#8370=CARTESIAN_POINT('Ctrl Pts',(15.3526943843833,-31.3434456196644,-0.166181422977342));
#8371=CARTESIAN_POINT('Ctrl Pts',(15.4269890492037,-31.5479874045836,-0.765115248193711));
#8372=CARTESIAN_POINT('Ctrl Pts',(15.2794847232809,-31.8805848965145,-1.28827884419634));
#8373=CARTESIAN_POINT('Ctrl Pts',(15.1319803973581,-32.2131823884454,-1.81144244019896));
#8374=CARTESIAN_POINT('Ctrl Pts',(14.8131130783409,-32.6447163505684,-2.15521684061908));
#8375=CARTESIAN_POINT('Ctrl Pts',(14.4942457593237,-33.0762503126915,-2.49899124103919));
#8376=CARTESIAN_POINT('Ctrl Pts',(14.0883919872725,-33.5580059268895,-2.59528770975726));
#8377=CARTESIAN_POINT('Ctrl Pts',(13.6825382152214,-34.0397615410876,-2.69158417847533));
#8378=CARTESIAN_POINT('Ctrl Pts',(13.291303264039,-34.5130769751218,-2.52133001886305));
#8379=CARTESIAN_POINT('Ctrl Pts',(12.9000683128565,-34.9863924091561,-2.35107585925076));
#8380=CARTESIAN_POINT('Ctrl Pts',(12.6221620196843,-35.3942775119812,-1.94799199564959));
#8381=CARTESIAN_POINT('Ctrl Pts',(12.3442557265121,-35.8021626148064,-1.54490813204841));
#8382=CARTESIAN_POINT('Ctrl Pts',(12.255941797888,-36.1005865149234,-0.988830267143717));
#8383=CARTESIAN_POINT('Ctrl Pts',(12.1676278692639,-36.3990104150405,-0.432752402239027));
#8384=CARTESIAN_POINT('Ctrl Pts',(12.3076189187291,-36.5656223746002,0.166181422977342));
#8385=CARTESIAN_POINT('Ctrl Pts',(12.4476099681944,-36.73223433416,0.765115248193711));
#8386=CARTESIAN_POINT('Ctrl Pts',(12.8094000084029,-36.7707905867082,1.28827884419634));
#8387=CARTESIAN_POINT('Ctrl Pts',(13.1711900486114,-36.8093468392564,1.81144244019896));
#8388=CARTESIAN_POINT('Ctrl Pts',(13.7043430819143,-36.7489666216124,2.15521684061908));
#8389=CARTESIAN_POINT('Ctrl Pts',(14.2374961152173,-36.6885864039684,2.49899124103919));
#8390=CARTESIAN_POINT('Ctrl Pts',(14.8576356015541,-36.5779845342494,2.59528770975726));
#8391=CARTESIAN_POINT('Ctrl Pts',(15.477775087891,-36.4673826645304,2.69158417847533));
#8392=CARTESIAN_POINT('Ctrl Pts',(16.0832957533591,-36.3652209749752,2.52133001886304));
#8393=CARTESIAN_POINT('Ctrl Pts',(16.6888164188273,-36.26305928542,2.35107585925076));
#8394=CARTESIAN_POINT('Ctrl Pts',(17.1810084262852,-36.2263279270739,1.94799199564959));
#8395=CARTESIAN_POINT('Ctrl Pts',(17.6732004337431,-36.1895965687278,1.54490813204841));
#8396=CARTESIAN_POINT('Ctrl Pts',(17.9758000766529,-36.2623264130898,0.988830267143717));
#8397=CARTESIAN_POINT('Ctrl Pts',(18.2783997195628,-36.3350562574518,0.432752402239027));
#8398=CARTESIAN_POINT('Ctrl Pts',(18.3526943843832,-36.539598042371,-0.166181422977342));
#8399=CARTESIAN_POINT('Ctrl Pts',(18.4269890492037,-36.7441398272903,-0.765115248193711));
#8400=CARTESIAN_POINT('Ctrl Pts',(18.2794847232809,-37.0767373192211,-1.28827884419634));
#8401=CARTESIAN_POINT('Ctrl Pts',(18.1319803973581,-37.409334811152,-1.81144244019896));
#8402=CARTESIAN_POINT('Ctrl Pts',(17.8131130783409,-37.8408687732751,-2.15521684061908));
#8403=CARTESIAN_POINT('Ctrl Pts',(17.4942457593237,-38.2724027353981,-2.49899124103919));
#8404=CARTESIAN_POINT('Ctrl Pts',(17.0883919872725,-38.7541583495962,-2.59528770975726));
#8405=CARTESIAN_POINT('Ctrl Pts',(16.6825382152214,-39.2359139637942,-2.69158417847533));
#8406=CARTESIAN_POINT('Ctrl Pts',(16.2913032640389,-39.7092293978285,-2.52133001886305));
#8407=CARTESIAN_POINT('Ctrl Pts',(15.9000683128565,-40.1825448318627,-2.35107585925076));
#8408=CARTESIAN_POINT('Ctrl Pts',(15.6221620196843,-40.5904299346879,-1.94799199564959));
#8409=CARTESIAN_POINT('Ctrl Pts',(15.3442557265121,-40.998315037513,-1.54490813204841));
#8410=CARTESIAN_POINT('Ctrl Pts',(15.255941797888,-41.2967389376301,-0.988830267143717));
#8411=CARTESIAN_POINT('Ctrl Pts',(15.1676278692638,-41.5951628377471,-0.432752402239027));
#8412=CARTESIAN_POINT('Ctrl Pts',(15.3076189187291,-41.7617747973069,0.166181422977342));
#8413=CARTESIAN_POINT('Ctrl Pts',(15.4476099681943,-41.9283867568667,0.765115248193711));
#8414=CARTESIAN_POINT('Ctrl Pts',(15.8094000084029,-41.9669430094149,1.28827884419634));
#8415=CARTESIAN_POINT('Ctrl Pts',(16.1711900486114,-42.0054992619631,1.81144244019896));
#8416=CARTESIAN_POINT('Ctrl Pts',(16.7043430819143,-41.945119044319,2.15521684061908));
#8417=CARTESIAN_POINT('Ctrl Pts',(17.2374961152172,-41.884738826675,2.49899124103919));
#8418=CARTESIAN_POINT('Ctrl Pts',(17.8576356015541,-41.774136956956,2.59528770975726));
#8419=CARTESIAN_POINT('Ctrl Pts',(18.4777750878909,-41.6635350872371,2.69158417847533));
#8420=CARTESIAN_POINT('Ctrl Pts',(19.0832957533591,-41.5613733976818,2.52133001886304));
#8421=CARTESIAN_POINT('Ctrl Pts',(19.6888164188272,-41.4592117081266,2.35107585925076));
#8422=CARTESIAN_POINT('Ctrl Pts',(20.1810084262851,-41.4224803497805,1.94799199564959));
#8423=CARTESIAN_POINT('Ctrl Pts',(20.673200433743,-41.3857489914344,1.54490813204841));
#8424=CARTESIAN_POINT('Ctrl Pts',(20.9758000766529,-41.4584788357964,0.988830267143717));
#8425=CARTESIAN_POINT('Ctrl Pts',(21.2783997195627,-41.5312086801584,0.432752402239027));
#8426=CARTESIAN_POINT('Ctrl Pts',(21.3526943843832,-41.7357504650777,-0.166181422977342));
#8427=CARTESIAN_POINT('Ctrl Pts',(21.4269890492037,-41.940292249997,-0.765115248193711));
#8428=CARTESIAN_POINT('Ctrl Pts',(21.2794847232809,-42.2728897419278,-1.28827884419634));
#8429=CARTESIAN_POINT('Ctrl Pts',(21.131980397358,-42.6054872338587,-1.81144244019896));
#8430=CARTESIAN_POINT('Ctrl Pts',(20.8131130783408,-43.0370211959817,-2.15521684061908));
#8431=CARTESIAN_POINT('Ctrl Pts',(20.4942457593236,-43.4685551581048,-2.49899124103919));
#8432=CARTESIAN_POINT('Ctrl Pts',(20.0883919872725,-43.9503107723028,-2.59528770975726));
#8433=CARTESIAN_POINT('Ctrl Pts',(19.6825382152213,-44.4320663865008,-2.69158417847533));
#8434=CARTESIAN_POINT('Ctrl Pts',(19.2913032640389,-44.9053818205351,-2.52133001886305));
#8435=CARTESIAN_POINT('Ctrl Pts',(18.9000683128565,-45.3786972545694,-2.35107585925076));
#8436=CARTESIAN_POINT('Ctrl Pts',(18.6221620196843,-45.7865823573945,-1.94799199564959));
#8437=CARTESIAN_POINT('Ctrl Pts',(4.55184415422078,-20.0688325405066,-1.69008569379309));
#8438=CARTESIAN_POINT('Ctrl Pts',(4.32491681918215,-20.4472849281303,-1.4407517010054));
#8439=CARTESIAN_POINT('Ctrl Pts',(4.22476116346577,-20.7525456525717,-1.04873843619563));
#8440=CARTESIAN_POINT('Ctrl Pts',(4.12460550774938,-21.0578063770131,-0.656725171385866));
#8441=CARTESIAN_POINT('Ctrl Pts',(4.19227954417643,-21.2661705835175,-0.199675669376779));
#8442=CARTESIAN_POINT('Ctrl Pts',(4.25995358060348,-21.4745347900219,0.257373832632308));
#8443=CARTESIAN_POINT('Ctrl Pts',(4.50327459317005,-21.5814891675698,0.688935312623524));
#8444=CARTESIAN_POINT('Ctrl Pts',(4.74659560573663,-21.6884435451177,1.12049679261474));
#8445=CARTESIAN_POINT('Ctrl Pts',(5.13859184064558,-21.7095602430244,1.44109420672161));
#8446=CARTESIAN_POINT('Ctrl Pts',(5.53058807555453,-21.7306769409311,1.76169162082848));
#8447=CARTESIAN_POINT('Ctrl Pts',(6.01484082784187,-21.6985293136949,1.90782671931788));
#8448=CARTESIAN_POINT('Ctrl Pts',(6.49909358012921,-21.6663816864587,2.05396181780729));
#8449=CARTESIAN_POINT('Ctrl Pts',(7.00091161011221,-21.6240927414165,1.99669075219403));
#8450=CARTESIAN_POINT('Ctrl Pts',(7.50272964009522,-21.5818037963743,1.93941968658077));
#8451=CARTESIAN_POINT('Ctrl Pts',(7.94394268941957,-21.5745051532296,1.69008569379309));
#8452=CARTESIAN_POINT('Ctrl Pts',(8.38515573874391,-21.5672065100849,1.4407517010054));
#8453=CARTESIAN_POINT('Ctrl Pts',(8.699597108746,-21.6330995301225,1.04873843619563));
#8454=CARTESIAN_POINT('Ctrl Pts',(9.0140384787481,-21.6989925501602,0.656725171385866));
#8455=CARTESIAN_POINT('Ctrl Pts',(9.16065015660677,-21.8617820881348,0.199675669376779));
#8456=CARTESIAN_POINT('Ctrl Pts',(9.30726183446543,-22.0245716261095,-0.257373832632308));
#8457=CARTESIAN_POINT('Ctrl Pts',(9.27822653618457,-22.2887709930406,-0.688935312623524));
#8458=CARTESIAN_POINT('Ctrl Pts',(9.24919123790371,-22.5529703599718,-1.12049679261474));
#8459=CARTESIAN_POINT('Ctrl Pts',(9.07148071728047,-22.9030074065441,-1.44109420672161));
#8460=CARTESIAN_POINT('Ctrl Pts',(8.89377019665723,-23.2530444531165,-1.76169162082848));
#8461=CARTESIAN_POINT('Ctrl Pts',(8.6238031586556,-23.6563458248317,-1.90782671931788));
#8462=CARTESIAN_POINT('Ctrl Pts',(8.35383612065398,-24.059647196547,-2.05396181780729));
#8463=CARTESIAN_POINT('Ctrl Pts',(8.06630380495668,-24.4730898860682,-1.99669075219403));
#8464=CARTESIAN_POINT('Ctrl Pts',(7.77877148925938,-24.8865325755895,-1.93941968658077));
#8465=CARTESIAN_POINT('Ctrl Pts',(7.55184415422075,-25.2649849632132,-1.69008569379309));
#8466=CARTESIAN_POINT('Ctrl Pts',(7.32491681918212,-25.6434373508369,-1.4407517010054));
#8467=CARTESIAN_POINT('Ctrl Pts',(7.22476116346574,-25.9486980752784,-1.04873843619563));
#8468=CARTESIAN_POINT('Ctrl Pts',(7.12460550774935,-26.2539587997198,-0.656725171385866));
#8469=CARTESIAN_POINT('Ctrl Pts',(7.1922795441764,-26.4623230062242,-0.199675669376779));
#8470=CARTESIAN_POINT('Ctrl Pts',(7.25995358060345,-26.6706872127285,0.257373832632308));
#8471=CARTESIAN_POINT('Ctrl Pts',(7.50327459317002,-26.7776415902764,0.688935312623524));
#8472=CARTESIAN_POINT('Ctrl Pts',(7.7465956057366,-26.8845959678243,1.12049679261474));
#8473=CARTESIAN_POINT('Ctrl Pts',(8.13859184064555,-26.905712665731,1.44109420672161));
#8474=CARTESIAN_POINT('Ctrl Pts',(8.5305880755545,-26.9268293636377,1.76169162082848));
#8475=CARTESIAN_POINT('Ctrl Pts',(9.01484082784184,-26.8946817364015,1.90782671931788));
#8476=CARTESIAN_POINT('Ctrl Pts',(9.49909358012917,-26.8625341091653,2.05396181780729));
#8477=CARTESIAN_POINT('Ctrl Pts',(10.0009116101122,-26.8202451641231,1.99669075219403));
#8478=CARTESIAN_POINT('Ctrl Pts',(10.5027296400952,-26.7779562190809,1.93941968658077));
#8479=CARTESIAN_POINT('Ctrl Pts',(10.9439426894195,-26.7706575759362,1.69008569379309));
#8480=CARTESIAN_POINT('Ctrl Pts',(11.3851557387439,-26.7633589327915,1.4407517010054));
#8481=CARTESIAN_POINT('Ctrl Pts',(11.699597108746,-26.8292519528292,1.04873843619563));
#8482=CARTESIAN_POINT('Ctrl Pts',(12.0140384787481,-26.8951449728668,0.656725171385866));
#8483=CARTESIAN_POINT('Ctrl Pts',(12.1606501566067,-27.0579345108415,0.199675669376779));
#8484=CARTESIAN_POINT('Ctrl Pts',(12.3072618344654,-27.2207240488161,-0.257373832632308));
#8485=CARTESIAN_POINT('Ctrl Pts',(12.2782265361845,-27.4849234157473,-0.688935312623524));
#8486=CARTESIAN_POINT('Ctrl Pts',(12.2491912379037,-27.7491227826784,-1.12049679261474));
#8487=CARTESIAN_POINT('Ctrl Pts',(12.0714807172804,-28.0991598292508,-1.44109420672161));
#8488=CARTESIAN_POINT('Ctrl Pts',(11.8937701966572,-28.4491968758231,-1.76169162082848));
#8489=CARTESIAN_POINT('Ctrl Pts',(11.6238031586556,-28.8524982475384,-1.90782671931788));
#8490=CARTESIAN_POINT('Ctrl Pts',(11.3538361206539,-29.2557996192536,-2.05396181780729));
#8491=CARTESIAN_POINT('Ctrl Pts',(11.0663038049567,-29.6692423087749,-1.99669075219403));
#8492=CARTESIAN_POINT('Ctrl Pts',(10.7787714892594,-30.0826849982961,-1.93941968658077));
#8493=CARTESIAN_POINT('Ctrl Pts',(10.5518441542207,-30.4611373859199,-1.69008569379309));
#8494=CARTESIAN_POINT('Ctrl Pts',(10.3249168191821,-30.8395897735436,-1.4407517010054));
#8495=CARTESIAN_POINT('Ctrl Pts',(10.2247611634657,-31.144850497985,-1.04873843619563));
#8496=CARTESIAN_POINT('Ctrl Pts',(10.1246055077493,-31.4501112224264,-0.656725171385866));
#8497=CARTESIAN_POINT('Ctrl Pts',(10.1922795441764,-31.6584754289308,-0.199675669376779));
#8498=CARTESIAN_POINT('Ctrl Pts',(10.2599535806034,-31.8668396354352,0.257373832632308));
#8499=CARTESIAN_POINT('Ctrl Pts',(10.50327459317,-31.9737940129831,0.688935312623524));
#8500=CARTESIAN_POINT('Ctrl Pts',(10.7465956057366,-32.080748390531,1.12049679261474));
#8501=CARTESIAN_POINT('Ctrl Pts',(11.1385918406455,-32.1018650884377,1.44109420672161));
#8502=CARTESIAN_POINT('Ctrl Pts',(11.5305880755545,-32.1229817863444,1.76169162082848));
#8503=CARTESIAN_POINT('Ctrl Pts',(12.0148408278418,-32.0908341591082,1.90782671931788));
#8504=CARTESIAN_POINT('Ctrl Pts',(12.4990935801291,-32.0586865318719,2.05396181780729));
#8505=CARTESIAN_POINT('Ctrl Pts',(13.0009116101121,-32.0163975868298,1.99669075219403));
#8506=CARTESIAN_POINT('Ctrl Pts',(13.5027296400952,-31.9741086417876,1.93941968658077));
#8507=CARTESIAN_POINT('Ctrl Pts',(13.9439426894195,-31.9668099986429,1.69008569379309));
#8508=CARTESIAN_POINT('Ctrl Pts',(14.3851557387438,-31.9595113554982,1.4407517010054));
#8509=CARTESIAN_POINT('Ctrl Pts',(14.6995971087459,-32.0254043755358,1.04873843619563));
#8510=CARTESIAN_POINT('Ctrl Pts',(15.014038478748,-32.0912973955735,0.656725171385866));
#8511=CARTESIAN_POINT('Ctrl Pts',(15.1606501566067,-32.2540869335481,0.199675669376779));
#8512=CARTESIAN_POINT('Ctrl Pts',(15.3072618344654,-32.4168764715228,-0.257373832632308));
#8513=CARTESIAN_POINT('Ctrl Pts',(15.2782265361845,-32.6810758384539,-0.688935312623524));
#8514=CARTESIAN_POINT('Ctrl Pts',(15.2491912379036,-32.9452752053851,-1.12049679261474));
#8515=CARTESIAN_POINT('Ctrl Pts',(15.0714807172804,-33.2953122519574,-1.44109420672161));
#8516=CARTESIAN_POINT('Ctrl Pts',(14.8937701966572,-33.6453492985298,-1.76169162082848));
#8517=CARTESIAN_POINT('Ctrl Pts',(14.6238031586555,-34.048650670245,-1.90782671931788));
#8518=CARTESIAN_POINT('Ctrl Pts',(14.3538361206539,-34.4519520419603,-2.05396181780729));
#8519=CARTESIAN_POINT('Ctrl Pts',(14.0663038049566,-34.8653947314815,-1.99669075219403));
#8520=CARTESIAN_POINT('Ctrl Pts',(13.7787714892593,-35.2788374210028,-1.93941968658077));
#8521=CARTESIAN_POINT('Ctrl Pts',(13.5518441542207,-35.6572898086265,-1.69008569379309));
#8522=CARTESIAN_POINT('Ctrl Pts',(13.3249168191821,-36.0357421962502,-1.4407517010054));
#8523=CARTESIAN_POINT('Ctrl Pts',(13.2247611634657,-36.3410029206916,-1.04873843619563));
#8524=CARTESIAN_POINT('Ctrl Pts',(13.1246055077493,-36.6462636451331,-0.656725171385866));
#8525=CARTESIAN_POINT('Ctrl Pts',(13.1922795441763,-36.8546278516375,-0.199675669376779));
#8526=CARTESIAN_POINT('Ctrl Pts',(13.2599535806034,-37.0629920581418,0.257373832632308));
#8527=CARTESIAN_POINT('Ctrl Pts',(13.50327459317,-37.1699464356897,0.688935312623524));
#8528=CARTESIAN_POINT('Ctrl Pts',(13.7465956057365,-37.2769008132376,1.12049679261474));
#8529=CARTESIAN_POINT('Ctrl Pts',(14.1385918406455,-37.2980175111443,1.44109420672161));
#8530=CARTESIAN_POINT('Ctrl Pts',(14.5305880755544,-37.319134209051,1.76169162082848));
#8531=CARTESIAN_POINT('Ctrl Pts',(15.0148408278418,-37.2869865818148,1.90782671931788));
#8532=CARTESIAN_POINT('Ctrl Pts',(15.4990935801291,-37.2548389545786,2.05396181780729));
#8533=CARTESIAN_POINT('Ctrl Pts',(16.0009116101121,-37.2125500095364,1.99669075219403));
#8534=CARTESIAN_POINT('Ctrl Pts',(16.5027296400951,-37.1702610644942,1.93941968658077));
#8535=CARTESIAN_POINT('Ctrl Pts',(16.9439426894195,-37.1629624213495,1.69008569379309));
#8536=CARTESIAN_POINT('Ctrl Pts',(17.3851557387438,-37.1556637782049,1.4407517010054));
#8537=CARTESIAN_POINT('Ctrl Pts',(17.6995971087459,-37.2215567982425,1.04873843619563));
#8538=CARTESIAN_POINT('Ctrl Pts',(18.014038478748,-37.2874498182801,0.656725171385866));
#8539=CARTESIAN_POINT('Ctrl Pts',(18.1606501566067,-37.4502393562548,0.199675669376779));
#8540=CARTESIAN_POINT('Ctrl Pts',(18.3072618344653,-37.6130288942294,-0.257373832632308));
#8541=CARTESIAN_POINT('Ctrl Pts',(18.2782265361845,-37.8772282611606,-0.688935312623524));
#8542=CARTESIAN_POINT('Ctrl Pts',(18.2491912379036,-38.1414276280917,-1.12049679261474));
#8543=CARTESIAN_POINT('Ctrl Pts',(18.0714807172804,-38.4914646746641,-1.44109420672161));
#8544=CARTESIAN_POINT('Ctrl Pts',(17.8937701966571,-38.8415017212364,-1.76169162082848));
#8545=CARTESIAN_POINT('Ctrl Pts',(17.6238031586555,-39.2448030929517,-1.90782671931788));
#8546=CARTESIAN_POINT('Ctrl Pts',(17.3538361206539,-39.6481044646669,-2.05396181780729));
#8547=CARTESIAN_POINT('Ctrl Pts',(17.0663038049566,-40.0615471541882,-1.99669075219403));
#8548=CARTESIAN_POINT('Ctrl Pts',(16.7787714892593,-40.4749898437094,-1.93941968658077));
#8549=CARTESIAN_POINT('Ctrl Pts',(16.5518441542207,-40.8534422313332,-1.69008569379309));
#8550=CARTESIAN_POINT('Ctrl Pts',(16.324916819182,-41.2318946189569,-1.4407517010054));
#8551=CARTESIAN_POINT('Ctrl Pts',(16.2247611634656,-41.5371553433983,-1.04873843619563));
#8552=CARTESIAN_POINT('Ctrl Pts',(16.1246055077493,-41.8424160678397,-0.656725171385866));
#8553=CARTESIAN_POINT('Ctrl Pts',(16.1922795441763,-42.0507802743441,-0.199675669376779));
#8554=CARTESIAN_POINT('Ctrl Pts',(16.2599535806034,-42.2591444808485,0.257373832632308));
#8555=CARTESIAN_POINT('Ctrl Pts',(16.5032745931699,-42.3660988583964,0.688935312623524));
#8556=CARTESIAN_POINT('Ctrl Pts',(16.7465956057365,-42.4730532359443,1.12049679261474));
#8557=CARTESIAN_POINT('Ctrl Pts',(17.1385918406455,-42.494169933851,1.44109420672161));
#8558=CARTESIAN_POINT('Ctrl Pts',(17.5305880755544,-42.5152866317577,1.76169162082848));
#8559=CARTESIAN_POINT('Ctrl Pts',(18.0148408278417,-42.4831390045215,1.90782671931788));
#8560=CARTESIAN_POINT('Ctrl Pts',(18.4990935801291,-42.4509913772853,2.05396181780729));
#8561=CARTESIAN_POINT('Ctrl Pts',(19.0009116101121,-42.4087024322431,1.99669075219403));
#8562=CARTESIAN_POINT('Ctrl Pts',(19.5027296400951,-42.3664134872009,1.93941968658077));
#8563=CARTESIAN_POINT('Ctrl Pts',(19.9439426894194,-42.3591148440562,1.69008569379309));
#8564=CARTESIAN_POINT('Ctrl Pts',(20.3851557387438,-42.3518162009115,1.4407517010054));
#8565=CARTESIAN_POINT('Ctrl Pts',(20.6995971087459,-42.4177092209491,1.04873843619563));
#8566=CARTESIAN_POINT('Ctrl Pts',(21.014038478748,-42.4836022409868,0.656725171385866));
#8567=CARTESIAN_POINT('Ctrl Pts',(21.1606501566066,-42.6463917789614,0.199675669376779));
#8568=CARTESIAN_POINT('Ctrl Pts',(21.3072618344653,-42.8091813169361,-0.257373832632308));
#8569=CARTESIAN_POINT('Ctrl Pts',(21.2782265361844,-43.0733806838672,-0.688935312623524));
#8570=CARTESIAN_POINT('Ctrl Pts',(21.2491912379036,-43.3375800507984,-1.12049679261474));
#8571=CARTESIAN_POINT('Ctrl Pts',(21.0714807172803,-43.6876170973707,-1.44109420672161));
#8572=CARTESIAN_POINT('Ctrl Pts',(20.8937701966571,-44.0376541439431,-1.76169162082848));
#8573=CARTESIAN_POINT('Ctrl Pts',(20.6238031586555,-44.4409555156583,-1.90782671931788));
#8574=CARTESIAN_POINT('Ctrl Pts',(20.3538361206538,-44.8442568873736,-2.05396181780729));
#8575=CARTESIAN_POINT('Ctrl Pts',(20.0663038049566,-45.2576995768948,-1.99669075219403));
#8576=CARTESIAN_POINT('Ctrl Pts',(19.7787714892593,-45.6711422664161,-1.93941968658077));
#8577=CARTESIAN_POINT('Ctrl Pts',(19.5518441542206,-46.0495946540398,-1.69008569379309));
#8578=CARTESIAN_POINT('Ctrl Pts',(4.55184415422078,-19.3686903861425,-0.976082217833403));
#8579=CARTESIAN_POINT('Ctrl Pts',(4.4660500642644,-19.6656594567264,-0.80664966398524));
#8580=CARTESIAN_POINT('Ctrl Pts',(4.46302775611024,-19.9148402168055,-0.557333680706485));
#8581=CARTESIAN_POINT('Ctrl Pts',(4.46000544795609,-20.1640209768846,-0.30801769742773));
#8582=CARTESIAN_POINT('Ctrl Pts',(4.56157448367832,-20.3528158964217,-0.0281983728666175));
#8583=CARTESIAN_POINT('Ctrl Pts',(4.66314351940055,-20.5416108159588,0.251620951694495));
#8584=CARTESIAN_POINT('Ctrl Pts',(4.87040786268996,-20.66938252122,0.506521968549832));
#8585=CARTESIAN_POINT('Ctrl Pts',(5.07767220597936,-20.7971542264811,0.761422985405168));
#8586=CARTESIAN_POINT('Ctrl Pts',(5.37080156859517,-20.8753517397202,0.940919422010711));
#8587=CARTESIAN_POINT('Ctrl Pts',(5.66393093121099,-20.9535492529593,1.12041585861625));
#8588=CARTESIAN_POINT('Ctrl Pts',(6.00608840476948,-21.0034403731477,1.18895624432295));
#8589=CARTESIAN_POINT('Ctrl Pts',(6.34824587832798,-21.0533314933362,1.25749663002964));
#8590=CARTESIAN_POINT('Ctrl Pts',(6.69288393578292,-21.1017904477443,1.2015057008556));
#8591=CARTESIAN_POINT('Ctrl Pts',(7.03752199323787,-21.1502494021524,1.14551477168157));
#8592=CARTESIAN_POINT('Ctrl Pts',(7.33760179747996,-21.2244340760476,0.976082217833403));
#8593=CARTESIAN_POINT('Ctrl Pts',(7.63768160172206,-21.2986187499427,0.80664966398524));
#8594=CARTESIAN_POINT('Ctrl Pts',(7.85498962416192,-21.4205917343427,0.557333680706485));
#8595=CARTESIAN_POINT('Ctrl Pts',(8.07229764660179,-21.5425647187427,0.308017697427731));
#8596=CARTESIAN_POINT('Ctrl Pts',(8.18501432516527,-21.7249235436846,0.0281983728666177));
#8597=CARTESIAN_POINT('Ctrl Pts',(8.29773100372875,-21.9072823686265,-0.251620951694495));
#8598=CARTESIAN_POINT('Ctrl Pts',(8.30475237472506,-22.1506644078444,-0.506521968549832));
#8599=CARTESIAN_POINT('Ctrl Pts',(8.31177374572137,-22.3940464470623,-0.761422985405168));
#8600=CARTESIAN_POINT('Ctrl Pts',(8.23293009739127,-22.6870026783022,-0.940919422010711));
#8601=CARTESIAN_POINT('Ctrl Pts',(8.15408644906117,-22.9799589095422,-1.12041585861625));
#8602=CARTESIAN_POINT('Ctrl Pts',(8.02621468978838,-23.3012215338328,-1.18895624432295));
#8603=CARTESIAN_POINT('Ctrl Pts',(7.8983429305156,-23.6224841581234,-1.25749663002964));
#8604=CARTESIAN_POINT('Ctrl Pts',(7.76799058734637,-23.9451789481943,-1.2015057008556));
#8605=CARTESIAN_POINT('Ctrl Pts',(7.63763824417713,-24.2678737382653,-1.14551477168157));
#8606=CARTESIAN_POINT('Ctrl Pts',(7.55184415422075,-24.5648428088492,-0.976082217833403));
#8607=CARTESIAN_POINT('Ctrl Pts',(7.46605006426437,-24.8618118794331,-0.80664966398524));
#8608=CARTESIAN_POINT('Ctrl Pts',(7.46302775611021,-25.1109926395121,-0.557333680706485));
#8609=CARTESIAN_POINT('Ctrl Pts',(7.46000544795606,-25.3601733995912,-0.30801769742773));
#8610=CARTESIAN_POINT('Ctrl Pts',(7.56157448367829,-25.5489683191283,-0.0281983728666175));
#8611=CARTESIAN_POINT('Ctrl Pts',(7.66314351940052,-25.7377632386655,0.251620951694495));
#8612=CARTESIAN_POINT('Ctrl Pts',(7.87040786268992,-25.8655349439266,0.506521968549832));
#8613=CARTESIAN_POINT('Ctrl Pts',(8.07767220597933,-25.9933066491878,0.761422985405168));
#8614=CARTESIAN_POINT('Ctrl Pts',(8.37080156859514,-26.0715041624269,0.940919422010711));
#8615=CARTESIAN_POINT('Ctrl Pts',(8.66393093121095,-26.1497016756659,1.12041585861625));
#8616=CARTESIAN_POINT('Ctrl Pts',(9.00608840476945,-26.1995927958544,1.18895624432295));
#8617=CARTESIAN_POINT('Ctrl Pts',(9.34824587832795,-26.2494839160429,1.25749663002964));
#8618=CARTESIAN_POINT('Ctrl Pts',(9.69288393578289,-26.297942870451,1.2015057008556));
#8619=CARTESIAN_POINT('Ctrl Pts',(10.0375219932378,-26.346401824859,1.14551477168157));
#8620=CARTESIAN_POINT('Ctrl Pts',(10.3376017974799,-26.4205864987542,0.976082217833403));
#8621=CARTESIAN_POINT('Ctrl Pts',(10.637681601722,-26.4947711726494,0.80664966398524));
#8622=CARTESIAN_POINT('Ctrl Pts',(10.8549896241619,-26.6167441570493,0.557333680706485));
#8623=CARTESIAN_POINT('Ctrl Pts',(11.0722976466018,-26.7387171414493,0.308017697427731));
#8624=CARTESIAN_POINT('Ctrl Pts',(11.1850143251652,-26.9210759663912,0.0281983728666177));
#8625=CARTESIAN_POINT('Ctrl Pts',(11.2977310037287,-27.1034347913331,-0.251620951694495));
#8626=CARTESIAN_POINT('Ctrl Pts',(11.304752374725,-27.346816830551,-0.506521968549832));
#8627=CARTESIAN_POINT('Ctrl Pts',(11.3117737457213,-27.5901988697689,-0.761422985405168));
#8628=CARTESIAN_POINT('Ctrl Pts',(11.2329300973912,-27.8831551010089,-0.940919422010711));
#8629=CARTESIAN_POINT('Ctrl Pts',(11.1540864490611,-28.1761113322489,-1.12041585861625));
#8630=CARTESIAN_POINT('Ctrl Pts',(11.0262146897884,-28.4973739565395,-1.18895624432295));
#8631=CARTESIAN_POINT('Ctrl Pts',(10.8983429305156,-28.8186365808301,-1.25749663002964));
#8632=CARTESIAN_POINT('Ctrl Pts',(10.7679905873463,-29.141331370901,-1.2015057008556));
#8633=CARTESIAN_POINT('Ctrl Pts',(10.6376382441771,-29.4640261609719,-1.14551477168157));
#8634=CARTESIAN_POINT('Ctrl Pts',(10.5518441542207,-29.7609952315558,-0.976082217833403));
#8635=CARTESIAN_POINT('Ctrl Pts',(10.4660500642643,-30.0579643021397,-0.80664966398524));
#8636=CARTESIAN_POINT('Ctrl Pts',(10.4630277561102,-30.3071450622188,-0.557333680706485));
#8637=CARTESIAN_POINT('Ctrl Pts',(10.460005447956,-30.5563258222979,-0.30801769742773));
#8638=CARTESIAN_POINT('Ctrl Pts',(10.5615744836783,-30.745120741835,-0.0281983728666175));
#8639=CARTESIAN_POINT('Ctrl Pts',(10.6631435194005,-30.9339156613721,0.251620951694495));
#8640=CARTESIAN_POINT('Ctrl Pts',(10.8704078626899,-31.0616873666333,0.506521968549832));
#8641=CARTESIAN_POINT('Ctrl Pts',(11.0776722059793,-31.1894590718944,0.761422985405168));
#8642=CARTESIAN_POINT('Ctrl Pts',(11.3708015685951,-31.2676565851335,0.940919422010711));
#8643=CARTESIAN_POINT('Ctrl Pts',(11.6639309312109,-31.3458540983726,1.12041585861625));
#8644=CARTESIAN_POINT('Ctrl Pts',(12.0060884047694,-31.395745218561,1.18895624432295));
#8645=CARTESIAN_POINT('Ctrl Pts',(12.3482458783279,-31.4456363387495,1.25749663002964));
#8646=CARTESIAN_POINT('Ctrl Pts',(12.6928839357829,-31.4940952931576,1.2015057008556));
#8647=CARTESIAN_POINT('Ctrl Pts',(13.0375219932378,-31.5425542475657,1.14551477168157));
#8648=CARTESIAN_POINT('Ctrl Pts',(13.3376017974799,-31.6167389214609,0.976082217833403));
#8649=CARTESIAN_POINT('Ctrl Pts',(13.637681601722,-31.690923595356,0.80664966398524));
#8650=CARTESIAN_POINT('Ctrl Pts',(13.8549896241619,-31.812896579756,0.557333680706485));
#8651=CARTESIAN_POINT('Ctrl Pts',(14.0722976466017,-31.934869564156,0.308017697427731));
#8652=CARTESIAN_POINT('Ctrl Pts',(14.1850143251652,-32.1172283890979,0.0281983728666177));
#8653=CARTESIAN_POINT('Ctrl Pts',(14.2977310037287,-32.2995872140398,-0.251620951694495));
#8654=CARTESIAN_POINT('Ctrl Pts',(14.304752374725,-32.5429692532577,-0.506521968549832));
#8655=CARTESIAN_POINT('Ctrl Pts',(14.3117737457213,-32.7863512924756,-0.761422985405168));
#8656=CARTESIAN_POINT('Ctrl Pts',(14.2329300973912,-33.0793075237155,-0.940919422010711));
#8657=CARTESIAN_POINT('Ctrl Pts',(14.1540864490611,-33.3722637549555,-1.12041585861625));
#8658=CARTESIAN_POINT('Ctrl Pts',(14.0262146897883,-33.6935263792461,-1.18895624432295));
#8659=CARTESIAN_POINT('Ctrl Pts',(13.8983429305155,-34.0147890035367,-1.25749663002964));
#8660=CARTESIAN_POINT('Ctrl Pts',(13.7679905873463,-34.3374837936076,-1.2015057008556));
#8661=CARTESIAN_POINT('Ctrl Pts',(13.6376382441771,-34.6601785836786,-1.14551477168157));
#8662=CARTESIAN_POINT('Ctrl Pts',(13.5518441542207,-34.9571476542625,-0.976082217833403));
#8663=CARTESIAN_POINT('Ctrl Pts',(13.4660500642643,-35.2541167248464,-0.80664966398524));
#8664=CARTESIAN_POINT('Ctrl Pts',(13.4630277561101,-35.5032974849254,-0.557333680706485));
#8665=CARTESIAN_POINT('Ctrl Pts',(13.460005447956,-35.7524782450045,-0.30801769742773));
#8666=CARTESIAN_POINT('Ctrl Pts',(13.5615744836782,-35.9412731645416,-0.0281983728666175));
#8667=CARTESIAN_POINT('Ctrl Pts',(13.6631435194005,-36.1300680840788,0.251620951694495));
#8668=CARTESIAN_POINT('Ctrl Pts',(13.8704078626899,-36.2578397893399,0.506521968549832));
#8669=CARTESIAN_POINT('Ctrl Pts',(14.0776722059793,-36.3856114946011,0.761422985405168));
#8670=CARTESIAN_POINT('Ctrl Pts',(14.3708015685951,-36.4638090078402,0.940919422010711));
#8671=CARTESIAN_POINT('Ctrl Pts',(14.6639309312109,-36.5420065210792,1.12041585861625));
#8672=CARTESIAN_POINT('Ctrl Pts',(15.0060884047694,-36.5918976412677,1.18895624432295));
#8673=CARTESIAN_POINT('Ctrl Pts',(15.3482458783279,-36.6417887614562,1.25749663002964));
#8674=CARTESIAN_POINT('Ctrl Pts',(15.6928839357828,-36.6902477158643,1.2015057008556));
#8675=CARTESIAN_POINT('Ctrl Pts',(16.0375219932378,-36.7387066702723,1.14551477168157));
#8676=CARTESIAN_POINT('Ctrl Pts',(16.3376017974799,-36.8128913441675,0.976082217833403));
#8677=CARTESIAN_POINT('Ctrl Pts',(16.637681601722,-36.8870760180627,0.80664966398524));
#8678=CARTESIAN_POINT('Ctrl Pts',(16.8549896241618,-37.0090490024626,0.557333680706485));
#8679=CARTESIAN_POINT('Ctrl Pts',(17.0722976466017,-37.1310219868626,0.308017697427731));
#8680=CARTESIAN_POINT('Ctrl Pts',(17.1850143251652,-37.3133808118045,0.0281983728666177));
#8681=CARTESIAN_POINT('Ctrl Pts',(17.2977310037287,-37.4957396367464,-0.251620951694495));
#8682=CARTESIAN_POINT('Ctrl Pts',(17.304752374725,-37.7391216759643,-0.506521968549832));
#8683=CARTESIAN_POINT('Ctrl Pts',(17.3117737457213,-37.9825037151822,-0.761422985405168));
#8684=CARTESIAN_POINT('Ctrl Pts',(17.2329300973912,-38.2754599464222,-0.940919422010711));
#8685=CARTESIAN_POINT('Ctrl Pts',(17.1540864490611,-38.5684161776622,-1.12041585861625));
#8686=CARTESIAN_POINT('Ctrl Pts',(17.0262146897883,-38.8896788019527,-1.18895624432295));
#8687=CARTESIAN_POINT('Ctrl Pts',(16.8983429305155,-39.2109414262433,-1.25749663002964));
#8688=CARTESIAN_POINT('Ctrl Pts',(16.7679905873463,-39.5336362163143,-1.2015057008556));
#8689=CARTESIAN_POINT('Ctrl Pts',(16.637638244177,-39.8563310063852,-1.14551477168157));
#8690=CARTESIAN_POINT('Ctrl Pts',(16.5518441542207,-40.1533000769691,-0.976082217833403));
#8691=CARTESIAN_POINT('Ctrl Pts',(16.4660500642643,-40.450269147553,-0.80664966398524));
#8692=CARTESIAN_POINT('Ctrl Pts',(16.4630277561101,-40.6994499076321,-0.557333680706485));
#8693=CARTESIAN_POINT('Ctrl Pts',(16.460005447956,-40.9486306677112,-0.30801769742773));
#8694=CARTESIAN_POINT('Ctrl Pts',(16.5615744836782,-41.1374255872483,-0.0281983728666175));
#8695=CARTESIAN_POINT('Ctrl Pts',(16.6631435194004,-41.3262205067854,0.251620951694495));
#8696=CARTESIAN_POINT('Ctrl Pts',(16.8704078626898,-41.4539922120466,0.506521968549832));
#8697=CARTESIAN_POINT('Ctrl Pts',(17.0776722059792,-41.5817639173077,0.761422985405168));
#8698=CARTESIAN_POINT('Ctrl Pts',(17.370801568595,-41.6599614305468,0.940919422010711));
#8699=CARTESIAN_POINT('Ctrl Pts',(17.6639309312109,-41.7381589437859,1.12041585861625));
#8700=CARTESIAN_POINT('Ctrl Pts',(18.0060884047694,-41.7880500639744,1.18895624432295));
#8701=CARTESIAN_POINT('Ctrl Pts',(18.3482458783279,-41.8379411841628,1.25749663002964));
#8702=CARTESIAN_POINT('Ctrl Pts',(18.6928839357828,-41.8864001385709,1.2015057008556));
#8703=CARTESIAN_POINT('Ctrl Pts',(19.0375219932377,-41.934859092979,1.14551477168157));
#8704=CARTESIAN_POINT('Ctrl Pts',(19.3376017974798,-42.0090437668742,0.976082217833403));
#8705=CARTESIAN_POINT('Ctrl Pts',(19.6376816017219,-42.0832284407693,0.80664966398524));
#8706=CARTESIAN_POINT('Ctrl Pts',(19.8549896241618,-42.2052014251693,0.557333680706485));
#8707=CARTESIAN_POINT('Ctrl Pts',(20.0722976466017,-42.3271744095693,0.308017697427731));
#8708=CARTESIAN_POINT('Ctrl Pts',(20.1850143251651,-42.5095332345112,0.0281983728666177));
#8709=CARTESIAN_POINT('Ctrl Pts',(20.2977310037286,-42.6918920594531,-0.251620951694495));
#8710=CARTESIAN_POINT('Ctrl Pts',(20.3047523747249,-42.935274098671,-0.506521968549832));
#8711=CARTESIAN_POINT('Ctrl Pts',(20.3117737457212,-43.1786561378889,-0.761422985405168));
#8712=CARTESIAN_POINT('Ctrl Pts',(20.2329300973911,-43.4716123691288,-0.940919422010711));
#8713=CARTESIAN_POINT('Ctrl Pts',(20.154086449061,-43.7645686003688,-1.12041585861625));
#8714=CARTESIAN_POINT('Ctrl Pts',(20.0262146897883,-44.0858312246594,-1.18895624432295));
#8715=CARTESIAN_POINT('Ctrl Pts',(19.8983429305155,-44.40709384895,-1.25749663002964));
#8716=CARTESIAN_POINT('Ctrl Pts',(19.7679905873462,-44.7297886390209,-1.2015057008556));
#8717=CARTESIAN_POINT('Ctrl Pts',(19.637638244177,-45.0524834290919,-1.14551477168157));
#8718=CARTESIAN_POINT('Ctrl Pts',(19.5518441542206,-45.3494524996758,-0.976082217833403));
#8719=CARTESIAN_POINT('Ctrl Pts',(3.62216201968442,-19.1056780894973,-1.2339885196899));
#8720=CARTESIAN_POINT('Ctrl Pts',(3.48538897159447,-19.4320798752826,-0.910806095028249));
#8721=CARTESIAN_POINT('Ctrl Pts',(3.49420839053257,-19.6744238110373,-0.497425511654571));
#8722=CARTESIAN_POINT('Ctrl Pts',(3.50302780947066,-19.916767746792,-0.0840449282808927));
#8723=CARTESIAN_POINT('Ctrl Pts',(3.67691385823109,-20.0638104193845,0.337658719487502));
#8724=CARTESIAN_POINT('Ctrl Pts',(3.85079990699151,-20.2108530919771,0.759362367255897));
#8725=CARTESIAN_POINT('Ctrl Pts',(4.17653327792288,-20.2702266722385,1.10586550012264));
#8726=CARTESIAN_POINT('Ctrl Pts',(4.50226664885425,-20.3296002524999,1.45236863298939));
#8727=CARTESIAN_POINT('Ctrl Pts',(4.93655280986403,-20.3263008501883,1.65504205590818));
#8728=CARTESIAN_POINT('Ctrl Pts',(5.3708389708738,-20.3230014478767,1.85771547882697));
#8729=CARTESIAN_POINT('Ctrl Pts',(5.84888317848182,-20.2944383255823,1.87641723476232));
#8730=CARTESIAN_POINT('Ctrl Pts',(6.32692738608983,-20.265875203288,1.89511899069768));
#8731=CARTESIAN_POINT('Ctrl Pts',(6.77526807902992,-20.2544614131831,1.72614496752462));
#8732=CARTESIAN_POINT('Ctrl Pts',(7.22360877197,-20.2430476230782,1.55717094435156));
#8733=CARTESIAN_POINT('Ctrl Pts',(7.57466753434566,-20.2877995817719,1.2339885196899));
#8734=CARTESIAN_POINT('Ctrl Pts',(7.92572629672132,-20.3325515404656,0.910806095028249));
#8735=CARTESIAN_POINT('Ctrl Pts',(8.13119259206894,-20.46136134919,0.497425511654571));
#8736=CARTESIAN_POINT('Ctrl Pts',(8.33665888741656,-20.5901711579143,0.084044928280893));
#8737=CARTESIAN_POINT('Ctrl Pts',(8.37705855294184,-20.8142822298008,-0.337658719487502));
#8738=CARTESIAN_POINT('Ctrl Pts',(8.41745821846713,-21.0383933016873,-0.759362367255897));
#8739=CARTESIAN_POINT('Ctrl Pts',(8.30601056182147,-21.350173465905,-1.10586550012264));
#8740=CARTESIAN_POINT('Ctrl Pts',(8.19456290517582,-21.6619536301226,-1.45236863298939));
#8741=CARTESIAN_POINT('Ctrl Pts',(7.97456245845175,-22.0364067769132,-1.65504205590818));
#8742=CARTESIAN_POINT('Ctrl Pts',(7.75456201172769,-22.4108599237039,-1.85771547882697));
#8743=CARTESIAN_POINT('Ctrl Pts',(7.49080351840538,-22.8105767904773,-1.87641723476232));
#8744=CARTESIAN_POINT('Ctrl Pts',(7.22704502508308,-23.2102936572507,-1.89511899069768));
#8745=CARTESIAN_POINT('Ctrl Pts',(6.99299004642871,-23.5928611918346,-1.72614496752462));
#8746=CARTESIAN_POINT('Ctrl Pts',(6.75893506777434,-23.9754287264186,-1.55717094435156));
#8747=CARTESIAN_POINT('Ctrl Pts',(6.62216201968439,-24.3018305122039,-1.2339885196899));
#8748=CARTESIAN_POINT('Ctrl Pts',(6.48538897159444,-24.6282322979892,-0.910806095028249));
#8749=CARTESIAN_POINT('Ctrl Pts',(6.49420839053254,-24.8705762337439,-0.497425511654571));
#8750=CARTESIAN_POINT('Ctrl Pts',(6.50302780947063,-25.1129201694986,-0.0840449282808927));
#8751=CARTESIAN_POINT('Ctrl Pts',(6.67691385823105,-25.2599628420912,0.337658719487502));
#8752=CARTESIAN_POINT('Ctrl Pts',(6.85079990699148,-25.4070055146837,0.759362367255897));
#8753=CARTESIAN_POINT('Ctrl Pts',(7.17653327792285,-25.4663790949451,1.10586550012264));
#8754=CARTESIAN_POINT('Ctrl Pts',(7.50226664885422,-25.5257526752066,1.45236863298939));
#8755=CARTESIAN_POINT('Ctrl Pts',(7.936552809864,-25.5224532728949,1.65504205590818));
#8756=CARTESIAN_POINT('Ctrl Pts',(8.37083897087377,-25.5191538705833,1.85771547882697));
#8757=CARTESIAN_POINT('Ctrl Pts',(8.84888317848179,-25.490590748289,1.87641723476232));
#8758=CARTESIAN_POINT('Ctrl Pts',(9.3269273860898,-25.4620276259946,1.89511899069768));
#8759=CARTESIAN_POINT('Ctrl Pts',(9.77526807902988,-25.4506138358897,1.72614496752462));
#8760=CARTESIAN_POINT('Ctrl Pts',(10.22360877197,-25.4392000457848,1.55717094435156));
#8761=CARTESIAN_POINT('Ctrl Pts',(10.5746675343456,-25.4839520044785,1.2339885196899));
#8762=CARTESIAN_POINT('Ctrl Pts',(10.9257262967213,-25.5287039631723,0.910806095028249));
#8763=CARTESIAN_POINT('Ctrl Pts',(11.1311925920689,-25.6575137718966,0.497425511654571));
#8764=CARTESIAN_POINT('Ctrl Pts',(11.3366588874165,-25.786323580621,0.084044928280893));
#8765=CARTESIAN_POINT('Ctrl Pts',(11.3770585529418,-26.0104346525075,-0.337658719487502));
#8766=CARTESIAN_POINT('Ctrl Pts',(11.4174582184671,-26.234545724394,-0.759362367255897));
#8767=CARTESIAN_POINT('Ctrl Pts',(11.3060105618214,-26.5463258886116,-1.10586550012264));
#8768=CARTESIAN_POINT('Ctrl Pts',(11.1945629051758,-26.8581060528292,-1.45236863298939));
#8769=CARTESIAN_POINT('Ctrl Pts',(10.9745624584517,-27.2325591996199,-1.65504205590818));
#8770=CARTESIAN_POINT('Ctrl Pts',(10.7545620117277,-27.6070123464106,-1.85771547882697));
#8771=CARTESIAN_POINT('Ctrl Pts',(10.4908035184054,-28.0067292131839,-1.87641723476232));
#8772=CARTESIAN_POINT('Ctrl Pts',(10.227045025083,-28.4064460799573,-1.89511899069768));
#8773=CARTESIAN_POINT('Ctrl Pts',(9.99299004642868,-28.7890136145413,-1.72614496752462));
#8774=CARTESIAN_POINT('Ctrl Pts',(9.75893506777431,-29.1715811491253,-1.55717094435156));
#8775=CARTESIAN_POINT('Ctrl Pts',(9.62216201968436,-29.4979829349106,-1.2339885196899));
#8776=CARTESIAN_POINT('Ctrl Pts',(9.48538897159441,-29.8243847206959,-0.910806095028249));
#8777=CARTESIAN_POINT('Ctrl Pts',(9.4942083905325,-30.0667286564506,-0.497425511654571));
#8778=CARTESIAN_POINT('Ctrl Pts',(9.5030278094706,-30.3090725922053,-0.0840449282808927));
#8779=CARTESIAN_POINT('Ctrl Pts',(9.67691385823102,-30.4561152647978,0.337658719487502));
#8780=CARTESIAN_POINT('Ctrl Pts',(9.85079990699145,-30.6031579373903,0.759362367255897));
#8781=CARTESIAN_POINT('Ctrl Pts',(10.1765332779228,-30.6625315176518,1.10586550012264));
#8782=CARTESIAN_POINT('Ctrl Pts',(10.5022666488542,-30.7219050979132,1.45236863298939));
#8783=CARTESIAN_POINT('Ctrl Pts',(10.936552809864,-30.7186056956016,1.65504205590818));
#8784=CARTESIAN_POINT('Ctrl Pts',(11.3708389708737,-30.71530629329,1.85771547882697));
#8785=CARTESIAN_POINT('Ctrl Pts',(11.8488831784818,-30.6867431709956,1.87641723476232));
#8786=CARTESIAN_POINT('Ctrl Pts',(12.3269273860898,-30.6581800487013,1.89511899069768));
#8787=CARTESIAN_POINT('Ctrl Pts',(12.7752680790299,-30.6467662585964,1.72614496752462));
#8788=CARTESIAN_POINT('Ctrl Pts',(13.2236087719699,-30.6353524684915,1.55717094435156));
#8789=CARTESIAN_POINT('Ctrl Pts',(13.5746675343456,-30.6801044271852,1.2339885196899));
#8790=CARTESIAN_POINT('Ctrl Pts',(13.9257262967213,-30.7248563858789,0.910806095028249));
#8791=CARTESIAN_POINT('Ctrl Pts',(14.1311925920689,-30.8536661946033,0.497425511654571));
#8792=CARTESIAN_POINT('Ctrl Pts',(14.3366588874165,-30.9824760033276,0.084044928280893));
#8793=CARTESIAN_POINT('Ctrl Pts',(14.3770585529418,-31.2065870752141,-0.337658719487502));
#8794=CARTESIAN_POINT('Ctrl Pts',(14.4174582184671,-31.4306981471006,-0.759362367255897));
#8795=CARTESIAN_POINT('Ctrl Pts',(14.3060105618214,-31.7424783113183,-1.10586550012264));
#8796=CARTESIAN_POINT('Ctrl Pts',(14.1945629051758,-32.0542584755359,-1.45236863298939));
#8797=CARTESIAN_POINT('Ctrl Pts',(13.9745624584517,-32.4287116223265,-1.65504205590818));
#8798=CARTESIAN_POINT('Ctrl Pts',(13.7545620117276,-32.8031647691172,-1.85771547882697));
#8799=CARTESIAN_POINT('Ctrl Pts',(13.4908035184053,-33.2028816358906,-1.87641723476232));
#8800=CARTESIAN_POINT('Ctrl Pts',(13.227045025083,-33.602598502664,-1.89511899069768));
#8801=CARTESIAN_POINT('Ctrl Pts',(12.9929900464286,-33.9851660372479,-1.72614496752462));
#8802=CARTESIAN_POINT('Ctrl Pts',(12.7589350677743,-34.3677335718319,-1.55717094435156));
#8803=CARTESIAN_POINT('Ctrl Pts',(12.6221620196843,-34.6941353576172,-1.2339885196899));
#8804=CARTESIAN_POINT('Ctrl Pts',(12.4853889715944,-35.0205371434025,-0.910806095028249));
#8805=CARTESIAN_POINT('Ctrl Pts',(12.4942083905325,-35.2628810791572,-0.497425511654571));
#8806=CARTESIAN_POINT('Ctrl Pts',(12.5030278094706,-35.5052250149119,-0.0840449282808927));
#8807=CARTESIAN_POINT('Ctrl Pts',(12.676913858231,-35.6522676875044,0.337658719487502));
#8808=CARTESIAN_POINT('Ctrl Pts',(12.8507999069914,-35.799310360097,0.759362367255897));
#8809=CARTESIAN_POINT('Ctrl Pts',(13.1765332779228,-35.8586839403584,1.10586550012264));
#8810=CARTESIAN_POINT('Ctrl Pts',(13.5022666488542,-35.9180575206199,1.45236863298939));
#8811=CARTESIAN_POINT('Ctrl Pts',(13.9365528098639,-35.9147581183082,1.65504205590818));
#8812=CARTESIAN_POINT('Ctrl Pts',(14.3708389708737,-35.9114587159966,1.85771547882697));
#8813=CARTESIAN_POINT('Ctrl Pts',(14.8488831784817,-35.8828955937023,1.87641723476232));
#8814=CARTESIAN_POINT('Ctrl Pts',(15.3269273860897,-35.8543324714079,1.89511899069768));
#8815=CARTESIAN_POINT('Ctrl Pts',(15.7752680790298,-35.842918681303,1.72614496752462));
#8816=CARTESIAN_POINT('Ctrl Pts',(16.2236087719699,-35.8315048911981,1.55717094435156));
#8817=CARTESIAN_POINT('Ctrl Pts',(16.5746675343456,-35.8762568498918,1.2339885196899));
#8818=CARTESIAN_POINT('Ctrl Pts',(16.9257262967212,-35.9210088085856,0.910806095028249));
#8819=CARTESIAN_POINT('Ctrl Pts',(17.1311925920688,-36.0498186173099,0.497425511654571));
#8820=CARTESIAN_POINT('Ctrl Pts',(17.3366588874165,-36.1786284260343,0.084044928280893));
#8821=CARTESIAN_POINT('Ctrl Pts',(17.3770585529417,-36.4027394979208,-0.337658719487502));
#8822=CARTESIAN_POINT('Ctrl Pts',(17.417458218467,-36.6268505698073,-0.759362367255897));
#8823=CARTESIAN_POINT('Ctrl Pts',(17.3060105618214,-36.9386307340249,-1.10586550012264));
#8824=CARTESIAN_POINT('Ctrl Pts',(17.1945629051757,-37.2504108982425,-1.45236863298939));
#8825=CARTESIAN_POINT('Ctrl Pts',(16.9745624584517,-37.6248640450332,-1.65504205590818));
#8826=CARTESIAN_POINT('Ctrl Pts',(16.7545620117276,-37.9993171918239,-1.85771547882697));
#8827=CARTESIAN_POINT('Ctrl Pts',(16.4908035184053,-38.3990340585972,-1.87641723476232));
#8828=CARTESIAN_POINT('Ctrl Pts',(16.227045025083,-38.7987509253706,-1.89511899069768));
#8829=CARTESIAN_POINT('Ctrl Pts',(15.9929900464286,-39.1813184599546,-1.72614496752462));
#8830=CARTESIAN_POINT('Ctrl Pts',(15.7589350677742,-39.5638859945386,-1.55717094435156));
#8831=CARTESIAN_POINT('Ctrl Pts',(15.6221620196843,-39.8902877803239,-1.2339885196899));
#8832=CARTESIAN_POINT('Ctrl Pts',(15.4853889715943,-40.2166895661092,-0.910806095028249));
#8833=CARTESIAN_POINT('Ctrl Pts',(15.4942083905324,-40.4590335018639,-0.497425511654571));
#8834=CARTESIAN_POINT('Ctrl Pts',(15.5030278094705,-40.7013774376186,-0.0840449282808927));
#8835=CARTESIAN_POINT('Ctrl Pts',(15.676913858231,-40.8484201102111,0.337658719487502));
#8836=CARTESIAN_POINT('Ctrl Pts',(15.8507999069914,-40.9954627828037,0.759362367255897));
#8837=CARTESIAN_POINT('Ctrl Pts',(16.1765332779228,-41.0548363630651,1.10586550012264));
#8838=CARTESIAN_POINT('Ctrl Pts',(16.5022666488541,-41.1142099433265,1.45236863298939));
#8839=CARTESIAN_POINT('Ctrl Pts',(16.9365528098639,-41.1109105410149,1.65504205590818));
#8840=CARTESIAN_POINT('Ctrl Pts',(17.3708389708737,-41.1076111387033,1.85771547882697));
#8841=CARTESIAN_POINT('Ctrl Pts',(17.8488831784817,-41.0790480164089,1.87641723476232));
#8842=CARTESIAN_POINT('Ctrl Pts',(18.3269273860897,-41.0504848941146,1.89511899069768));
#8843=CARTESIAN_POINT('Ctrl Pts',(18.7752680790298,-41.0390711040097,1.72614496752462));
#8844=CARTESIAN_POINT('Ctrl Pts',(19.2236087719699,-41.0276573139048,1.55717094435156));
#8845=CARTESIAN_POINT('Ctrl Pts',(19.5746675343455,-41.0724092725985,1.2339885196899));
#8846=CARTESIAN_POINT('Ctrl Pts',(19.9257262967212,-41.1171612312922,0.910806095028249));
#8847=CARTESIAN_POINT('Ctrl Pts',(20.1311925920688,-41.2459710400166,0.497425511654571));
#8848=CARTESIAN_POINT('Ctrl Pts',(20.3366588874164,-41.374780848741,0.084044928280893));
#8849=CARTESIAN_POINT('Ctrl Pts',(20.3770585529417,-41.5988919206274,-0.337658719487502));
#8850=CARTESIAN_POINT('Ctrl Pts',(20.417458218467,-41.823002992514,-0.759362367255897));
#8851=CARTESIAN_POINT('Ctrl Pts',(20.3060105618213,-42.1347831567316,-1.10586550012264));
#8852=CARTESIAN_POINT('Ctrl Pts',(20.1945629051757,-42.4465633209492,-1.45236863298939));
#8853=CARTESIAN_POINT('Ctrl Pts',(19.9745624584516,-42.8210164677398,-1.65504205590818));
#8854=CARTESIAN_POINT('Ctrl Pts',(19.7545620117276,-43.1954696145305,-1.85771547882697));
#8855=CARTESIAN_POINT('Ctrl Pts',(19.4908035184053,-43.5951864813039,-1.87641723476232));
#8856=CARTESIAN_POINT('Ctrl Pts',(19.227045025083,-43.9949033480773,-1.89511899069768));
#8857=CARTESIAN_POINT('Ctrl Pts',(18.9929900464286,-44.3774708826612,-1.72614496752462));
#8858=CARTESIAN_POINT('Ctrl Pts',(18.7589350677742,-44.7600384172452,-1.55717094435156));
#8859=CARTESIAN_POINT('Ctrl Pts',(18.6221620196843,-45.0864402030305,-1.2339885196899));
#8860=CARTESIAN_POINT('Ctrl Pts',(2.69247988514806,-18.842665792852,-1.4918948215464));
#8861=CARTESIAN_POINT('Ctrl Pts',(2.50472787892454,-19.1985002938387,-1.01496252607126));
#8862=CARTESIAN_POINT('Ctrl Pts',(2.52538902495489,-19.434007405269,-0.437517342602656));
#8863=CARTESIAN_POINT('Ctrl Pts',(2.54605017098523,-19.6695145166993,0.139927840865946));
#8864=CARTESIAN_POINT('Ctrl Pts',(2.79225323278385,-19.7748049423473,0.703515811841622));
#8865=CARTESIAN_POINT('Ctrl Pts',(3.03845629458247,-19.8800953679953,1.2671037828173));
#8866=CARTESIAN_POINT('Ctrl Pts',(3.48265869315581,-19.871070823257,1.70520903169545));
#8867=CARTESIAN_POINT('Ctrl Pts',(3.92686109172914,-19.8620462785187,2.1433142805736));
#8868=CARTESIAN_POINT('Ctrl Pts',(4.50230405113288,-19.7772499606563,2.36916468980564));
#8869=CARTESIAN_POINT('Ctrl Pts',(5.07774701053662,-19.692453642794,2.59501509903768));
#8870=CARTESIAN_POINT('Ctrl Pts',(5.69167795219416,-19.5854362780169,2.5638782252017));
#8871=CARTESIAN_POINT('Ctrl Pts',(6.30560889385169,-19.4784189132398,2.53274135136572));
#8872=CARTESIAN_POINT('Ctrl Pts',(6.85765222227691,-19.4071323786218,2.25078423419363));
#8873=CARTESIAN_POINT('Ctrl Pts',(7.40969555070213,-19.3358458440039,1.96882711702155));
#8874=CARTESIAN_POINT('Ctrl Pts',(7.81173327121136,-19.3511650874962,1.4918948215464));
#8875=CARTESIAN_POINT('Ctrl Pts',(8.21377099172059,-19.3664843309885,1.01496252607126));
#8876=CARTESIAN_POINT('Ctrl Pts',(8.40739555997595,-19.5021309640373,0.437517342602656));
#8877=CARTESIAN_POINT('Ctrl Pts',(8.60102012823132,-19.637777597086,-0.139927840865945));
#8878=CARTESIAN_POINT('Ctrl Pts',(8.56910278071841,-19.9036409159171,-0.703515811841622));
#8879=CARTESIAN_POINT('Ctrl Pts',(8.5371854332055,-20.1695042347482,-1.2671037828173));
#8880=CARTESIAN_POINT('Ctrl Pts',(8.30726874891788,-20.5496825239655,-1.70520903169545));
#8881=CARTESIAN_POINT('Ctrl Pts',(8.07735206463027,-20.9298608131829,-2.1433142805736));
#8882=CARTESIAN_POINT('Ctrl Pts',(7.71619481951224,-21.3858108755242,-2.36916468980564));
#8883=CARTESIAN_POINT('Ctrl Pts',(7.35503757439421,-21.8417609378656,-2.59501509903768));
#8884=CARTESIAN_POINT('Ctrl Pts',(6.95539234702238,-22.3199320471218,-2.5638782252017));
#8885=CARTESIAN_POINT('Ctrl Pts',(6.55574711965056,-22.7981031563779,-2.53274135136572));
#8886=CARTESIAN_POINT('Ctrl Pts',(6.21798950551105,-23.2405434354749,-2.25078423419363));
#8887=CARTESIAN_POINT('Ctrl Pts',(5.88023189137154,-23.6829837145719,-1.96882711702155));
#8888=CARTESIAN_POINT('Ctrl Pts',(5.69247988514803,-24.0388182155586,-1.4918948215464));
#8889=CARTESIAN_POINT('Ctrl Pts',(5.50472787892451,-24.3946527165454,-1.01496252607126));
#8890=CARTESIAN_POINT('Ctrl Pts',(5.52538902495486,-24.6301598279757,-0.437517342602656));
#8891=CARTESIAN_POINT('Ctrl Pts',(5.5460501709852,-24.865666939406,0.139927840865946));
#8892=CARTESIAN_POINT('Ctrl Pts',(5.79225323278382,-24.970957365054,0.703515811841622));
#8893=CARTESIAN_POINT('Ctrl Pts',(6.03845629458244,-25.0762477907019,1.2671037828173));
#8894=CARTESIAN_POINT('Ctrl Pts',(6.48265869315577,-25.0672232459636,1.70520903169545));
#8895=CARTESIAN_POINT('Ctrl Pts',(6.92686109172911,-25.0581987012253,2.1433142805736));
#8896=CARTESIAN_POINT('Ctrl Pts',(7.50230405113285,-24.973402383363,2.36916468980564));
#8897=CARTESIAN_POINT('Ctrl Pts',(8.07774701053659,-24.8886060655007,2.59501509903768));
#8898=CARTESIAN_POINT('Ctrl Pts',(8.69167795219413,-24.7815887007236,2.5638782252017));
#8899=CARTESIAN_POINT('Ctrl Pts',(9.30560889385166,-24.6745713359464,2.53274135136572));
#8900=CARTESIAN_POINT('Ctrl Pts',(9.85765222227688,-24.6032848013285,2.25078423419363));
#8901=CARTESIAN_POINT('Ctrl Pts',(10.4096955507021,-24.5319982667106,1.96882711702155));
#8902=CARTESIAN_POINT('Ctrl Pts',(10.8117332712113,-24.5473175102029,1.4918948215464));
#8903=CARTESIAN_POINT('Ctrl Pts',(11.2137709917206,-24.5626367536952,1.01496252607126));
#8904=CARTESIAN_POINT('Ctrl Pts',(11.4073955599759,-24.6982833867439,0.437517342602656));
#8905=CARTESIAN_POINT('Ctrl Pts',(11.6010201282313,-24.8339300197927,-0.139927840865945));
#8906=CARTESIAN_POINT('Ctrl Pts',(11.5691027807184,-25.0997933386238,-0.703515811841622));
#8907=CARTESIAN_POINT('Ctrl Pts',(11.5371854332055,-25.3656566574548,-1.2671037828173));
#8908=CARTESIAN_POINT('Ctrl Pts',(11.3072687489179,-25.7458349466722,-1.70520903169545));
#8909=CARTESIAN_POINT('Ctrl Pts',(11.0773520646302,-26.1260132358895,-2.1433142805736));
#8910=CARTESIAN_POINT('Ctrl Pts',(10.7161948195122,-26.5819632982309,-2.36916468980564));
#8911=CARTESIAN_POINT('Ctrl Pts',(10.3550375743942,-27.0379133605723,-2.59501509903768));
#8912=CARTESIAN_POINT('Ctrl Pts',(9.95539234702235,-27.5160844698284,-2.5638782252017));
#8913=CARTESIAN_POINT('Ctrl Pts',(9.55574711965053,-27.9942555790846,-2.53274135136572));
#8914=CARTESIAN_POINT('Ctrl Pts',(9.21798950551102,-28.4366958581816,-2.25078423419363));
#8915=CARTESIAN_POINT('Ctrl Pts',(8.88023189137151,-28.8791361372786,-1.96882711702155));
#8916=CARTESIAN_POINT('Ctrl Pts',(8.692479885148,-29.2349706382653,-1.4918948215464));
#8917=CARTESIAN_POINT('Ctrl Pts',(8.50472787892448,-29.590805139252,-1.01496252607126));
#8918=CARTESIAN_POINT('Ctrl Pts',(8.52538902495483,-29.8263122506823,-0.437517342602656));
#8919=CARTESIAN_POINT('Ctrl Pts',(8.54605017098517,-30.0618193621126,0.139927840865946));
#8920=CARTESIAN_POINT('Ctrl Pts',(8.79225323278379,-30.1671097877606,0.703515811841622));
#8921=CARTESIAN_POINT('Ctrl Pts',(9.03845629458241,-30.2724002134086,1.2671037828173));
#8922=CARTESIAN_POINT('Ctrl Pts',(9.48265869315574,-30.2633756686703,1.70520903169545));
#8923=CARTESIAN_POINT('Ctrl Pts',(9.92686109172908,-30.254351123932,2.1433142805736));
#8924=CARTESIAN_POINT('Ctrl Pts',(10.5023040511328,-30.1695548060697,2.36916468980564));
#8925=CARTESIAN_POINT('Ctrl Pts',(11.0777470105366,-30.0847584882073,2.59501509903768));
#8926=CARTESIAN_POINT('Ctrl Pts',(11.6916779521941,-29.9777411234302,2.5638782252017));
#8927=CARTESIAN_POINT('Ctrl Pts',(12.3056088938516,-29.8707237586531,2.53274135136572));
#8928=CARTESIAN_POINT('Ctrl Pts',(12.8576522222768,-29.7994372240352,2.25078423419363));
#8929=CARTESIAN_POINT('Ctrl Pts',(13.4096955507021,-29.7281506894172,1.96882711702155));
#8930=CARTESIAN_POINT('Ctrl Pts',(13.8117332712113,-29.7434699329095,1.4918948215464));
#8931=CARTESIAN_POINT('Ctrl Pts',(14.2137709917205,-29.7587891764018,1.01496252607126));
#8932=CARTESIAN_POINT('Ctrl Pts',(14.4073955599759,-29.8944358094506,0.437517342602656));
#8933=CARTESIAN_POINT('Ctrl Pts',(14.6010201282313,-30.0300824424993,-0.139927840865945));
#8934=CARTESIAN_POINT('Ctrl Pts',(14.5691027807183,-30.2959457613304,-0.703515811841622));
#8935=CARTESIAN_POINT('Ctrl Pts',(14.5371854332054,-30.5618090801615,-1.2671037828173));
#8936=CARTESIAN_POINT('Ctrl Pts',(14.3072687489178,-30.9419873693788,-1.70520903169545));
#8937=CARTESIAN_POINT('Ctrl Pts',(14.0773520646302,-31.3221656585962,-2.1433142805736));
#8938=CARTESIAN_POINT('Ctrl Pts',(13.7161948195122,-31.7781157209375,-2.36916468980564));
#8939=CARTESIAN_POINT('Ctrl Pts',(13.3550375743941,-32.2340657832789,-2.59501509903768));
#8940=CARTESIAN_POINT('Ctrl Pts',(12.9553923470223,-32.7122368925351,-2.5638782252017));
#8941=CARTESIAN_POINT('Ctrl Pts',(12.5557471196505,-33.1904080017912,-2.53274135136572));
#8942=CARTESIAN_POINT('Ctrl Pts',(12.217989505511,-33.6328482808882,-2.25078423419363));
#8943=CARTESIAN_POINT('Ctrl Pts',(11.8802318913715,-34.0752885599852,-1.96882711702155));
#8944=CARTESIAN_POINT('Ctrl Pts',(11.692479885148,-34.4311230609719,-1.4918948215464));
#8945=CARTESIAN_POINT('Ctrl Pts',(11.5047278789244,-34.7869575619587,-1.01496252607126));
#8946=CARTESIAN_POINT('Ctrl Pts',(11.5253890249548,-35.022464673389,-0.437517342602656));
#8947=CARTESIAN_POINT('Ctrl Pts',(11.5460501709851,-35.2579717848193,0.139927840865946));
#8948=CARTESIAN_POINT('Ctrl Pts',(11.7922532327838,-35.3632622104672,0.703515811841622));
#8949=CARTESIAN_POINT('Ctrl Pts',(12.0384562945824,-35.4685526361152,1.2671037828173));
#8950=CARTESIAN_POINT('Ctrl Pts',(12.4826586931557,-35.4595280913769,1.70520903169545));
#8951=CARTESIAN_POINT('Ctrl Pts',(12.926861091729,-35.4505035466386,2.1433142805736));
#8952=CARTESIAN_POINT('Ctrl Pts',(13.5023040511328,-35.3657072287763,2.36916468980564));
#8953=CARTESIAN_POINT('Ctrl Pts',(14.0777470105365,-35.280910910914,2.59501509903768));
#8954=CARTESIAN_POINT('Ctrl Pts',(14.6916779521941,-35.1738935461369,2.5638782252017));
#8955=CARTESIAN_POINT('Ctrl Pts',(15.3056088938516,-35.0668761813597,2.53274135136572));
#8956=CARTESIAN_POINT('Ctrl Pts',(15.8576522222768,-34.9955896467418,2.25078423419363));
#8957=CARTESIAN_POINT('Ctrl Pts',(16.409695550702,-34.9243031121239,1.96882711702155));
#8958=CARTESIAN_POINT('Ctrl Pts',(16.8117332712113,-34.9396223556162,1.4918948215464));
#8959=CARTESIAN_POINT('Ctrl Pts',(17.2137709917205,-34.9549415991085,1.01496252607126));
#8960=CARTESIAN_POINT('Ctrl Pts',(17.4073955599759,-35.0905882321572,0.437517342602656));
#8961=CARTESIAN_POINT('Ctrl Pts',(17.6010201282312,-35.226234865206,-0.139927840865945));
#8962=CARTESIAN_POINT('Ctrl Pts',(17.5691027807183,-35.4920981840371,-0.703515811841622));
#8963=CARTESIAN_POINT('Ctrl Pts',(17.5371854332054,-35.7579615028681,-1.2671037828173));
#8964=CARTESIAN_POINT('Ctrl Pts',(17.3072687489178,-36.1381397920855,-1.70520903169545));
#8965=CARTESIAN_POINT('Ctrl Pts',(17.0773520646302,-36.5183180813028,-2.1433142805736));
#8966=CARTESIAN_POINT('Ctrl Pts',(16.7161948195121,-36.9742681436442,-2.36916468980564));
#8967=CARTESIAN_POINT('Ctrl Pts',(16.3550375743941,-37.4302182059856,-2.59501509903768));
#8968=CARTESIAN_POINT('Ctrl Pts',(15.9553923470223,-37.9083893152417,-2.5638782252017));
#8969=CARTESIAN_POINT('Ctrl Pts',(15.5557471196505,-38.3865604244979,-2.53274135136572));
#8970=CARTESIAN_POINT('Ctrl Pts',(15.217989505511,-38.8290007035949,-2.25078423419363));
#8971=CARTESIAN_POINT('Ctrl Pts',(14.8802318913715,-39.2714409826919,-1.96882711702155));
#8972=CARTESIAN_POINT('Ctrl Pts',(14.6924798851479,-39.6272754836786,-1.4918948215464));
#8973=CARTESIAN_POINT('Ctrl Pts',(14.5047278789244,-39.9831099846653,-1.01496252607126));
#8974=CARTESIAN_POINT('Ctrl Pts',(14.5253890249548,-40.2186170960956,-0.437517342602656));
#8975=CARTESIAN_POINT('Ctrl Pts',(14.5460501709851,-40.4541242075259,0.139927840865946));
#8976=CARTESIAN_POINT('Ctrl Pts',(14.7922532327837,-40.5594146331739,0.703515811841622));
#8977=CARTESIAN_POINT('Ctrl Pts',(15.0384562945823,-40.6647050588219,1.2671037828173));
#8978=CARTESIAN_POINT('Ctrl Pts',(15.4826586931557,-40.6556805140836,1.70520903169545));
#8979=CARTESIAN_POINT('Ctrl Pts',(15.926861091729,-40.6466559693453,2.1433142805736));
#8980=CARTESIAN_POINT('Ctrl Pts',(16.5023040511328,-40.5618596514829,2.36916468980564));
#8981=CARTESIAN_POINT('Ctrl Pts',(17.0777470105365,-40.4770633336206,2.59501509903768));
#8982=CARTESIAN_POINT('Ctrl Pts',(17.691677952194,-40.3700459688435,2.5638782252017));
#8983=CARTESIAN_POINT('Ctrl Pts',(18.3056088938516,-40.2630286040664,2.53274135136572));
#8984=CARTESIAN_POINT('Ctrl Pts',(18.8576522222768,-40.1917420694485,2.25078423419363));
#8985=CARTESIAN_POINT('Ctrl Pts',(19.409695550702,-40.1204555348305,1.96882711702155));
#8986=CARTESIAN_POINT('Ctrl Pts',(19.8117332712112,-40.1357747783228,1.4918948215464));
#8987=CARTESIAN_POINT('Ctrl Pts',(20.2137709917205,-40.1510940218152,1.01496252607126));
#8988=CARTESIAN_POINT('Ctrl Pts',(20.4073955599758,-40.2867406548639,0.437517342602656));
#8989=CARTESIAN_POINT('Ctrl Pts',(20.6010201282312,-40.4223872879126,-0.139927840865945));
#8990=CARTESIAN_POINT('Ctrl Pts',(20.5691027807183,-40.6882506067437,-0.703515811841622));
#8991=CARTESIAN_POINT('Ctrl Pts',(20.5371854332054,-40.9541139255748,-1.2671037828173));
#8992=CARTESIAN_POINT('Ctrl Pts',(20.3072687489178,-41.3342922147921,-1.70520903169545));
#8993=CARTESIAN_POINT('Ctrl Pts',(20.0773520646301,-41.7144705040095,-2.1433142805736));
#8994=CARTESIAN_POINT('Ctrl Pts',(19.7161948195121,-42.1704205663508,-2.36916468980564));
#8995=CARTESIAN_POINT('Ctrl Pts',(19.3550375743941,-42.6263706286922,-2.59501509903768));
#8996=CARTESIAN_POINT('Ctrl Pts',(18.9553923470223,-43.1045417379484,-2.5638782252017));
#8997=CARTESIAN_POINT('Ctrl Pts',(18.5557471196504,-43.5827128472045,-2.53274135136572));
#8998=CARTESIAN_POINT('Ctrl Pts',(18.2179895055109,-44.0251531263015,-2.25078423419363));
#8999=CARTESIAN_POINT('Ctrl Pts',(17.8802318913714,-44.4675934053985,-1.96882711702155));
#9000=CARTESIAN_POINT('Ctrl Pts',(17.6924798851479,-44.8234279063853,-1.4918948215464));
#9001=CARTESIAN_POINT('Ctrl Pts',(2.69247988514806,-19.542807947216,-2.20589829750609));
#9002=CARTESIAN_POINT('Ctrl Pts',(2.3635946338423,-19.9801257652426,-1.64906456309142));
#9003=CARTESIAN_POINT('Ctrl Pts',(2.28712243231041,-20.2717128410352,-0.928922098091803));
#9004=CARTESIAN_POINT('Ctrl Pts',(2.21065023077853,-20.5632999168279,-0.208779633092189));
#9005=CARTESIAN_POINT('Ctrl Pts',(2.42295829328197,-20.6881596294431,0.532038515331462));
#9006=CARTESIAN_POINT('Ctrl Pts',(2.63526635578541,-20.8130193420583,1.27285666375511));
#9007=CARTESIAN_POINT('Ctrl Pts',(3.1155254236359,-20.7831774696068,1.88762237576914));
#9008=CARTESIAN_POINT('Ctrl Pts',(3.5957844914864,-20.7533355971552,2.50238808778318));
#9009=CARTESIAN_POINT('Ctrl Pts',(4.27009432318328,-20.6114584639605,2.86933947451654));
#9010=CARTESIAN_POINT('Ctrl Pts',(4.94440415488017,-20.4695813307658,3.2362908612499));
#9011=CARTESIAN_POINT('Ctrl Pts',(5.70043037526654,-20.280525218564,3.28274870019663));
#9012=CARTESIAN_POINT('Ctrl Pts',(6.45645659565292,-20.0914691063622,3.32920653914337));
#9013=CARTESIAN_POINT('Ctrl Pts',(7.1656798966062,-19.929434672294,3.04596928553206));
#9014=CARTESIAN_POINT('Ctrl Pts',(7.87490319755949,-19.7674002382258,2.76273203192075));
#9015=CARTESIAN_POINT('Ctrl Pts',(8.41807416315096,-19.7012361646782,2.20589829750609));
#9016=CARTESIAN_POINT('Ctrl Pts',(8.96124512874244,-19.6350720911307,1.64906456309142));
#9017=CARTESIAN_POINT('Ctrl Pts',(9.25200304456004,-19.7146387598171,0.928922098091803));
#9018=CARTESIAN_POINT('Ctrl Pts',(9.54276096037763,-19.7942054285035,0.20877963309219));
#9019=CARTESIAN_POINT('Ctrl Pts',(9.5447386121599,-20.0404994603673,-0.532038515331461));
#9020=CARTESIAN_POINT('Ctrl Pts',(9.54671626394218,-20.2867934922312,-1.27285666375511));
#9021=CARTESIAN_POINT('Ctrl Pts',(9.28074291037739,-20.6877891091618,-1.88762237576914));
#9022=CARTESIAN_POINT('Ctrl Pts',(9.01476955681261,-21.0887847260924,-2.50238808778318));
#9023=CARTESIAN_POINT('Ctrl Pts',(8.55474543940143,-21.6018156037661,-2.86933947451654));
#9024=CARTESIAN_POINT('Ctrl Pts',(8.09472132199027,-22.1148464814399,-3.2362908612499));
#9025=CARTESIAN_POINT('Ctrl Pts',(7.5529808158896,-22.6750563381207,-3.28274870019663));
#9026=CARTESIAN_POINT('Ctrl Pts',(7.01124030978894,-23.2352661948015,-3.32920653914337));
#9027=CARTESIAN_POINT('Ctrl Pts',(6.51630272312137,-23.7684543733488,-3.04596928553206));
#9028=CARTESIAN_POINT('Ctrl Pts',(6.02136513645379,-24.3016425518961,-2.76273203192075));
#9029=CARTESIAN_POINT('Ctrl Pts',(5.69247988514803,-24.7389603699227,-2.20589829750609));
#9030=CARTESIAN_POINT('Ctrl Pts',(5.36359463384226,-25.1762781879492,-1.64906456309142));
#9031=CARTESIAN_POINT('Ctrl Pts',(5.28712243231038,-25.4678652637419,-0.928922098091803));
#9032=CARTESIAN_POINT('Ctrl Pts',(5.2106502307785,-25.7594523395345,-0.208779633092189));
#9033=CARTESIAN_POINT('Ctrl Pts',(5.42295829328193,-25.8843120521498,0.532038515331462));
#9034=CARTESIAN_POINT('Ctrl Pts',(5.63526635578538,-26.009171764765,1.27285666375511));
#9035=CARTESIAN_POINT('Ctrl Pts',(6.11552542363587,-25.9793298923134,1.88762237576914));
#9036=CARTESIAN_POINT('Ctrl Pts',(6.59578449148637,-25.9494880198619,2.50238808778318));
#9037=CARTESIAN_POINT('Ctrl Pts',(7.27009432318325,-25.8076108866672,2.86933947451654));
#9038=CARTESIAN_POINT('Ctrl Pts',(7.94440415488013,-25.6657337534725,3.2362908612499));
#9039=CARTESIAN_POINT('Ctrl Pts',(8.70043037526651,-25.4766776412707,3.28274870019663));
#9040=CARTESIAN_POINT('Ctrl Pts',(9.45645659565288,-25.2876215290689,3.32920653914337));
#9041=CARTESIAN_POINT('Ctrl Pts',(10.1656798966062,-25.1255870950007,3.04596928553206));
#9042=CARTESIAN_POINT('Ctrl Pts',(10.8749031975595,-24.9635526609324,2.76273203192075));
#9043=CARTESIAN_POINT('Ctrl Pts',(11.4180741631509,-24.8973885873849,2.20589829750609));
#9044=CARTESIAN_POINT('Ctrl Pts',(11.9612451287424,-24.8312245138374,1.64906456309142));
#9045=CARTESIAN_POINT('Ctrl Pts',(12.25200304456,-24.9107911825238,0.928922098091803));
#9046=CARTESIAN_POINT('Ctrl Pts',(12.5427609603776,-24.9903578512102,0.20877963309219));
#9047=CARTESIAN_POINT('Ctrl Pts',(12.5447386121599,-25.236651883074,-0.532038515331461));
#9048=CARTESIAN_POINT('Ctrl Pts',(12.5467162639421,-25.4829459149378,-1.27285666375511));
#9049=CARTESIAN_POINT('Ctrl Pts',(12.2807429103774,-25.8839415318684,-1.88762237576914));
#9050=CARTESIAN_POINT('Ctrl Pts',(12.0147695568126,-26.284937148799,-2.50238808778318));
#9051=CARTESIAN_POINT('Ctrl Pts',(11.5547454394014,-26.7979680264728,-2.86933947451654));
#9052=CARTESIAN_POINT('Ctrl Pts',(11.0947213219902,-27.3109989041465,-3.2362908612499));
#9053=CARTESIAN_POINT('Ctrl Pts',(10.5529808158896,-27.8712087608274,-3.28274870019663));
#9054=CARTESIAN_POINT('Ctrl Pts',(10.0112403097889,-28.4314186175082,-3.32920653914337));
#9055=CARTESIAN_POINT('Ctrl Pts',(9.51630272312133,-28.9646067960555,-3.04596928553206));
#9056=CARTESIAN_POINT('Ctrl Pts',(9.02136513645376,-29.4977949746027,-2.76273203192075));
#9057=CARTESIAN_POINT('Ctrl Pts',(8.692479885148,-29.9351127926293,-2.20589829750609));
#9058=CARTESIAN_POINT('Ctrl Pts',(8.36359463384224,-30.3724306106559,-1.64906456309142));
#9059=CARTESIAN_POINT('Ctrl Pts',(8.28712243231035,-30.6640176864485,-0.928922098091803));
#9060=CARTESIAN_POINT('Ctrl Pts',(8.21065023077846,-30.9556047622412,-0.208779633092189));
#9061=CARTESIAN_POINT('Ctrl Pts',(8.4229582932819,-31.0804644748564,0.532038515331462));
#9062=CARTESIAN_POINT('Ctrl Pts',(8.63526635578534,-31.2053241874716,1.27285666375511));
#9063=CARTESIAN_POINT('Ctrl Pts',(9.11552542363584,-31.1754823150201,1.88762237576914));
#9064=CARTESIAN_POINT('Ctrl Pts',(9.59578449148634,-31.1456404425685,2.50238808778318));
#9065=CARTESIAN_POINT('Ctrl Pts',(10.2700943231832,-31.0037633093738,2.86933947451654));
#9066=CARTESIAN_POINT('Ctrl Pts',(10.9444041548801,-30.8618861761791,3.2362908612499));
#9067=CARTESIAN_POINT('Ctrl Pts',(11.7004303752665,-30.6728300639773,3.28274870019663));
#9068=CARTESIAN_POINT('Ctrl Pts',(12.4564565956529,-30.4837739517755,3.32920653914337));
#9069=CARTESIAN_POINT('Ctrl Pts',(13.1656798966061,-30.3217395177073,3.04596928553206));
#9070=CARTESIAN_POINT('Ctrl Pts',(13.8749031975594,-30.1597050836391,2.76273203192075));
#9071=CARTESIAN_POINT('Ctrl Pts',(14.4180741631509,-30.0935410100915,2.20589829750609));
#9072=CARTESIAN_POINT('Ctrl Pts',(14.9612451287424,-30.027376936544,1.64906456309142));
#9073=CARTESIAN_POINT('Ctrl Pts',(15.25200304456,-30.1069436052304,0.928922098091803));
#9074=CARTESIAN_POINT('Ctrl Pts',(15.5427609603776,-30.1865102739168,0.20877963309219));
#9075=CARTESIAN_POINT('Ctrl Pts',(15.5447386121598,-30.4328043057806,-0.532038515331461));
#9076=CARTESIAN_POINT('Ctrl Pts',(15.5467162639421,-30.6790983376445,-1.27285666375511));
#9077=CARTESIAN_POINT('Ctrl Pts',(15.2807429103773,-31.0800939545751,-1.88762237576914));
#9078=CARTESIAN_POINT('Ctrl Pts',(15.0147695568125,-31.4810895715057,-2.50238808778318));
#9079=CARTESIAN_POINT('Ctrl Pts',(14.5547454394014,-31.9941204491794,-2.86933947451654));
#9080=CARTESIAN_POINT('Ctrl Pts',(14.0947213219902,-32.5071513268532,-3.2362908612499));
#9081=CARTESIAN_POINT('Ctrl Pts',(13.5529808158895,-33.067361183534,-3.28274870019663));
#9082=CARTESIAN_POINT('Ctrl Pts',(13.0112403097889,-33.6275710402148,-3.32920653914337));
#9083=CARTESIAN_POINT('Ctrl Pts',(12.5163027231213,-34.1607592187621,-3.04596928553206));
#9084=CARTESIAN_POINT('Ctrl Pts',(12.0213651364537,-34.6939473973094,-2.76273203192075));
#9085=CARTESIAN_POINT('Ctrl Pts',(11.692479885148,-35.131265215336,-2.20589829750609));
#9086=CARTESIAN_POINT('Ctrl Pts',(11.3635946338422,-35.5685830333625,-1.64906456309142));
#9087=CARTESIAN_POINT('Ctrl Pts',(11.2871224323103,-35.8601701091552,-0.928922098091803));
#9088=CARTESIAN_POINT('Ctrl Pts',(11.2106502307784,-36.1517571849478,-0.208779633092189));
#9089=CARTESIAN_POINT('Ctrl Pts',(11.4229582932819,-36.2766168975631,0.532038515331462));
#9090=CARTESIAN_POINT('Ctrl Pts',(11.6352663557853,-36.4014766101783,1.27285666375511));
#9091=CARTESIAN_POINT('Ctrl Pts',(12.1155254236358,-36.3716347377267,1.88762237576914));
#9092=CARTESIAN_POINT('Ctrl Pts',(12.5957844914863,-36.3417928652752,2.50238808778318));
#9093=CARTESIAN_POINT('Ctrl Pts',(13.2700943231832,-36.1999157320805,2.86933947451654));
#9094=CARTESIAN_POINT('Ctrl Pts',(13.9444041548801,-36.0580385988858,3.2362908612499));
#9095=CARTESIAN_POINT('Ctrl Pts',(14.7004303752664,-35.868982486684,3.28274870019663));
#9096=CARTESIAN_POINT('Ctrl Pts',(15.4564565956528,-35.6799263744822,3.32920653914337));
#9097=CARTESIAN_POINT('Ctrl Pts',(16.1656798966061,-35.517891940414,3.04596928553206));
#9098=CARTESIAN_POINT('Ctrl Pts',(16.8749031975594,-35.3558575063457,2.76273203192075));
#9099=CARTESIAN_POINT('Ctrl Pts',(17.4180741631509,-35.2896934327982,2.20589829750609));
#9100=CARTESIAN_POINT('Ctrl Pts',(17.9612451287423,-35.2235293592507,1.64906456309142));
#9101=CARTESIAN_POINT('Ctrl Pts',(18.2520030445599,-35.3030960279371,0.928922098091803));
#9102=CARTESIAN_POINT('Ctrl Pts',(18.5427609603775,-35.3826626966235,0.20877963309219));
#9103=CARTESIAN_POINT('Ctrl Pts',(18.5447386121598,-35.6289567284873,-0.532038515331461));
#9104=CARTESIAN_POINT('Ctrl Pts',(18.5467162639421,-35.8752507603511,-1.27285666375511));
#9105=CARTESIAN_POINT('Ctrl Pts',(18.2807429103773,-36.2762463772817,-1.88762237576914));
#9106=CARTESIAN_POINT('Ctrl Pts',(18.0147695568125,-36.6772419942123,-2.50238808778318));
#9107=CARTESIAN_POINT('Ctrl Pts',(17.5547454394013,-37.1902728718861,-2.86933947451654));
#9108=CARTESIAN_POINT('Ctrl Pts',(17.0947213219902,-37.7033037495598,-3.2362908612499));
#9109=CARTESIAN_POINT('Ctrl Pts',(16.5529808158895,-38.2635136062407,-3.28274870019663));
#9110=CARTESIAN_POINT('Ctrl Pts',(16.0112403097889,-38.8237234629215,-3.32920653914337));
#9111=CARTESIAN_POINT('Ctrl Pts',(15.5163027231213,-39.3569116414688,-3.04596928553206));
#9112=CARTESIAN_POINT('Ctrl Pts',(15.0213651364537,-39.890099820016,-2.76273203192075));
#9113=CARTESIAN_POINT('Ctrl Pts',(14.6924798851479,-40.3274176380426,-2.20589829750609));
#9114=CARTESIAN_POINT('Ctrl Pts',(14.3635946338422,-40.7647354560692,-1.64906456309142));
#9115=CARTESIAN_POINT('Ctrl Pts',(14.2871224323103,-41.0563225318618,-0.928922098091803));
#9116=CARTESIAN_POINT('Ctrl Pts',(14.2106502307784,-41.3479096076545,-0.208779633092189));
#9117=CARTESIAN_POINT('Ctrl Pts',(14.4229582932818,-41.4727693202697,0.532038515331462));
#9118=CARTESIAN_POINT('Ctrl Pts',(14.6352663557853,-41.5976290328849,1.27285666375511));
#9119=CARTESIAN_POINT('Ctrl Pts',(15.1155254236358,-41.5677871604334,1.88762237576914));
#9120=CARTESIAN_POINT('Ctrl Pts',(15.5957844914863,-41.5379452879818,2.50238808778318));
#9121=CARTESIAN_POINT('Ctrl Pts',(16.2700943231832,-41.3960681547871,2.86933947451654));
#9122=CARTESIAN_POINT('Ctrl Pts',(16.94440415488,-41.2541910215924,3.2362908612499));
#9123=CARTESIAN_POINT('Ctrl Pts',(17.7004303752664,-41.0651349093906,3.28274870019663));
#9124=CARTESIAN_POINT('Ctrl Pts',(18.4564565956528,-40.8760787971888,3.32920653914337));
#9125=CARTESIAN_POINT('Ctrl Pts',(19.1656798966061,-40.7140443631206,3.04596928553206));
#9126=CARTESIAN_POINT('Ctrl Pts',(19.8749031975594,-40.5520099290524,2.76273203192075));
#9127=CARTESIAN_POINT('Ctrl Pts',(20.4180741631508,-40.4858458555049,2.20589829750609));
#9128=CARTESIAN_POINT('Ctrl Pts',(20.9612451287423,-40.4196817819573,1.64906456309142));
#9129=CARTESIAN_POINT('Ctrl Pts',(21.2520030445599,-40.4992484506437,0.928922098091803));
#9130=CARTESIAN_POINT('Ctrl Pts',(21.5427609603775,-40.5788151193301,0.20877963309219));
#9131=CARTESIAN_POINT('Ctrl Pts',(21.5447386121598,-40.8251091511939,-0.532038515331461));
#9132=CARTESIAN_POINT('Ctrl Pts',(21.546716263942,-41.0714031830578,-1.27285666375511));
#9133=CARTESIAN_POINT('Ctrl Pts',(21.2807429103773,-41.4723987999884,-1.88762237576914));
#9134=CARTESIAN_POINT('Ctrl Pts',(21.0147695568125,-41.873394416919,-2.50238808778318));
#9135=CARTESIAN_POINT('Ctrl Pts',(20.5547454394013,-42.3864252945927,-2.86933947451654));
#9136=CARTESIAN_POINT('Ctrl Pts',(20.0947213219901,-42.8994561722665,-3.2362908612499));
#9137=CARTESIAN_POINT('Ctrl Pts',(19.5529808158895,-43.4596660289473,-3.28274870019663));
#9138=CARTESIAN_POINT('Ctrl Pts',(19.0112403097888,-44.0198758856281,-3.32920653914337));
#9139=CARTESIAN_POINT('Ctrl Pts',(18.5163027231212,-44.5530640641754,-3.04596928553206));
#9140=CARTESIAN_POINT('Ctrl Pts',(18.0213651364537,-45.0862522427227,-2.76273203192075));
#9141=CARTESIAN_POINT('Ctrl Pts',(17.6924798851479,-45.5235700607493,-2.20589829750609));
#9142=CARTESIAN_POINT('Ctrl Pts',(3.62216201968442,-19.8058202438613,-1.94799199564959));
#9143=CARTESIAN_POINT('Ctrl Pts',(3.34425572651223,-20.2137053466864,-1.54490813204841));
#9144=CARTESIAN_POINT('Ctrl Pts',(3.25594179788809,-20.5121292468035,-0.988830267143717));
#9145=CARTESIAN_POINT('Ctrl Pts',(3.16762786926396,-20.8105531469205,-0.432752402239027));
#9146=CARTESIAN_POINT('Ctrl Pts',(3.3076189187292,-20.9771651064803,0.166181422977342));
#9147=CARTESIAN_POINT('Ctrl Pts',(3.44760996819445,-21.1437770660401,0.765115248193711));
#9148=CARTESIAN_POINT('Ctrl Pts',(3.80940000840298,-21.1823333185883,1.28827884419634));
#9149=CARTESIAN_POINT('Ctrl Pts',(4.17119004861151,-21.2208895711365,1.81144244019896));
#9150=CARTESIAN_POINT('Ctrl Pts',(4.70434308191443,-21.1605093534924,2.15521684061908));
#9151=CARTESIAN_POINT('Ctrl Pts',(5.23749611521735,-21.1001291358485,2.49899124103919));
#9152=CARTESIAN_POINT('Ctrl Pts',(5.8576356015542,-20.9895272661294,2.59528770975726));
#9153=CARTESIAN_POINT('Ctrl Pts',(6.47777508789106,-20.8789253964104,2.69158417847533));
#9154=CARTESIAN_POINT('Ctrl Pts',(7.08329575335921,-20.7767637068552,2.52133001886304));
#9155=CARTESIAN_POINT('Ctrl Pts',(7.68881641882736,-20.6746020173,2.35107585925076));
#9156=CARTESIAN_POINT('Ctrl Pts',(8.18100842628526,-20.6378706589539,1.94799199564959));
#9157=CARTESIAN_POINT('Ctrl Pts',(8.67320043374317,-20.6011393006078,1.54490813204841));
#9158=CARTESIAN_POINT('Ctrl Pts',(8.97580007665302,-20.6738691449698,0.988830267143717));
#9159=CARTESIAN_POINT('Ctrl Pts',(9.27839971956287,-20.7465989893318,0.432752402239027));
#9160=CARTESIAN_POINT('Ctrl Pts',(9.35269438438334,-20.9511407742511,-0.166181422977342));
#9161=CARTESIAN_POINT('Ctrl Pts',(9.4269890492038,-21.1556825591703,-0.765115248193711));
#9162=CARTESIAN_POINT('Ctrl Pts',(9.27948472328098,-21.4882800511012,-1.28827884419634));
#9163=CARTESIAN_POINT('Ctrl Pts',(9.13198039735816,-21.8208775430321,-1.81144244019896));
#9164=CARTESIAN_POINT('Ctrl Pts',(8.81311307834095,-22.2524115051551,-2.15521684061908));
#9165=CARTESIAN_POINT('Ctrl Pts',(8.49424575932375,-22.6839454672782,-2.49899124103919));
#9166=CARTESIAN_POINT('Ctrl Pts',(8.0883919872726,-23.1657010814762,-2.59528770975726));
#9167=CARTESIAN_POINT('Ctrl Pts',(7.68253821522146,-23.6474566956743,-2.69158417847533));
#9168=CARTESIAN_POINT('Ctrl Pts',(7.29130326403902,-24.1207721297085,-2.52133001886305));
#9169=CARTESIAN_POINT('Ctrl Pts',(6.90006831285659,-24.5940875637428,-2.35107585925076));
#9170=CARTESIAN_POINT('Ctrl Pts',(6.62216201968439,-25.0019726665679,-1.94799199564959));
#9171=CARTESIAN_POINT('Ctrl Pts',(6.34425572651219,-25.4098577693931,-1.54490813204841));
#9172=CARTESIAN_POINT('Ctrl Pts',(6.25594179788806,-25.7082816695101,-0.988830267143717));
#9173=CARTESIAN_POINT('Ctrl Pts',(6.16762786926392,-26.0067055696272,-0.432752402239027));
#9174=CARTESIAN_POINT('Ctrl Pts',(6.30761891872917,-26.1733175291869,0.166181422977342));
#9175=CARTESIAN_POINT('Ctrl Pts',(6.44760996819441,-26.3399294887468,0.765115248193711));
#9176=CARTESIAN_POINT('Ctrl Pts',(6.80940000840295,-26.3784857412949,1.28827884419634));
#9177=CARTESIAN_POINT('Ctrl Pts',(7.17119004861148,-26.4170419938431,1.81144244019896));
#9178=CARTESIAN_POINT('Ctrl Pts',(7.7043430819144,-26.3566617761991,2.15521684061908));
#9179=CARTESIAN_POINT('Ctrl Pts',(8.23749611521731,-26.2962815585551,2.49899124103919));
#9180=CARTESIAN_POINT('Ctrl Pts',(8.85763560155417,-26.1856796888361,2.59528770975726));
#9181=CARTESIAN_POINT('Ctrl Pts',(9.47777508789103,-26.0750778191171,2.69158417847533));
#9182=CARTESIAN_POINT('Ctrl Pts',(10.0832957533592,-25.9729161295619,2.52133001886304));
#9183=CARTESIAN_POINT('Ctrl Pts',(10.6888164188273,-25.8707544400067,2.35107585925076));
#9184=CARTESIAN_POINT('Ctrl Pts',(11.1810084262852,-25.8340230816606,1.94799199564959));
#9185=CARTESIAN_POINT('Ctrl Pts',(11.6732004337431,-25.7972917233145,1.54490813204841));
#9186=CARTESIAN_POINT('Ctrl Pts',(11.975800076653,-25.8700215676765,0.988830267143717));
#9187=CARTESIAN_POINT('Ctrl Pts',(12.2783997195628,-25.9427514120385,0.432752402239027));
#9188=CARTESIAN_POINT('Ctrl Pts',(12.3526943843833,-26.1472931969577,-0.166181422977342));
#9189=CARTESIAN_POINT('Ctrl Pts',(12.4269890492038,-26.351834981877,-0.765115248193711));
#9190=CARTESIAN_POINT('Ctrl Pts',(12.279484723281,-26.6844324738078,-1.28827884419634));
#9191=CARTESIAN_POINT('Ctrl Pts',(12.1319803973581,-27.0170299657387,-1.81144244019896));
#9192=CARTESIAN_POINT('Ctrl Pts',(11.8131130783409,-27.4485639278618,-2.15521684061908));
#9193=CARTESIAN_POINT('Ctrl Pts',(11.4942457593237,-27.8800978899848,-2.49899124103919));
#9194=CARTESIAN_POINT('Ctrl Pts',(11.0883919872726,-28.3618535041829,-2.59528770975726));
#9195=CARTESIAN_POINT('Ctrl Pts',(10.6825382152214,-28.8436091183809,-2.69158417847533));
#9196=CARTESIAN_POINT('Ctrl Pts',(10.291303264039,-29.3169245524152,-2.52133001886305));
#9197=CARTESIAN_POINT('Ctrl Pts',(9.90006831285655,-29.7902399864494,-2.35107585925076));
#9198=CARTESIAN_POINT('Ctrl Pts',(9.62216201968436,-30.1981250892746,-1.94799199564959));
#9199=CARTESIAN_POINT('Ctrl Pts',(9.34425572651217,-30.6060101920997,-1.54490813204841));
#9200=CARTESIAN_POINT('Ctrl Pts',(9.25594179788803,-30.9044340922168,-0.988830267143717));
#9201=CARTESIAN_POINT('Ctrl Pts',(9.16762786926389,-31.2028579923338,-0.432752402239027));
#9202=CARTESIAN_POINT('Ctrl Pts',(9.30761891872914,-31.3694699518936,0.166181422977342));
#9203=CARTESIAN_POINT('Ctrl Pts',(9.44760996819438,-31.5360819114534,0.765115248193711));
#9204=CARTESIAN_POINT('Ctrl Pts',(9.80940000840292,-31.5746381640016,1.28827884419634));
#9205=CARTESIAN_POINT('Ctrl Pts',(10.1711900486115,-31.6131944165497,1.81144244019896));
#9206=CARTESIAN_POINT('Ctrl Pts',(10.7043430819144,-31.5528141989058,2.15521684061908));
#9207=CARTESIAN_POINT('Ctrl Pts',(11.2374961152173,-31.4924339812617,2.49899124103919));
#9208=CARTESIAN_POINT('Ctrl Pts',(11.8576356015541,-31.3818321115427,2.59528770975726));
#9209=CARTESIAN_POINT('Ctrl Pts',(12.477775087891,-31.2712302418237,2.69158417847533));
#9210=CARTESIAN_POINT('Ctrl Pts',(13.0832957533591,-31.1690685522685,2.52133001886304));
#9211=CARTESIAN_POINT('Ctrl Pts',(13.6888164188273,-31.0669068627133,2.35107585925076));
#9212=CARTESIAN_POINT('Ctrl Pts',(14.1810084262852,-31.0301755043672,1.94799199564959));
#9213=CARTESIAN_POINT('Ctrl Pts',(14.6732004337431,-30.9934441460211,1.54490813204841));
#9214=CARTESIAN_POINT('Ctrl Pts',(14.975800076653,-31.0661739903831,0.988830267143717));
#9215=CARTESIAN_POINT('Ctrl Pts',(15.2783997195628,-31.1389038347451,0.432752402239027));
#9216=CARTESIAN_POINT('Ctrl Pts',(15.3526943843833,-31.3434456196644,-0.166181422977342));
#9217=CARTESIAN_POINT('Ctrl Pts',(15.4269890492037,-31.5479874045836,-0.765115248193711));
#9218=CARTESIAN_POINT('Ctrl Pts',(15.2794847232809,-31.8805848965145,-1.28827884419634));
#9219=CARTESIAN_POINT('Ctrl Pts',(15.1319803973581,-32.2131823884454,-1.81144244019896));
#9220=CARTESIAN_POINT('Ctrl Pts',(14.8131130783409,-32.6447163505684,-2.15521684061908));
#9221=CARTESIAN_POINT('Ctrl Pts',(14.4942457593237,-33.0762503126915,-2.49899124103919));
#9222=CARTESIAN_POINT('Ctrl Pts',(14.0883919872725,-33.5580059268895,-2.59528770975726));
#9223=CARTESIAN_POINT('Ctrl Pts',(13.6825382152214,-34.0397615410876,-2.69158417847533));
#9224=CARTESIAN_POINT('Ctrl Pts',(13.291303264039,-34.5130769751218,-2.52133001886305));
#9225=CARTESIAN_POINT('Ctrl Pts',(12.9000683128565,-34.9863924091561,-2.35107585925076));
#9226=CARTESIAN_POINT('Ctrl Pts',(12.6221620196843,-35.3942775119812,-1.94799199564959));
#9227=CARTESIAN_POINT('Ctrl Pts',(12.3442557265121,-35.8021626148064,-1.54490813204841));
#9228=CARTESIAN_POINT('Ctrl Pts',(12.255941797888,-36.1005865149234,-0.988830267143717));
#9229=CARTESIAN_POINT('Ctrl Pts',(12.1676278692639,-36.3990104150405,-0.432752402239027));
#9230=CARTESIAN_POINT('Ctrl Pts',(12.3076189187291,-36.5656223746002,0.166181422977342));
#9231=CARTESIAN_POINT('Ctrl Pts',(12.4476099681944,-36.73223433416,0.765115248193711));
#9232=CARTESIAN_POINT('Ctrl Pts',(12.8094000084029,-36.7707905867082,1.28827884419634));
#9233=CARTESIAN_POINT('Ctrl Pts',(13.1711900486114,-36.8093468392564,1.81144244019896));
#9234=CARTESIAN_POINT('Ctrl Pts',(13.7043430819143,-36.7489666216124,2.15521684061908));
#9235=CARTESIAN_POINT('Ctrl Pts',(14.2374961152173,-36.6885864039684,2.49899124103919));
#9236=CARTESIAN_POINT('Ctrl Pts',(14.8576356015541,-36.5779845342494,2.59528770975726));
#9237=CARTESIAN_POINT('Ctrl Pts',(15.477775087891,-36.4673826645304,2.69158417847533));
#9238=CARTESIAN_POINT('Ctrl Pts',(16.0832957533591,-36.3652209749752,2.52133001886304));
#9239=CARTESIAN_POINT('Ctrl Pts',(16.6888164188273,-36.26305928542,2.35107585925076));
#9240=CARTESIAN_POINT('Ctrl Pts',(17.1810084262852,-36.2263279270739,1.94799199564959));
#9241=CARTESIAN_POINT('Ctrl Pts',(17.6732004337431,-36.1895965687278,1.54490813204841));
#9242=CARTESIAN_POINT('Ctrl Pts',(17.9758000766529,-36.2623264130898,0.988830267143717));
#9243=CARTESIAN_POINT('Ctrl Pts',(18.2783997195628,-36.3350562574518,0.432752402239027));
#9244=CARTESIAN_POINT('Ctrl Pts',(18.3526943843832,-36.539598042371,-0.166181422977342));
#9245=CARTESIAN_POINT('Ctrl Pts',(18.4269890492037,-36.7441398272903,-0.765115248193711));
#9246=CARTESIAN_POINT('Ctrl Pts',(18.2794847232809,-37.0767373192211,-1.28827884419634));
#9247=CARTESIAN_POINT('Ctrl Pts',(18.1319803973581,-37.409334811152,-1.81144244019896));
#9248=CARTESIAN_POINT('Ctrl Pts',(17.8131130783409,-37.8408687732751,-2.15521684061908));
#9249=CARTESIAN_POINT('Ctrl Pts',(17.4942457593237,-38.2724027353981,-2.49899124103919));
#9250=CARTESIAN_POINT('Ctrl Pts',(17.0883919872725,-38.7541583495962,-2.59528770975726));
#9251=CARTESIAN_POINT('Ctrl Pts',(16.6825382152214,-39.2359139637942,-2.69158417847533));
#9252=CARTESIAN_POINT('Ctrl Pts',(16.2913032640389,-39.7092293978285,-2.52133001886305));
#9253=CARTESIAN_POINT('Ctrl Pts',(15.9000683128565,-40.1825448318627,-2.35107585925076));
#9254=CARTESIAN_POINT('Ctrl Pts',(15.6221620196843,-40.5904299346879,-1.94799199564959));
#9255=CARTESIAN_POINT('Ctrl Pts',(15.3442557265121,-40.998315037513,-1.54490813204841));
#9256=CARTESIAN_POINT('Ctrl Pts',(15.255941797888,-41.2967389376301,-0.988830267143717));
#9257=CARTESIAN_POINT('Ctrl Pts',(15.1676278692638,-41.5951628377471,-0.432752402239027));
#9258=CARTESIAN_POINT('Ctrl Pts',(15.3076189187291,-41.7617747973069,0.166181422977342));
#9259=CARTESIAN_POINT('Ctrl Pts',(15.4476099681943,-41.9283867568667,0.765115248193711));
#9260=CARTESIAN_POINT('Ctrl Pts',(15.8094000084029,-41.9669430094149,1.28827884419634));
#9261=CARTESIAN_POINT('Ctrl Pts',(16.1711900486114,-42.0054992619631,1.81144244019896));
#9262=CARTESIAN_POINT('Ctrl Pts',(16.7043430819143,-41.945119044319,2.15521684061908));
#9263=CARTESIAN_POINT('Ctrl Pts',(17.2374961152172,-41.884738826675,2.49899124103919));
#9264=CARTESIAN_POINT('Ctrl Pts',(17.8576356015541,-41.774136956956,2.59528770975726));
#9265=CARTESIAN_POINT('Ctrl Pts',(18.4777750878909,-41.6635350872371,2.69158417847533));
#9266=CARTESIAN_POINT('Ctrl Pts',(19.0832957533591,-41.5613733976818,2.52133001886304));
#9267=CARTESIAN_POINT('Ctrl Pts',(19.6888164188272,-41.4592117081266,2.35107585925076));
#9268=CARTESIAN_POINT('Ctrl Pts',(20.1810084262851,-41.4224803497805,1.94799199564959));
#9269=CARTESIAN_POINT('Ctrl Pts',(20.673200433743,-41.3857489914344,1.54490813204841));
#9270=CARTESIAN_POINT('Ctrl Pts',(20.9758000766529,-41.4584788357964,0.988830267143717));
#9271=CARTESIAN_POINT('Ctrl Pts',(21.2783997195627,-41.5312086801584,0.432752402239027));
#9272=CARTESIAN_POINT('Ctrl Pts',(21.3526943843832,-41.7357504650777,-0.166181422977342));
#9273=CARTESIAN_POINT('Ctrl Pts',(21.4269890492037,-41.940292249997,-0.765115248193711));
#9274=CARTESIAN_POINT('Ctrl Pts',(21.2794847232809,-42.2728897419278,-1.28827884419634));
#9275=CARTESIAN_POINT('Ctrl Pts',(21.131980397358,-42.6054872338587,-1.81144244019896));
#9276=CARTESIAN_POINT('Ctrl Pts',(20.8131130783408,-43.0370211959817,-2.15521684061908));
#9277=CARTESIAN_POINT('Ctrl Pts',(20.4942457593236,-43.4685551581048,-2.49899124103919));
#9278=CARTESIAN_POINT('Ctrl Pts',(20.0883919872725,-43.9503107723028,-2.59528770975726));
#9279=CARTESIAN_POINT('Ctrl Pts',(19.6825382152213,-44.4320663865008,-2.69158417847533));
#9280=CARTESIAN_POINT('Ctrl Pts',(19.2913032640389,-44.9053818205351,-2.52133001886305));
#9281=CARTESIAN_POINT('Ctrl Pts',(18.9000683128565,-45.3786972545694,-2.35107585925076));
#9282=CARTESIAN_POINT('Ctrl Pts',(18.6221620196843,-45.7865823573945,-1.94799199564959));
#9549=UNCERTAINTY_MEASURE_WITH_UNIT(LENGTH_MEASURE(0.01),#9562,
'DISTANCE_ACCURACY_VALUE',
'Maximum model space distance between geometric entities at asserted c
onnectivities');
#9553=UNCERTAINTY_MEASURE_WITH_UNIT(LENGTH_MEASURE(0.01),#9562,
'DISTANCE_ACCURACY_VALUE',
'Maximum model space distance between geometric entities at asserted c
onnectivities');
#9557=(
GEOMETRIC_REPRESENTATION_CONTEXT(3)
GLOBAL_UNCERTAINTY_ASSIGNED_CONTEXT((#9549))
GLOBAL_UNIT_ASSIGNED_CONTEXT((#9562,#9564,#9565))
REPRESENTATION_CONTEXT('','3D')
);
#9561=(
GEOMETRIC_REPRESENTATION_CONTEXT(3)
GLOBAL_UNCERTAINTY_ASSIGNED_CONTEXT((#9553))
GLOBAL_UNIT_ASSIGNED_CONTEXT((#9562,#9564,#9565))
REPRESENTATION_CONTEXT('','3D')
);
#9562=(
LENGTH_UNIT()
NAMED_UNIT(*)
SI_UNIT(.MILLI.,.METRE.)
);
#9564=(
NAMED_UNIT(*)
PLANE_ANGLE_UNIT()
SI_UNIT($,.RADIAN.)
);
#9565=(
NAMED_UNIT(*)
SI_UNIT($,.STERADIAN.)
SOLID_ANGLE_UNIT()
);
#9569=SHAPE_DEFINITION_REPRESENTATION(#9576,#9589);
#9576=PRODUCT_DEFINITION_SHAPE('',$,#9597);
#9589=SHAPE_REPRESENTATION('',(#2590),#9557);
#9593=PRODUCT_DEFINITION_CONTEXT('part definition',#9616,'design');
#9597=PRODUCT_DEFINITION('Central Grooved Worm Spiral Wire',
'Central Grooved Worm Spiral Wire',#9604,#9593);
#9604=PRODUCT_DEFINITION_FORMATION('',$,#9621);
#9616=APPLICATION_CONTEXT(
'Core Data for Automotive Mechanical Design Process');
#9617=PRODUCT_CONTEXT('part definition',#9616,'mechanical');
#9621=PRODUCT('Central Grooved Worm Spiral Wire',
'Central Grooved Worm Spiral Wire',$,(#9617));
#9628=PRESENTATION_STYLE_ASSIGNMENT((#9633));
#9633=SURFACE_STYLE_USAGE(.BOTH.,#9638);
#9638=SURFACE_SIDE_STYLE('',(#9643));
#9643=SURFACE_STYLE_FILL_AREA(#9648);
#9648=FILL_AREA_STYLE('Opaque(227,224,212)',(#9653));
#9653=FILL_AREA_STYLE_COLOUR('Opaque(227,224,212)',#9658);
#9658=COLOUR_RGB('Opaque(227,224,212)',0.890196078431372,0.87843137254902,
0.831372549019608);
ENDSEC;
END-ISO-10303-21;
